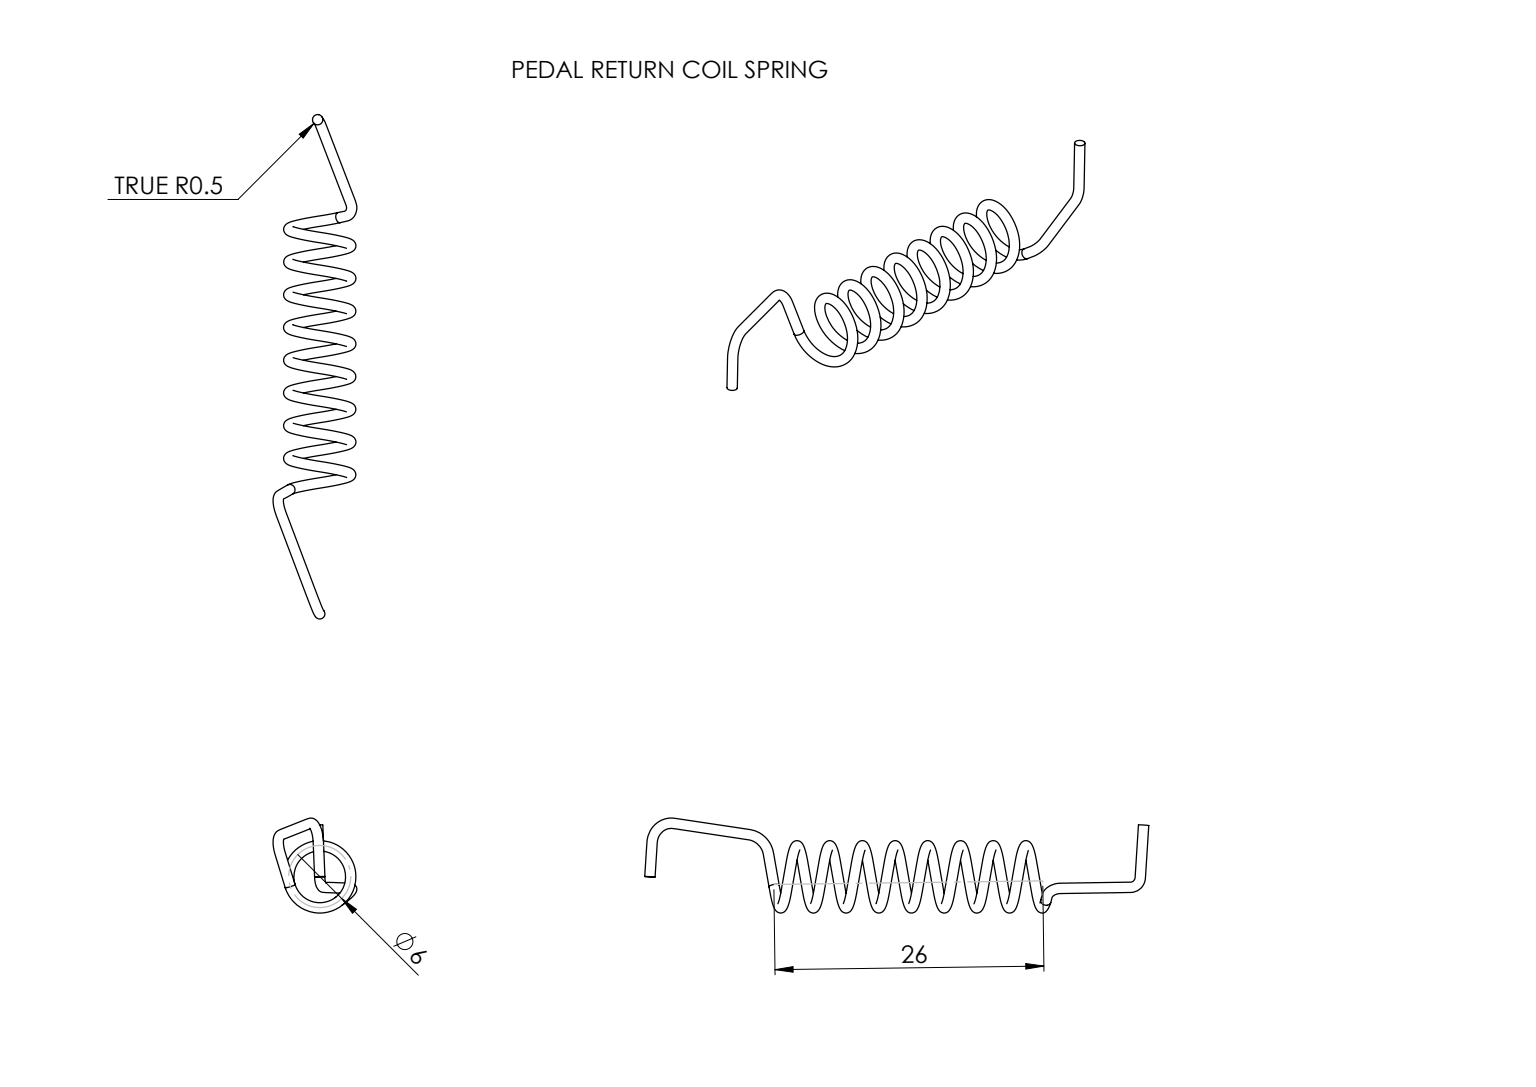
ISO-10303-21;
HEADER;
FILE_DESCRIPTION (('STEP AP214'),
    '1' );
FILE_NAME ('Pedal Return Coil Spring.step',
    '2026-09-30T16:28:02',
    ( '' ),
    ( '' ),
    'SwSTEP 2.0',
    'SolidWorks 2026',
    '' );
FILE_SCHEMA (( 'AUTOMOTIVE_DESIGN' ));
ENDSEC;

DATA;
#3=CARTESIAN_POINT ( 'NONE',  ( 10.46436961932593945, 16.48727764291732711, -17.33901581970886241 ) ) ;
#5=CARTESIAN_POINT ( 'NONE',  ( 33.35202879388211983, -12.33251541790028760, -19.68467382345759376 ) ) ;
#7=CARTESIAN_POINT ( 'NONE',  ( 11.86544027865023843, 7.919735734555668039, -16.84125344233394372 ) ) ;
#10=CARTESIAN_POINT ( 'NONE',  ( 20.51249478307574847, 1.942573248051725709, -13.31196225760961838 ) ) ;
#11=CARTESIAN_POINT ( 'NONE',  ( 11.27738072919014911, 16.67146171448561276, -16.78403338633166442 ) ) ;
#12=CARTESIAN_POINT ( 'NONE',  ( 35.03938282813840743, -19.89690018161999419, -20.20402626681843117 ) ) ;
#15=CARTESIAN_POINT ( 'NONE',  ( 9.776119957569173735, 17.05082265352876547, -16.72288386497739765 ) ) ;
#18=CARTESIAN_POINT ( 'NONE',  ( 9.641351338355821810, 17.66888872024471624, -17.91303689663363130 ) ) ;
#25=CARTESIAN_POINT ( 'NONE',  ( 10.43477690885096720, 16.62299358534909288, -17.37687480348504820 ) ) ;
#28=CARTESIAN_POINT ( 'NONE',  ( 36.54859390953724585, -22.18451583373416014, -17.64281456791166036 ) ) ;
#29=CARTESIAN_POINT ( 'NONE',  ( 24.62590367393082502, -9.567571807129121808, -15.85044010117769098 ) ) ;
#37=CARTESIAN_POINT ( 'NONE',  ( 19.85258860919307367, 6.732389232436280402, -16.96582824858274208 ) ) ;
#39=CARTESIAN_POINT ( 'NONE',  ( 29.40876261992080032, -8.787110225502646088, -16.42709622331022956 ) ) ;
#44=CARTESIAN_POINT ( 'NONE',  ( 10.00000000000007816, 17.32050807568872486, -23.00000000000000711 ) ) ;
#48=CARTESIAN_POINT ( 'NONE',  ( 10.33812866905494587, 18.38613571942487113, -17.90056368370468931 ) ) ;
#54=CARTESIAN_POINT ( 'NONE',  ( 9.917712295358372288, 16.40146214360271770, -16.50402730409559027 ) ) ;
#56=CARTESIAN_POINT ( 'NONE',  ( 28.55476651072185845, -11.97999099613336504, -13.94805024529803994 ) ) ;
#58=CARTESIAN_POINT ( 'NONE',  ( 25.71553203045151292, -8.406338935355361031, -18.42709291467145150 ) ) ;
#61=CARTESIAN_POINT ( 'NONE',  ( 11.05541548581436118, 17.68942261459453036, -17.91440211708152574 ) ) ;
#63=CARTESIAN_POINT ( 'NONE',  ( 32.97927115036063839, -11.75136040154610662, -17.31233706439427067 ) ) ;
#64=CARTESIAN_POINT ( 'NONE',  ( 14.34656430690936624, 9.113120221615268690, -15.03016663717492563 ) ) ;
#68=CARTESIAN_POINT ( 'NONE',  ( 23.37849240255853189, -5.075553540114302820, -18.86401745356084447 ) ) ;
#73=CARTESIAN_POINT ( 'NONE',  ( 16.00562779705659011, 2.776126820729137190, -17.20623408552720690 ) ) ;
#74=CARTESIAN_POINT ( 'NONE',  ( 16.42253358145367415, 4.166353156564198024, -16.06924993952044289 ) ) ;
#83=CARTESIAN_POINT ( 'NONE',  ( 9.641350810849047548, 17.66889113945805789, -17.91928203681695564 ) ) ;
#84=CARTESIAN_POINT ( 'NONE',  ( 20.82548126942529976, -5.669333895406754031, -14.77195412306030420 ) ) ;
#85=CARTESIAN_POINT ( 'NONE',  ( 23.74924978780510898, -3.048960050427876656, -13.27477993493952191 ) ) ;
#87=CARTESIAN_POINT ( 'NONE',  ( 36.54859390953724585, -23.18451583373416014, -18.06010107863414405 ) ) ;
#95=CARTESIAN_POINT ( 'NONE',  ( 10.33811987107833552, 18.38617606806709048, -17.90816805339326834 ) ) ;
#100=CARTESIAN_POINT ( 'NONE',  ( 14.18486973814142793, 6.324582201221724098, -17.68508340245422872 ) ) ;
#104=CARTESIAN_POINT ( 'NONE',  ( 25.08912532741139501, -12.86307741315042108, -14.91192194027685147 ) ) ;
#107=CARTESIAN_POINT ( 'NONE',  ( 34.90271572771163733, -20.28292729397994876, -21.20502438346732887 ) ) ;
#108=CARTESIAN_POINT ( 'NONE',  ( 24.18628427323349328, -0.8779346998738073449, -17.06787597161793357 ) ) ;
#109=CARTESIAN_POINT ( 'NONE',  ( 18.93384218461971358, 6.651393094135895190, -15.21227712214292538 ) ) ;
#111=CARTESIAN_POINT ( 'NONE',  ( 28.58746438791548528, -7.443717211345676432, -18.79719194573140584 ) ) ;
#120=CARTESIAN_POINT ( 'NONE',  ( 33.16581763841239194, -10.35476010881584052, -17.60936685258081624 ) ) ;
#121=CARTESIAN_POINT ( 'NONE',  ( 9.641890818133653340, 17.66641459721583374, -17.82828029666912073 ) ) ;
#126=CARTESIAN_POINT ( 'NONE',  ( 10.46960557229346733, 16.46326489517938541, -17.33590790293451178 ) ) ;
#139=CARTESIAN_POINT ( 'NONE',  ( 11.09431937732777129, 9.685491096586417825, -17.29518830297554643 ) ) ;
#140=CARTESIAN_POINT ( 'NONE',  ( 25.86320101420157158, -8.291784280105535032, -12.84902276017926859 ) ) ;
#141=CARTESIAN_POINT ( 'NONE',  ( 19.89307947303188229, -2.966738011908462092, -16.73278295482091949 ) ) ;
#143=CARTESIAN_POINT ( 'NONE',  ( 18.39996379557756256, 0.6904185378075045065, -15.43317298867526866 ) ) ;
#147=CARTESIAN_POINT ( 'NONE',  ( 27.44219139316946965, -6.774709612358828181, -18.29578255718776703 ) ) ;
#156=CARTESIAN_POINT ( 'NONE',  ( 10.35864918915110877, 16.97212501191939538, -17.92279151347709032 ) ) ;
#157=CARTESIAN_POINT ( 'NONE',  ( 35.24964364652129234, -20.84149066036063047, -20.16262864730545346 ) ) ;
#158=CARTESIAN_POINT ( 'NONE',  ( 31.39893620166130717, -10.86152586746012183, -14.84747879817187943 ) ) ;
#160=CARTESIAN_POINT ( 'NONE',  ( 8.944584812045984989, 16.95159217075808655, -17.91472939532503261 ) ) ;
#163=CARTESIAN_POINT ( 'NONE',  ( 19.38992137333195842, 2.881095379261479739, -20.30776781288435373 ) ) ;
#164=CARTESIAN_POINT ( 'NONE',  ( 11.27814055543051630, 16.66797705449195988, -16.78371917145281955 ) ) ;
#169=CARTESIAN_POINT ( 'NONE',  ( 9.916551108984865692, 16.40678749232849398, -16.50450761325770443 ) ) ;
#171=CARTESIAN_POINT ( 'NONE',  ( 9.843778300897430000, 16.74053286659246709, -16.57516421589427225 ) ) ;
#179=CARTESIAN_POINT ( 'NONE',  ( 10.35887147716723611, 16.97110557074245563, -17.87975733919941845 ) ) ;
#181=CARTESIAN_POINT ( 'NONE',  ( 36.04209255463945993, -19.90907354740926394, -20.43687144983462289 ) ) ;
#182=CARTESIAN_POINT ( 'NONE',  ( 21.18945582756405344, -5.194394521544061227, -16.21196392551894405 ) ) ;
#183=CARTESIAN_POINT ( 'NONE',  ( 27.21278356834291756, -7.014839303453253905, -18.45691071023835761 ) ) ;
#186=CIRCLE ( 'NONE', #15750, 0.4999999999999998335 ) ;
#189=CARTESIAN_POINT ( 'NONE',  ( 19.09420370221858931, 5.586061004495046056, -18.95245686415860220 ) ) ;
#190=CARTESIAN_POINT ( 'NONE',  ( 26.02011856185544048, -9.832954462109395166, -14.66174570188732140 ) ) ;
#200=CARTESIAN_POINT ( 'NONE',  ( 10.73095126193553028, 16.58460123524055874, -15.94999808000346242 ) ) ;
#204=CARTESIAN_POINT ( 'NONE',  ( 9.916551108984865692, 16.40678749232849398, -16.50450761325770443 ) ) ;
#206=CARTESIAN_POINT ( 'NONE',  ( 18.72855672543857608, 2.184447897796080174, -13.82944682127929426 ) ) ;
#210=CARTESIAN_POINT ( 'NONE',  ( 25.79824969357368047, -12.24460132778619226, -15.92960863319586906 ) ) ;
#213=CARTESIAN_POINT ( 'NONE',  ( 11.05541700792677062, 17.68941563399299710, -17.91138715956864047 ) ) ;
#215=CARTESIAN_POINT ( 'NONE',  ( 33.76744293605320024, -13.18274801178271005, -18.77722780292321758 ) ) ;
#219=CARTESIAN_POINT ( 'NONE',  ( 23.38597214775318278, -9.778565425610747042, -17.35394146810280347 ) ) ;
#223=CARTESIAN_POINT ( 'NONE',  ( 21.13650371987585075, 4.769999862021419901, -15.38713752973847448 ) ) ;
#224=CARTESIAN_POINT ( 'NONE',  ( 17.80416238081608071, 8.561068417093343541, -18.87148919878627140 ) ) ;
#238=CARTESIAN_POINT ( 'NONE',  ( 9.921764701973689426, 16.38287729030320250, -16.50235149140834778 ) ) ;
#239=CARTESIAN_POINT ( 'NONE',  ( 23.58034929565730309, -2.629172400889816075, -20.70693660786654888 ) ) ;
#240=CARTESIAN_POINT ( 'NONE',  ( 19.50876870223950377, -1.661710298099399630, -15.95382585723518432 ) ) ;
#241=CARTESIAN_POINT ( 'NONE',  ( 32.24963562184495203, -10.43994945000269148, -19.19593526939238970 ) ) ;
#242=ORIENTED_EDGE ( 'NONE', *, *, #15818, .F. ) ;
#248=CARTESIAN_POINT ( 'NONE',  ( 14.39533340154967433, 6.572929804808670617, -18.54476805420031837 ) ) ;
#251=CARTESIAN_POINT ( 'NONE',  ( 10.68867725192709273, 16.77847523382220984, -15.97313786900300059 ) ) ;
#255=CARTESIAN_POINT ( 'NONE',  ( 19.20291185354690811, 8.143073066566493878, -16.32372945079811188 ) ) ;
#256=CARTESIAN_POINT ( 'NONE',  ( 16.48605814428184857, 11.34583003460130435, -14.75612992736757256 ) ) ;
#258=CARTESIAN_POINT ( 'NONE',  ( 35.54859390953724585, -23.18451583373416014, -16.11276402859391510 ) ) ;
#259=CARTESIAN_POINT ( 'NONE',  ( 20.30498772102510685, -2.023023832184298154, -16.94527736422809028 ) ) ;
#260=CARTESIAN_POINT ( 'NONE',  ( 18.10666546173949953, 1.615696121519054618, -15.79491705146812563 ) ) ;
#262=CARTESIAN_POINT ( 'NONE',  ( 25.27233071153842303, -10.58027458246514207, -17.53878701932553952 ) ) ;
#272=CARTESIAN_POINT ( 'NONE',  ( 36.32827445255054499, -20.19473721995742821, -19.46526261299151983 ) ) ;
#273=CARTESIAN_POINT ( 'NONE',  ( 15.87304960759194650, 9.003283391651189405, -12.44179493704351280 ) ) ;
#277=CARTESIAN_POINT ( 'NONE',  ( 10.55304143273637330, 16.08061740358965253, -17.30129946959702281 ) ) ;
#289=CARTESIAN_POINT ( 'NONE',  ( 9.667856465286563505, 16.22743184293591057, -17.88508098240584587 ) ) ;
#290=CARTESIAN_POINT ( 'NONE',  ( 26.82298874931487020, -4.830090842487210878, -14.67398021261910301 ) ) ;
#291=CARTESIAN_POINT ( 'NONE',  ( 23.41849298471255381, -3.203224238779429633, -13.27670244232306018 ) ) ;
#296=CARTESIAN_POINT ( 'NONE',  ( 25.26806593431409453, -8.821542497490490575, -18.05414547114721557 ) ) ;
#309=CARTESIAN_POINT ( 'NONE',  ( 10.47103768343372288, 16.45669705093847313, -17.33522727542475295 ) ) ;
#313=CARTESIAN_POINT ( 'NONE',  ( 13.40647825129878612, 7.637826363492710158, -15.68645975549014082 ) ) ;
#316=CARTESIAN_POINT ( 'NONE',  ( 23.66272512268759343, 2.894330346666426745, -16.12005855839824520 ) ) ;
#317=CARTESIAN_POINT ( 'NONE',  ( 11.27662090294977837, 16.67494637447927275, -16.78434760121053060 ) ) ;
#321=CARTESIAN_POINT ( 'NONE',  ( 9.641350835837977584, 17.66889102485563612, -17.91507476468484938 ) ) ;
#324=CARTESIAN_POINT ( 'NONE',  ( 9.916953853453376766, 16.40494045485788632, -16.50434094533541085 ) ) ;
#330=CARTESIAN_POINT ( 'NONE',  ( 10.47325967749744180, 16.44650670292386607, -17.33429203187744250 ) ) ;
#333=CARTESIAN_POINT ( 'NONE',  ( 32.72409873491027099, -9.637868425582460929, -18.36260606011342844 ) ) ;
#334=CARTESIAN_POINT ( 'NONE',  ( 29.22485947447185595, -8.910266539455653501, -18.36689805200119707 ) ) ;
#335=CARTESIAN_POINT ( 'NONE',  ( 25.23810427664335165, -6.496417100615061280, -13.69959235629456629 ) ) ;
#338=CARTESIAN_POINT ( 'NONE',  ( 34.33515578781254618, -12.24072284059296933, -19.92088757525016973 ) ) ;
#340=CARTESIAN_POINT ( 'NONE',  ( 15.71409287621466788, 5.292507472020409942, -15.15310296786427635 ) ) ;
#341=CARTESIAN_POINT ( 'NONE',  ( 26.65048721414892086, -11.67344998524500355, -15.88597958324129777 ) ) ;
#353=CARTESIAN_POINT ( 'NONE',  ( 10.71275814632708823, 16.66803718250374899, -15.95787532639072914 ) ) ;
#358=CARTESIAN_POINT ( 'NONE',  ( 9.914377700407460026, 16.41675502110963336, -16.50544604630902867 ) ) ;
#359=CARTESIAN_POINT ( 'NONE',  ( 9.667469407758799704, 16.22920693809672343, -17.88529630510330293 ) ) ;
#360=CARTESIAN_POINT ( 'NONE',  ( 17.70496941102466693, 2.403166580496164606, -19.15355645582771871 ) ) ;
#363=CARTESIAN_POINT ( 'NONE',  ( 29.90031526554274777, -7.862644070287768905, -16.42500436498598049 ) ) ;
#365=CARTESIAN_POINT ( 'NONE',  ( 11.27712745377669101, 16.67262326781682802, -16.78413812462462573 ) ) ;
#367=CARTESIAN_POINT ( 'NONE',  ( 35.54859390953724585, -21.18451583373416014, -16.94733705004010105 ) ) ;
#370=CARTESIAN_POINT ( 'NONE',  ( 9.112490548836888138, 16.18155505883174783, -17.05474119751274031 ) ) ;
#371=CARTESIAN_POINT ( 'NONE',  ( 28.50845745928996067, -4.315366227951761502, -16.60164569054668604 ) ) ;
#375=CARTESIAN_POINT ( 'NONE',  ( 18.32179412900206827, 3.681508181950223335, -14.15692665485406643 ) ) ;
#377=CARTESIAN_POINT ( 'NONE',  ( 16.45434084995319424, 8.990804261541395448, -14.78801614696073408 ) ) ;
#387=CARTESIAN_POINT ( 'NONE',  ( 9.926830210242822972, 16.35964622367879784, -16.50025672554925293 ) ) ;
#388=CARTESIAN_POINT ( 'NONE',  ( 29.32553208039167458, -8.962988822949116141, -16.84503999589972523 ) ) ;
#389=CARTESIAN_POINT ( 'NONE',  ( 19.55718041265476970, -1.390565517676688900, -17.79492730709450754 ) ) ;
#390=CARTESIAN_POINT ( 'NONE',  ( 36.54859390953724585, -23.18451583373416014, -16.94733705004010105 ) ) ;
#396=CARTESIAN_POINT ( 'NONE',  ( 14.03850921439652311, 8.975161913830900673, -15.18271992443145635 ) ) ;
#399=CARTESIAN_POINT ( 'NONE',  ( 10.35722669462089840, 18.29854973974792998, -17.31575102165233915 ) ) ;
#403=CARTESIAN_POINT ( 'NONE',  ( 15.14574614762244487, 6.587483969391940697, -15.14885142785537830 ) ) ;
#405=CARTESIAN_POINT ( 'NONE',  ( 12.96291568738609890, 5.695260009123724210, -16.43886026595064109 ) ) ;
#407=CARTESIAN_POINT ( 'NONE',  ( 32.30218501430429967, -10.99871056796995816, -17.40035725849610060 ) ) ;
#410=CARTESIAN_POINT ( 'NONE',  ( 23.12480016457037379, 1.528454477237789488, -15.53356264363713102 ) ) ;
#412=CARTESIAN_POINT ( 'NONE',  ( 19.55510877418759819, -0.09764134006120470111, -19.21341144728512518 ) ) ;
#414=CARTESIAN_POINT ( 'NONE',  ( 27.32534031592636836, -8.675155620653059785, -19.25315075663615971 ) ) ;
#422=CARTESIAN_POINT ( 'NONE',  ( 35.57309713841538468, -16.80212557611773505, -19.25277297559858525 ) ) ;
#423=CARTESIAN_POINT ( 'NONE',  ( 9.641566850259106758, 17.66790035518494051, -17.86107206016944460 ) ) ;
#427=CARTESIAN_POINT ( 'NONE',  ( 12.02823749386838514, 9.315180647891255106, -16.69125397286443047 ) ) ;
#437=CARTESIAN_POINT ( 'NONE',  ( 9.667845848563926481, 16.22748053257927126, -17.88508528815513543 ) ) ;
#441=CARTESIAN_POINT ( 'NONE',  ( 25.04433344647707571, -4.420048373160954114, -18.22226412361657921 ) ) ;
#443=CARTESIAN_POINT ( 'NONE',  ( 21.55249387529322647, -4.041031698679099726, -14.19001464829599435 ) ) ;
#447=DIRECTION ( 'NONE',  ( -0.7172983783020613346, 0.6967661275386690667, -3.330669073875468142E-16 ) ) ;
#448=CARTESIAN_POINT ( 'NONE',  ( 26.72181814967143509, -3.137724904577397389, -15.69709663067708050 ) ) ;
#456=CARTESIAN_POINT ( 'NONE',  ( 12.02305193244137449, 9.338961869187645704, -16.69339841729684437 ) ) ;
#458=CARTESIAN_POINT ( 'NONE',  ( 34.96805304670973413, -19.57645325810014114, -20.18246498508359466 ) ) ;
#460=CARTESIAN_POINT ( 'NONE',  ( 13.81482270056995532, 7.818281081198240834, -15.36100202165747675 ) ) ;
#463=CARTESIAN_POINT ( 'NONE',  ( 21.66440995182641416, 5.535554982823286174, -17.57621636221614025 ) ) ;
#464=CARTESIAN_POINT ( 'NONE',  ( 12.84801357566967717, 9.517348710814296453, -16.13078356789775469 ) ) ;
#469=CARTESIAN_POINT ( 'NONE',  ( 11.40798482813988635, 9.566882342703072695, -15.88774718835883348 ) ) ;
#471=CARTESIAN_POINT ( 'NONE',  ( 10.24089172292967298, 14.91932009296530559, -16.37038124228770997 ) ) ;
#476=CARTESIAN_POINT ( 'NONE',  ( 10.40163623209820365, 16.77498095339038287, -17.46874319472340176 ) ) ;
#479=CARTESIAN_POINT ( 'NONE',  ( 32.45862320860160821, -9.597537451891041016, -17.61229109800368064 ) ) ;
#480=CARTESIAN_POINT ( 'NONE',  ( 29.62588713853392264, -10.65184931322849060, -12.76488833982454629 ) ) ;
#481=CARTESIAN_POINT ( 'NONE',  ( 29.46565128511723586, -7.689737916804423534, -14.82739468409561567 ) ) ;
#492=CARTESIAN_POINT ( 'NONE',  ( 28.92040988821396752, -12.03996551347764132, -12.87516188627701474 ) ) ;
#493=CARTESIAN_POINT ( 'NONE',  ( 26.45169718342334164, -9.008644514675534509, -18.11399877363951205 ) ) ;
#503=CARTESIAN_POINT ( 'NONE',  ( 10.33813570737955700, 18.38610344077106973, -17.89676158639688452 ) ) ;
#507=CARTESIAN_POINT ( 'NONE',  ( 9.917965570771830386, 16.40030059027150600, -16.50392256580263606 ) ) ;
#508=CARTESIAN_POINT ( 'NONE',  ( 20.43163981785493988, 0.2187255735321424754, -20.49791845872360341 ) ) ;
#514=CARTESIAN_POINT ( 'NONE',  ( 11.27864710625743427, 16.66565394782951515, -16.78350969486689692 ) ) ;
#516=EDGE_LOOP ( 'NONE', ( #242, #27504, #8040, #18443, #3018 ) ) ;
#517=CARTESIAN_POINT ( 'NONE',  ( 35.24753590068310416, -19.83202167481471889, -19.22462439892593977 ) ) ;
#519=CARTESIAN_POINT ( 'NONE',  ( 17.72480397827495224, 1.356124466512965476, -19.40231245121514903 ) ) ;
#522=CARTESIAN_POINT ( 'NONE',  ( 9.112135424753279977, 16.18318370314694832, -17.05489040841110437 ) ) ;
#523=CARTESIAN_POINT ( 'NONE',  ( 24.27832910178602788, -5.559203070376852018, -13.12236226054620047 ) ) ;
#530=CARTESIAN_POINT ( 'NONE',  ( 21.58357356133149807, 4.347441036859617469, -17.91576365920758107 ) ) ;
#531=CARTESIAN_POINT ( 'NONE',  ( 18.42634509371275797, 7.189141296957872740, -15.94500943014882210 ) ) ;
#545=CARTESIAN_POINT ( 'NONE',  ( 9.916411867603999397, 16.40742607105030260, -16.50456570466356965 ) ) ;
#546=CARTESIAN_POINT ( 'NONE',  ( 28.54819463643023880, -8.737303380947411213, -14.37855314081258307 ) ) ;
#547=CARTESIAN_POINT ( 'NONE',  ( 20.97044927184332508, -4.289323992320570156, -15.06659861376252429 ) ) ;
#549=CARTESIAN_POINT ( 'NONE',  ( 32.45272648307624053, -11.02157468472264412, -17.82583700188536824 ) ) ;
#555=CARTESIAN_POINT ( 'NONE',  ( 16.09764958744793262, 8.143416238145906760, -19.84970969296679044 ) ) ;
#558=CARTESIAN_POINT ( 'NONE',  ( 10.33819201225523621, 18.38584521943398187, -17.87775236254758227 ) ) ;
#561=CARTESIAN_POINT ( 'NONE',  ( 17.32695330507268494, 5.471673316493076200, -20.08600194542987794 ) ) ;
#562=CARTESIAN_POINT ( 'NONE',  ( 16.38450301900381945, 9.168174629645104545, -21.04437084800770918 ) ) ;
#564=CARTESIAN_POINT ( 'NONE',  ( 32.45272648307624053, -11.02157468472264412, -17.82583700188536824 ) ) ;
#566=CARTESIAN_POINT ( 'NONE',  ( 23.60892706051935619, -2.861763136178346212, -14.25286661070829908 ) ) ;
#568=CARTESIAN_POINT ( 'NONE',  ( 22.48601049859325585, 2.925819830077934558, -17.76611561182923893 ) ) ;
#569=CARTESIAN_POINT ( 'NONE',  ( 28.63790973356518776, -5.888324979419876648, -13.82040474618100312 ) ) ;
#577=CARTESIAN_POINT ( 'NONE',  ( 32.71419323209526908, -10.28616775856061416, -16.33292762241428520 ) ) ;
#579=CARTESIAN_POINT ( 'NONE',  ( 9.641354186875979337, 17.66887565656821124, -17.90893343548146177 ) ) ;
#583=CARTESIAN_POINT ( 'NONE',  ( 13.10707286029108865, 8.563798077496334926, -15.92507172258792281 ) ) ;
#593=CARTESIAN_POINT ( 'NONE',  ( 11.22273001195053155, 9.096583557657577757, -17.24208598844832352 ) ) ;
#594=CARTESIAN_POINT ( 'NONE',  ( 27.63487812444411418, -5.020849242181972372, -17.14317672846274831 ) ) ;
#595=CARTESIAN_POINT ( 'NONE',  ( 26.02348467347448491, -3.622150272347476108, -19.21400332953221124 ) ) ;
#602=CARTESIAN_POINT ( 'NONE',  ( 35.54859390953723874, -22.18451583373416014, -15.00000000000000000 ) ) ;
#605=CARTESIAN_POINT ( 'NONE',  ( 12.02786405831828986, 9.316892843345049968, -16.69140843421181231 ) ) ;
#609=CARTESIAN_POINT ( 'NONE',  ( 32.54305136433941215, -11.03529315477374517, -18.08112484791816499 ) ) ;
#611=CARTESIAN_POINT ( 'NONE',  ( 8.944584663113916534, 16.95159285377954461, -17.91618150236991269 ) ) ;
#616=CARTESIAN_POINT ( 'NONE',  ( 23.86551563699305234, 2.542095107771292106, -17.79649620197707094 ) ) ;
#617=CARTESIAN_POINT ( 'NONE',  ( 12.83210864641033844, 9.541281304504437344, -16.14109870176968897 ) ) ;
#620=CARTESIAN_POINT ( 'NONE',  ( 11.47029057985033340, 9.281140223223081520, -15.86198156829250117 ) ) ;
#622=CARTESIAN_POINT ( 'NONE',  ( 9.745779815811758340, 17.18996641109745482, -16.82979807527155458 ) ) ;
#627=CARTESIAN_POINT ( 'NONE',  ( 12.00785540763395254, 9.408655069060824161, -16.69968271487400813 ) ) ;
#629=CARTESIAN_POINT ( 'NONE',  ( 36.54859390954303677, -22.18451583373416014, -15.55638201429745848 ) ) ;
#630=CARTESIAN_POINT ( 'NONE',  ( 30.24922550192677306, -10.40856591028444278, -13.02298783260255988 ) ) ;
#631=CARTESIAN_POINT ( 'NONE',  ( 27.11191462667604313, -11.78482644060662743, -13.28705938033944989 ) ) ;
#636=CARTESIAN_POINT ( 'NONE',  ( 17.00902653454025071, 3.367308883600929281, -16.20218648120260951 ) ) ;
#637=CARTESIAN_POINT ( 'NONE',  ( 26.84622329165386745, -11.42663724297536554, -16.80226328336580366 ) ) ;
#649=CARTESIAN_POINT ( 'NONE',  ( 12.26681336913932974, 9.540941834721429871, -15.31486507153535648 ) ) ;
#654=CARTESIAN_POINT ( 'NONE',  ( 12.23783994716398560, 8.515526397163364791, -15.33449341356891615 ) ) ;
#656=CARTESIAN_POINT ( 'NONE',  ( 17.93652952100233833, 4.843921488302829204, -14.86957952233187896 ) ) ;
#661=CARTESIAN_POINT ( 'NONE',  ( 12.83625023806442655, 9.529724225483313660, -16.13881881377442795 ) ) ;
#663=CARTESIAN_POINT ( 'NONE',  ( 33.57416420788476330, -12.34692739235205217, -18.69991813917680190 ) ) ;
#664=CARTESIAN_POINT ( 'NONE',  ( 14.33367420948735393, 6.252843122977492563, -16.41390433006782956 ) ) ;
#666=CARTESIAN_POINT ( 'NONE',  ( 22.02790516022008660, -6.446180030103099590, -16.19395709203531197 ) ) ;
#670=CARTESIAN_POINT ( 'NONE',  ( 21.81760893248375766, -3.923850722439390815, -13.93537712798182682 ) ) ;
#671=CARTESIAN_POINT ( 'NONE',  ( 15.53255613197921647, 5.987779765840379298, -16.04456276566740058 ) ) ;
#684=CARTESIAN_POINT ( 'NONE',  ( 11.47748818427356987, 9.248962635895034978, -15.85894168489154765 ) ) ;
#686=CARTESIAN_POINT ( 'NONE',  ( 29.25528888857379783, -9.059906918047152757, -17.02304095575280130 ) ) ;
#687=CARTESIAN_POINT ( 'NONE',  ( 21.37428249720081297, 2.009508332918806151, -14.44682725892062614 ) ) ;
#688=CARTESIAN_POINT ( 'NONE',  ( 35.54750751241274287, -23.17963522693337453, -18.53372063443203999 ) ) ;
#695=CARTESIAN_POINT ( 'NONE',  ( 20.52488529563827058, 3.974637744936419637, -19.97762432673833288 ) ) ;
#698=CARTESIAN_POINT ( 'NONE',  ( 10.72031594518761466, 16.63337615353409760, -15.95439753950889106 ) ) ;
#702=CARTESIAN_POINT ( 'NONE',  ( 22.29983652437130814, 0.6627547066652448304, -20.09853802436992964 ) ) ;
#704=CARTESIAN_POINT ( 'NONE',  ( 28.86700826148938859, -9.048814421258168039, -19.66053155205330683 ) ) ;
#706=CARTESIAN_POINT ( 'NONE',  ( 35.32886446602115171, -21.19738783794349857, -20.03221113960638178 ) ) ;
#707=CARTESIAN_POINT ( 'NONE',  ( 22.40033610297568956, 1.362009800809227178, -14.54093962742820700 ) ) ;
#708=CARTESIAN_POINT ( 'NONE',  ( 19.97593658988278165, 3.663230212540239616, -18.70116431613266883 ) ) ;
#715=CARTESIAN_POINT ( 'NONE',  ( 34.70514358766799745, -13.90287004036446739, -20.03273298744158737 ) ) ;
#716=CARTESIAN_POINT ( 'NONE',  ( 12.81042928357508970, 7.649856678006609734, -14.88275739421262855 ) ) ;
#719=CARTESIAN_POINT ( 'NONE',  ( 13.12048998592846871, 8.569482736746577345, -15.91439669260688561 ) ) ;
#728=CARTESIAN_POINT ( 'NONE',  ( 11.21893088074867073, 9.114006857625895464, -17.24365706284262600 ) ) ;
#729=CARTESIAN_POINT ( 'NONE',  ( 24.63339645208565543, -5.721020077635508905, -14.05062826560360278 ) ) ;
#730=CARTESIAN_POINT ( 'NONE',  ( 20.05514754915220266, -1.452567280579552866, -14.87399747198034738 ) ) ;
#743=CARTESIAN_POINT ( 'NONE',  ( 10.79618582965528439, 14.96552620561766567, -17.20075070836251996 ) ) ;
#745=CARTESIAN_POINT ( 'NONE',  ( 33.55945865873172096, -12.30028340163019607, -18.68418013052470883 ) ) ;
#747=CARTESIAN_POINT ( 'NONE',  ( 13.39286676965551059, 7.631811206235384226, -15.69730834661896424 ) ) ;
#750=CARTESIAN_POINT ( 'NONE',  ( 21.69765170278760280, -5.035756590920279940, -14.89200278627170881 ) ) ;
#751=CARTESIAN_POINT ( 'NONE',  ( 12.86751881037522871, 9.515731068868671372, -16.11601834121851340 ) ) ;
#757=CARTESIAN_POINT ( 'NONE',  ( 11.47155695691762212, 9.275332456566969697, -15.86145787682774078 ) ) ;
#759=CARTESIAN_POINT ( 'NONE',  ( 9.870716668364401869, 16.61699007954640805, -16.53972800451630931 ) ) ;
#765=CARTESIAN_POINT ( 'NONE',  ( 12.02932678857878734, 9.310239991255825132, -16.69079931733866218 ) ) ;
#768=CARTESIAN_POINT ( 'NONE',  ( 36.54859682288668665, -23.18452892187019643, -18.24988411864624993 ) ) ;
#769=CARTESIAN_POINT ( 'NONE',  ( 24.62590367393082502, -9.567571807129121808, -15.85044010117769098 ) ) ;
#770=CARTESIAN_POINT ( 'NONE',  ( 31.22280883588763700, -10.09333740185288875, -13.86128061636125786 ) ) ;
#773=CARTESIAN_POINT ( 'NONE',  ( 34.31936231504242585, -12.17391896401218609, -19.91370162440023250 ) ) ;
#777=CARTESIAN_POINT ( 'NONE',  ( 18.73405575602592776, 1.888441813480535414, -14.99786396448725156 ) ) ;
#780=CARTESIAN_POINT ( 'NONE',  ( 14.79111372287554715, 6.954724682967856175, -19.27298399620107361 ) ) ;
#792=CARTESIAN_POINT ( 'NONE',  ( 12.27691635572497830, 9.494607244959519576, -15.31068720787289728 ) ) ;
#798=CARTESIAN_POINT ( 'NONE',  ( 12.50226005284522657, 8.571700941790735939, -15.12837371066060221 ) ) ;
#801=CARTESIAN_POINT ( 'NONE',  ( 19.55603740332541918, 4.113176889600292263, -19.54140316641015573 ) ) ;
#807=CARTESIAN_POINT ( 'NONE',  ( 12.57288446902313872, 10.73011642529405307, -16.24829701787703939 ) ) ;
#809=CARTESIAN_POINT ( 'NONE',  ( 34.19542162461613799, -15.10542955289956346, -18.90659549333309286 ) ) ;
#810=CARTESIAN_POINT ( 'NONE',  ( 15.14574614762244487, 6.587483969391940697, -15.14885142785537830 ) ) ;
#812=CARTESIAN_POINT ( 'NONE',  ( 16.96387855261641775, 8.441957738943033362, -20.67322241009641814 ) ) ;
#816=CARTESIAN_POINT ( 'NONE',  ( 21.34960977245966873, -3.524359730468174412, -18.69795900347392248 ) ) ;
#818=CARTESIAN_POINT ( 'NONE',  ( 17.70496941102466693, 2.403166580496164606, -19.15355645582771871 ) ) ;
#828=DIRECTION ( 'NONE',  ( 1.665334536937734318E-16, -2.498001805406601723E-16, -1.000000000000000000 ) ) ;
#833=CARTESIAN_POINT ( 'NONE',  ( 11.55687758731922798, 9.016417257711555777, -15.81607864292198329 ) ) ;
#834=CARTESIAN_POINT ( 'NONE',  ( 26.64397501440380012, -9.555891369342745634, -14.23407566704858951 ) ) ;
#835=CARTESIAN_POINT ( 'NONE',  ( 24.30592326428028827, -5.273034306582022879, -19.67074064463221106 ) ) ;
#836=CARTESIAN_POINT ( 'NONE',  ( 33.41663030065195272, -12.60673267154789201, -19.71350710734569134 ) ) ;
#845=CARTESIAN_POINT ( 'NONE',  ( 18.21616227284554057, 4.699354889203569918, -13.86658597208997179 ) ) ;
#848=CARTESIAN_POINT ( 'NONE',  ( 12.27693042220145969, 9.494543488390625896, -15.31068133337694803 ) ) ;
#853=CARTESIAN_POINT ( 'NONE',  ( 18.34549112274340033, 0.9605221043122941227, -13.99314825615798341 ) ) ;
#854=CARTESIAN_POINT ( 'NONE',  ( 18.76228799092704236, 0.4007544294800896578, -19.29634928253052806 ) ) ;
#856=CARTESIAN_POINT ( 'NONE',  ( 33.54145741815126058, -13.16751478770765793, -19.75123935038191192 ) ) ;
#857=( NAMED_UNIT ( * ) PLANE_ANGLE_UNIT ( ) SI_UNIT ( $, .RADIAN. ) );
#858=CARTESIAN_POINT ( 'NONE',  ( 25.72734949418555317, -2.696321649843969936, -17.76569039084671786 ) ) ;
#859=CARTESIAN_POINT ( 'NONE',  ( 17.76107737582129431, 3.703408080355245158, -15.36634439411934316 ) ) ;
#874=CARTESIAN_POINT ( 'NONE',  ( 33.36027191889437660, -10.38700102556154903, -18.15738432823107473 ) ) ;
#875=CIRCLE ( 'NONE', #26731, 0.4999999999999998335 ) ;
#876=CARTESIAN_POINT ( 'NONE',  ( 9.905109554012803130, 16.45925992188944420, -16.51025697316969953 ) ) ;
#879=CARTESIAN_POINT ( 'NONE',  ( 12.02558468657594659, 9.327346335875439820, -16.69235103436730938 ) ) ;
#889=CARTESIAN_POINT ( 'NONE',  ( 13.34629304935920757, 7.611730149031187054, -15.73439023580873730 ) ) ;
#891=CARTESIAN_POINT ( 'NONE',  ( 14.42366234001531922, 7.375548675892134476, -20.85295579936483179 ) ) ;
#893=CARTESIAN_POINT ( 'NONE',  ( 19.95076809599375878, -1.008983920988137495, -18.52968236344498720 ) ) ;
#904=CARTESIAN_POINT ( 'NONE',  ( 11.70392491148546732, 10.80251906652491556, -16.82536866641744311 ) ) ;
#905=CARTESIAN_POINT ( 'NONE',  ( 35.32886446602115171, -21.19738783794349857, -20.03221113960638178 ) ) ;
#908=CARTESIAN_POINT ( 'NONE',  ( 9.274674406624409784, 15.43775921338471413, -16.98767239532306661 ) ) ;
#909=CARTESIAN_POINT ( 'NONE',  ( 21.18945582756405344, -5.194394521544061227, -16.21196392551894405 ) ) ;
#910=CARTESIAN_POINT ( 'NONE',  ( 12.86796368952119174, 9.515911916162036022, -16.11566496612908139 ) ) ;
#917=CARTESIAN_POINT ( 'NONE',  ( 11.45661370752365116, 9.343864103108954211, -15.86763743611193789 ) ) ;
#923=CARTESIAN_POINT ( 'NONE',  ( 12.67163634847678644, 8.538173360731750705, -16.25940050138558135 ) ) ;
#925=CARTESIAN_POINT ( 'NONE',  ( 36.54859390953723874, -23.18451583373416014, -14.99999999999999822 ) ) ;
#926=CARTESIAN_POINT ( 'NONE',  ( 22.35254782987788147, 5.884919045556002537, -15.62344653218675283 ) ) ;
#927=CARTESIAN_POINT ( 'NONE',  ( 13.40325769311605164, 6.909072298322937122, -18.40730773563142719 ) ) ;
#937=B_SPLINE_CURVE_WITH_KNOTS ( 'NONE', 3,
 ( #12217, #16653, #16799, #14042, #25971, #23835, #3091, #9467, #19090, #18790, #19231, #11762, #12361, #23371, #21080, #2781, #7645, #14198, #9921, #2488, #23526, #26128, #5207, #16949, #7203, #14498, #21672, #773, #338, #10070, #4901, #19384, #5052, #7051, #16340, #21223, #9623, #18944, #14342, #23677, #28297, #21832, #13117, #24429, #12817, #29046, #10826, #1235, #22130, #8082, #3826, #19679, #28904, #28749, #6107, #19534, #29196, #3524, #17392, #8232, #15096, #1095, #24735, #7936, #26736, #5809, #17250, #12967, #29361, #24582, #17544, #10524, #19992, #26578, #3231, #10681, #5662, #10373 ),
 .UNSPECIFIED., .F., .F.,
 ( 4, 2, 2, 2, 2, 2, 2, 2, 2, 2, 2, 2, 2, 2, 2, 2, 2, 2, 2, 2, 2, 2, 2, 2, 2, 2, 2, 2, 2, 2, 2, 2, 2, 2, 2, 2, 2, 2, 4 ),
 ( 0.04625696548573639266, 0.1003381136405422785, 0.1505071704608134109, 0.1755916988709489979, 0.1881339630760167636, 0.1944050951785506465, 0.2006762272810845293, 0.2086934065084689038, 0.2167105857358532783, 0.2327449441906219718, 0.2648136611001593588, 0.2968823780096967457, 0.3129167364644654947, 0.3209339156918498137, 0.3289510949192341327, 0.3346579968240730452, 0.3403648987289118466, 0.3517787025385894495, 0.3746063101579446553, 0.4202615253966550668, 0.5115719558740758899, 0.6028823863514967130, 0.6485376015902071245, 0.6713652092095623303, 0.6827790130192399332, 0.6941928168289175360, 0.7036545619149295883, 0.7131163070009416405, 0.7320397971729657449, 0.7698867775170139538, 0.8077337578610621627, 0.8266572480330862671, 0.8361189931190984304, 0.8455807382051104826, 0.8552319420672911399, 0.8648831459294716861, 0.8841855536538327787, 0.9227903691025551858, 1.000000000000000000 ),
 .UNSPECIFIED. ) ;
#938=CARTESIAN_POINT ( 'NONE',  ( 18.22321846687148650, 1.664438589611230812, -15.57940112478783945 ) ) ;
#940=CARTESIAN_POINT ( 'NONE',  ( 19.91209246711783010, 5.411768277715644615, -14.29674560697521457 ) ) ;
#948=CARTESIAN_POINT ( 'NONE',  ( 12.25159070717542065, 9.517778977577904698, -15.32825133053543887 ) ) ;
#956=CARTESIAN_POINT ( 'NONE',  ( 12.49977518293622758, 8.570603418560722275, -15.13035415120363325 ) ) ;
#959=CARTESIAN_POINT ( 'NONE',  ( 10.58765414998594245, 9.416266744339480965, -16.44470908465386572 ) ) ;
#967=CARTESIAN_POINT ( 'NONE',  ( 12.81602886594196988, 9.615025227323064527, -16.14774825664093783 ) ) ;
#969=CARTESIAN_POINT ( 'NONE',  ( 33.33106278064285277, -11.02967194543584029, -16.07471553095689742 ) ) ;
#970=CARTESIAN_POINT ( 'NONE',  ( 21.19279910686179846, 4.720633506281588510, -19.26595127233560234 ) ) ;
#973=CARTESIAN_POINT ( 'NONE',  ( 18.51594006248351931, 7.284897756227690202, -14.24483590514913089 ) ) ;
#978=CARTESIAN_POINT ( 'NONE',  ( 21.30888034401541731, -0.8953576338359930942, -14.03585182699830369 ) ) ;
#980=CARTESIAN_POINT ( 'NONE',  ( 23.16309603597909472, 3.730466837354933674, -16.34659541137592598 ) ) ;
#992=CARTESIAN_POINT ( 'NONE',  ( 11.47464782381437587, 9.261287281732329291, -15.86016978468419936 ) ) ;
#993=CARTESIAN_POINT ( 'NONE',  ( 27.10702390817755614, -8.414881854042032927, -18.30456363717458146 ) ) ;
#994=CARTESIAN_POINT ( 'NONE',  ( 27.50962693642323131, -9.092369620780022643, -12.61635453147917474 ) ) ;
#997=CARTESIAN_POINT ( 'NONE',  ( 32.00110207675911767, -10.95298233446834502, -16.54939777171900417 ) ) ;
#1008=CARTESIAN_POINT ( 'NONE',  ( 16.89369580670022941, 0.5033910033923695293, -17.32063897790030893 ) ) ;
#1011=CARTESIAN_POINT ( 'NONE',  ( 12.24452513275510235, 9.643158527868859409, -15.32408204131529317 ) ) ;
#1016=CARTESIAN_POINT ( 'NONE',  ( 19.61192361542596529, -2.405681417800469291, -14.70675912396028906 ) ) ;
#1018=CARTESIAN_POINT ( 'NONE',  ( 18.97422388862426601, -0.1098198481195374748, -14.77765307979439058 ) ) ;
#1020=CARTESIAN_POINT ( 'NONE',  ( 35.49237112349044310, -21.93193663806729887, -19.32748734164077931 ) ) ;
#1022=CARTESIAN_POINT ( 'NONE',  ( 30.37590262355644910, -7.260401249342992358, -13.74898149931492775 ) ) ;
#1023=CARTESIAN_POINT ( 'NONE',  ( 24.20684193479931068, 1.026663266619176840, -14.52337054612115708 ) ) ;
#1025=CARTESIAN_POINT ( 'NONE',  ( 28.47856004806874353, -11.16640101040803401, -12.66155532224275149 ) ) ;
#1033=CARTESIAN_POINT ( 'NONE',  ( 34.06228043176686526, -11.34293828116054037, -19.64761387034043949 ) ) ;
#1034=CARTESIAN_POINT ( 'NONE',  ( 11.21346931060482000, 10.45895530107994098, -15.96818619734747458 ) ) ;
#1040=CARTESIAN_POINT ( 'NONE',  ( 11.98759337455738816, 9.501579335558542283, -16.70806177831036976 ) ) ;
#1052=CARTESIAN_POINT ( 'NONE',  ( 13.10901043280714084, 7.538357286119017786, -15.92110722978107873 ) ) ;
#1055=CARTESIAN_POINT ( 'NONE',  ( 15.78898853071975061, 11.08777142890889245, -14.37707943039971781 ) ) ;
#1056=CARTESIAN_POINT ( 'NONE',  ( 26.53548354394225228, -12.81408696708834860, -17.07385457597708367 ) ) ;
#1069=CARTESIAN_POINT ( 'NONE',  ( 12.67163634847678644, 8.538173360731750705, -16.25940050138558135 ) ) ;
#1071=CARTESIAN_POINT ( 'NONE',  ( 33.63121621376239290, -12.57075016180469262, -18.73605167971255980 ) ) ;
#1073=CARTESIAN_POINT ( 'NONE',  ( 9.106918858820071350, 16.20710753947419747, -17.05743340929950946 ) ) ;
#1076=CARTESIAN_POINT ( 'NONE',  ( 26.72358035960067824, -3.685970424986596772, -17.59444040205794835 ) ) ;
#1078=CARTESIAN_POINT ( 'NONE',  ( 12.83223741744420288, 9.540690758033102625, -16.14104544935691976 ) ) ;
#1084=CARTESIAN_POINT ( 'NONE',  ( 12.48484057295006977, 8.564241722236854315, -15.14223913367768759 ) ) ;
#1089=CARTESIAN_POINT ( 'NONE',  ( 12.02685106364323531, 9.321538569219327997, -16.69182734290254899 ) ) ;
#1091=CARTESIAN_POINT ( 'NONE',  ( 13.93547621865856634, 6.828337171336619882, -15.16703734247451507 ) ) ;
#1092=CARTESIAN_POINT ( 'NONE',  ( 26.48263329513011755, -12.06126822337667903, -13.95730679897583038 ) ) ;
#1095=CARTESIAN_POINT ( 'NONE',  ( 36.52322468491136220, -22.07054534594105988, -19.04503427665075321 ) ) ;
#1098=CARTESIAN_POINT ( 'NONE',  ( 19.48014203372339992, 3.175912578606837844, -18.88683143354647243 ) ) ;
#1099=CARTESIAN_POINT ( 'NONE',  ( 20.23291344124205793, 5.521974472852556381, -14.51730806008046137 ) ) ;
#1108=CARTESIAN_POINT ( 'NONE',  ( 12.27009251048667160, 9.509012028593735621, -15.31479730457434307 ) ) ;
#1113=CARTESIAN_POINT ( 'NONE',  ( 12.49860086554322436, 8.570087612320898884, -15.13128986298120537 ) ) ;
#1116=CARTESIAN_POINT ( 'NONE',  ( 10.90022735844294388, 8.411956631741958290, -16.28271526948893921 ) ) ;
#1123=CARTESIAN_POINT ( 'NONE',  ( 11.60030688134799171, 15.19048121717941768, -16.65049206281727479 ) ) ;
#1124=CARTESIAN_POINT ( 'NONE',  ( 33.69236230569678980, -11.08454582564024449, -17.09586691508924972 ) ) ;
#1125=CARTESIAN_POINT ( 'NONE',  ( 19.23836061553175369, 5.151828676608854352, -13.99136221198299168 ) ) ;
#1128=CARTESIAN_POINT ( 'NONE',  ( 16.36264732604271899, 7.873549196589271659, -20.78255227469630739 ) ) ;
#1131=CARTESIAN_POINT ( 'NONE',  ( 26.39122182234759961, -2.132411660323914049, -15.07701415690354274 ) ) ;
#1132=CARTESIAN_POINT ( 'NONE',  ( 20.97462796522363959, -1.010871063906457534, -12.65628865346789134 ) ) ;
#1142=CARTESIAN_POINT ( 'NONE',  ( 11.47257016429183452, 9.270685755423764718, -15.86103888016343255 ) ) ;
#1143=CARTESIAN_POINT ( 'NONE',  ( 16.53304876882650731, 8.555045913257369961, -19.77053526944897754 ) ) ;
#1144=CARTESIAN_POINT ( 'NONE',  ( 22.75855789899217640, -7.280205122891536540, -14.30210469086359915 ) ) ;
#1152=CARTESIAN_POINT ( 'NONE',  ( 20.99533150354982070, 4.487273811465053441, -19.54336078777620500 ) ) ;
#1156=CARTESIAN_POINT ( 'NONE',  ( 12.27630411038995106, 9.497004473356668086, -15.31097170929839812 ) ) ;
#1157=CARTESIAN_POINT ( 'NONE',  ( 32.57315965809380742, -11.03986597812349935, -18.16622079659612510 ) ) ;
#1159=CARTESIAN_POINT ( 'NONE',  ( 17.72480397827495224, 1.356124466512965476, -19.40231245121514903 ) ) ;
#1161=CARTESIAN_POINT ( 'NONE',  ( 20.68391251823057075, 0.6588762160484964436, -13.99488169736409304 ) ) ;
#1164=CARTESIAN_POINT ( 'NONE',  ( 30.91631662189391250, -8.208988707411489116, -18.28093047724294351 ) ) ;
#1165=CARTESIAN_POINT ( 'NONE',  ( 22.59259966355045890, -3.831908474886262184, -12.47183693924707804 ) ) ;
#1169=EDGE_CURVE ( 'NONE', #8937, #4557, #27768, .T. ) ;
#1180=CARTESIAN_POINT ( 'NONE',  ( 34.36632712588347260, -12.38074715364594347, -19.93031689919964222 ) ) ;
#1181=CARTESIAN_POINT ( 'NONE',  ( 9.916411867603999397, 16.40742607105030260, -16.50456570466356965 ) ) ;
#1185=CARTESIAN_POINT ( 'NONE',  ( 9.661883061612440926, 16.25482663361732705, -17.91796598306941135 ) ) ;
#1196=CARTESIAN_POINT ( 'NONE',  ( 8.944584663113916534, 16.95159285377954461, -17.91618150236991269 ) ) ;
#1198=CARTESIAN_POINT ( 'NONE',  ( 15.41439956623108642, 10.93483300904300215, -14.25553973300288568 ) ) ;
#1199=CARTESIAN_POINT ( 'NONE',  ( 27.03959252790357581, -7.665547941290169476, -19.57376043866218041 ) ) ;
#1212=CARTESIAN_POINT ( 'NONE',  ( 12.02859841272590735, 9.313533661810568631, -16.69110409223909741 ) ) ;
#1213=CARTESIAN_POINT ( 'NONE',  ( 33.51257387524950815, -12.16639167148776224, -18.62538556556795655 ) ) ;
#1215=CARTESIAN_POINT ( 'NONE',  ( 9.008298112641352162, 16.65939485267133335, -17.25320607661530303 ) ) ;
#1216=CARTESIAN_POINT ( 'NONE',  ( 23.21730923944814506, -4.364887171357101359, -13.63095412955673247 ) ) ;
#1217=CARTESIAN_POINT ( 'NONE',  ( 10.35865474790814211, 16.97209951875106526, -17.91014213605047445 ) ) ;
#1222=CARTESIAN_POINT ( 'NONE',  ( 11.47304865262203499, 9.268493388164605662, -15.86084085272616484 ) ) ;
#1228=CARTESIAN_POINT ( 'NONE',  ( 12.14965596459611774, 8.983642127099937369, -16.62385966901067391 ) ) ;
#1230=CARTESIAN_POINT ( 'NONE',  ( 20.25609397779747312, 2.611002146465201346, -20.92159891259701610 ) ) ;
#1231=CARTESIAN_POINT ( 'NONE',  ( 20.53425600248055005, 0.8933117467920750343, -13.02782074225586406 ) ) ;
#1235=CARTESIAN_POINT ( 'NONE',  ( 35.97124720801268438, -19.59080293283771823, -20.41544573823858144 ) ) ;
#1238=CARTESIAN_POINT ( 'NONE',  ( 17.88091890332929523, 4.544920326333207861, -13.91018511019278669 ) ) ;
#1246=CARTESIAN_POINT ( 'NONE',  ( 31.49119590023542870, -10.87553819600004701, -15.10823507476435523 ) ) ;
#1249=CARTESIAN_POINT ( 'NONE',  ( 11.05541531668977662, 17.68942339022145305, -17.92454625180715411 ) ) ;
#1255=CARTESIAN_POINT ( 'NONE',  ( 12.49957999542663600, 8.570517509188613658, -15.13050969259218981 ) ) ;
#1258=CARTESIAN_POINT ( 'NONE',  ( 10.67240773364005868, 9.027839897374207112, -16.40964036978800777 ) ) ;
#1265=CARTESIAN_POINT ( 'NONE',  ( 12.83192189813640738, 9.542137755788996145, -16.14117592875819440 ) ) ;
#1267=CARTESIAN_POINT ( 'NONE',  ( 34.59231264378541937, -12.39598037772099559, -18.95630535174095499 ) ) ;
#1268=CARTESIAN_POINT ( 'NONE',  ( 22.34083945069921739, -4.755659482961629436, -14.12236044035638116 ) ) ;
#1272=CARTESIAN_POINT ( 'NONE',  ( 18.47844294452917424, 10.16049799425131361, -18.92511192449534718 ) ) ;
#1275=CARTESIAN_POINT ( 'NONE',  ( 21.00058363250239069, -3.857595149258782996, -18.17417979037076847 ) ) ;
#1276=CARTESIAN_POINT ( 'NONE',  ( 18.66675855576620791, -1.414919486740021881, -19.12600662388792117 ) ) ;
#1290=CARTESIAN_POINT ( 'NONE',  ( 11.47250673971808688, 9.270976631574885829, -15.86106510822916249 ) ) ;
#1291=CARTESIAN_POINT ( 'NONE',  ( 26.84208138670940968, -2.489200896322508516, -17.35162900556907317 ) ) ;
#1299=CARTESIAN_POINT ( 'NONE',  ( 19.25770813156441008, -2.543370271471735222, -15.40753146551623587 ) ) ;
#1303=CARTESIAN_POINT ( 'NONE',  ( 12.25668235260104844, 9.587403967970216101, -15.31905460325341117 ) ) ;
#1306=CARTESIAN_POINT ( 'NONE',  ( 32.00110207675911767, -10.95298233446834502, -16.54939777171900417 ) ) ;
#1309=CARTESIAN_POINT ( 'NONE',  ( 19.50856600871340873, -1.908691058934758100, -18.90332006808282728 ) ) ;
#1311=CARTESIAN_POINT ( 'NONE',  ( 18.41232452102509143, -0.3525767977158695277, -15.58598945151665305 ) ) ;
#1314=CARTESIAN_POINT ( 'NONE',  ( 22.23398510282979146, -6.138177547518383292, -17.55864386164050472 ) ) ;
#1316=CARTESIAN_POINT ( 'NONE',  ( 22.08361411416106534, -2.618483922437499611, -20.46533185456077319 ) ) ;
#1327=CARTESIAN_POINT ( 'NONE',  ( 28.80153578082395427, -7.039779562103731791, -13.29052886957691371 ) ) ;
#1328=CARTESIAN_POINT ( 'NONE',  ( 13.15390973649967599, 8.859676595473322536, -14.60899741038990562 ) ) ;
#1329=CARTESIAN_POINT ( 'NONE',  ( 36.54779501103016770, -22.18092680593016652, -18.48200341583098449 ) ) ;
#1332=CARTESIAN_POINT ( 'NONE',  ( 9.917332382238186028, 16.40320447359955125, -16.50418441153501448 ) ) ;
#1336=CARTESIAN_POINT ( 'NONE',  ( 9.661883061612440926, 16.25482663361732705, -17.91928203681695564 ) ) ;
#1340=CARTESIAN_POINT ( 'NONE',  ( 9.924804006935172396, 16.36893865032855899, -16.50109463189289016 ) ) ;
#1349=CARTESIAN_POINT ( 'NONE',  ( 8.944584683310379702, 16.95159276115599667, -23.00000000000000711 ) ) ;
#1351=CARTESIAN_POINT ( 'NONE',  ( 27.68941694697105760, -11.75984073208553582, -11.85267853464266352 ) ) ;
#1352=CARTESIAN_POINT ( 'NONE',  ( 25.66600519952783799, -8.909200411882650883, -19.30012332941604924 ) ) ;
#1364=CARTESIAN_POINT ( 'NONE',  ( 13.11043623405165448, 8.565188957795726310, -15.92239833454181230 ) ) ;
#1365=CARTESIAN_POINT ( 'NONE',  ( 32.61797162530606187, -11.69648652134232414, -16.29118568026193614 ) ) ;
#1367=CARTESIAN_POINT ( 'NONE',  ( 9.112490548836888138, 16.18155505883174783, -17.05474119751274031 ) ) ;
#1370=CARTESIAN_POINT ( 'NONE',  ( 21.43917814492346707, -4.799604530101110988, -17.97822123721208243 ) ) ;
#1371=CARTESIAN_POINT ( 'NONE',  ( 13.00452062571394229, 9.576253617860157163, -16.00682707811506233 ) ) ;
#1377=CARTESIAN_POINT ( 'NONE',  ( 11.47276097331165623, 9.269810413962238371, -15.86095999428340697 ) ) ;
#1384=CARTESIAN_POINT ( 'NONE',  ( 9.661883061612440926, 16.25482663361732705, -17.98596209335946128 ) ) ;
#1386=CARTESIAN_POINT ( 'NONE',  ( 22.56675539556120924, 5.189497681140571750, -18.50903523470404011 ) ) ;
#1387=CARTESIAN_POINT ( 'NONE',  ( 19.63206833423595299, 9.033623817254925470, -16.13982763006638166 ) ) ;
#1392=CARTESIAN_POINT ( 'NONE',  ( 16.53304876882650731, 8.555045913257369961, -19.77053526944897754 ) ) ;
#1400=CARTESIAN_POINT ( 'NONE',  ( 33.57712230886461668, -13.32773824946660923, -19.76201999124979736 ) ) ;
#1405=CARTESIAN_POINT ( 'NONE',  ( 12.35402573141577598, 9.564223303342972216, -15.24651908135525957 ) ) ;
#1408=CARTESIAN_POINT ( 'NONE',  ( 13.04501788334644630, 8.811555337407297017, -14.69578613943112799 ) ) ;
#1411=CARTESIAN_POINT ( 'NONE',  ( 10.66667607898454939, 9.053862104998891880, -16.41203073725236905 ) ) ;
#1414=EDGE_CURVE ( 'NONE', #4557, #23709, #24844, .T. ) ;
#1416=CARTESIAN_POINT ( 'NONE',  ( 13.77718166750865869, 8.859676595473324312, -15.39100258941132182 ) ) ;
#1419=CARTESIAN_POINT ( 'NONE',  ( 12.86818510107347890, 9.516005823298000266, -16.11548879760486130 ) ) ;
#1421=CARTESIAN_POINT ( 'NONE',  ( 36.25073006198487491, -19.84637134955221072, -19.45760515208133512 ) ) ;
#1422=CARTESIAN_POINT ( 'NONE',  ( 23.66601916330066402, 2.199037240492611733, -18.57254039386976885 ) ) ;
#1429=CARTESIAN_POINT ( 'NONE',  ( 26.64416741123070054, -12.70369174447049332, -17.39020166599120643 ) ) ;
#1430=CARTESIAN_POINT ( 'NONE',  ( 18.16797961131436523, 4.950584380424773556, -14.83967967756414730 ) ) ;
#1440=CARTESIAN_POINT ( 'NONE',  ( 11.19157713609530269, 9.239454617397717229, -17.25496879848155629 ) ) ;
#1441=CARTESIAN_POINT ( 'NONE',  ( 12.48484057295006977, 8.564241722236854315, -15.14223913367768759 ) ) ;
#1443=CARTESIAN_POINT ( 'NONE',  ( 23.54468722040186890, -6.934586491718037315, -13.40271233150634878 ) ) ;
#1455=CARTESIAN_POINT ( 'NONE',  ( 26.84970692451943819, -5.812874930055231815, -14.04107299160273037 ) ) ;
#1459=CARTESIAN_POINT ( 'NONE',  ( 10.78565875124225393, 16.33370571569710705, -15.92737460872590738 ) ) ;
#1460=FACE_OUTER_BOUND ( 'NONE', #27089, .T. ) ;
#1462=CARTESIAN_POINT ( 'NONE',  ( 22.09544204423535874, -4.864148257255451746, -14.35781331922719772 ) ) ;
#1464=CARTESIAN_POINT ( 'NONE',  ( 20.51677437365689372, 7.544110930723523012, -19.48516728630390915 ) ) ;
#1468=CARTESIAN_POINT ( 'NONE',  ( 25.64694198568010819, -13.68525919019184300, -15.02544717525507778 ) ) ;
#1469=CARTESIAN_POINT ( 'NONE',  ( 27.64540148246904749, -2.072091111371471506, -15.50399641584551702 ) ) ;
#1473=CARTESIAN_POINT ( 'NONE',  ( 27.20760296572909809, -8.488227175050779394, -13.35743234967312354 ) ) ;
#1479=MANIFOLD_SOLID_BREP ( 'Sweep3', #18491 ) ;
#1484=CARTESIAN_POINT ( 'NONE',  ( 23.44948677240984480, -6.246615351793893822, -14.99377964970044808 ) ) ;
#1486=CARTESIAN_POINT ( 'NONE',  ( 32.94969931363368687, -9.746457777152386370, -18.95700739231402920 ) ) ;
#1489=CARTESIAN_POINT ( 'NONE',  ( 9.916824447075894611, 16.40553392900050156, -16.50439446175997205 ) ) ;
#1493=CARTESIAN_POINT ( 'NONE',  ( 9.661884236495001943, 16.25482124545614937, -17.91517755594902894 ) ) ;
#1496=CARTESIAN_POINT ( 'NONE',  ( 11.49350937636955372, 9.187954247928445284, -15.85136552863131421 ) ) ;
#1500=CARTESIAN_POINT ( 'NONE',  ( 17.32873655921053313, 10.26331207550778579, -16.20725374984683143 ) ) ;
#1503=CARTESIAN_POINT ( 'NONE',  ( 8.944589832665828411, 16.95156914555548866, -17.90909639166975609 ) ) ;
#1504=CARTESIAN_POINT ( 'NONE',  ( 31.74553205326546390, -10.26435202779689604, -17.82876124730869805 ) ) ;
#1506=CARTESIAN_POINT ( 'NONE',  ( 13.62270618888621776, 10.12723052195839024, -14.35540206260209573 ) ) ;
#1508=CARTESIAN_POINT ( 'NONE',  ( 26.83671086236671144, -5.482767762337403816, -13.01846673106422436 ) ) ;
#1516=( NAMED_UNIT ( * ) SI_UNIT ( $, .STERADIAN. ) SOLID_ANGLE_UNIT ( ) );
#1522=CARTESIAN_POINT ( 'NONE',  ( 13.19188795686497429, 8.601024833420110483, -15.85749200792911573 ) ) ;
#1523=CARTESIAN_POINT ( 'NONE',  ( 33.45149595566165601, -11.04796323883829423, -16.41509932566969354 ) ) ;
#1526=CARTESIAN_POINT ( 'NONE',  ( 9.112705230111354027, 16.18057050314154210, -17.05465234812585607 ) ) ;
#1529=CARTESIAN_POINT ( 'NONE',  ( 10.35864918915110877, 16.97212501191939538, -17.92981046679734547 ) ) ;
#1534=CARTESIAN_POINT ( 'NONE',  ( 11.47652547240386944, 9.253065934422213701, -15.85936358228339316 ) ) ;
#1538=CARTESIAN_POINT ( 'NONE',  ( 9.661883061612440926, 16.25482663361732705, -17.92981046679734547 ) ) ;
#1539=CARTESIAN_POINT ( 'NONE',  ( 13.26656245924271005, 6.725567473591735457, -17.69027979179009691 ) ) ;
#1540=CARTESIAN_POINT ( 'NONE',  ( 14.64418905516944314, 2.941711854493593403, -16.63492386420942282 ) ) ;
#1547=CARTESIAN_POINT ( 'NONE',  ( 22.89472691350227507, 1.279074496056108901, -19.72372301458170796 ) ) ;
#1556=CARTESIAN_POINT ( 'NONE',  ( 32.45272648307624053, -11.02157468472264412, -17.82583700188536824 ) ) ;
#1561=CARTESIAN_POINT ( 'NONE',  ( 11.05541531668977662, 17.68942339022145305, -17.92981046679734547 ) ) ;
#1562=CARTESIAN_POINT ( 'NONE',  ( 35.54859661768235668, -23.18452799999607805, -18.25366188177437365 ) ) ;
#1564=CARTESIAN_POINT ( 'NONE',  ( 9.641350810849047548, 17.66889113945805789, -23.00000000000000711 ) ) ;
#1565=CARTESIAN_POINT ( 'NONE',  ( 10.66059746906157635, 9.081739384948186000, -16.41454445628326297 ) ) ;
#1571=CARTESIAN_POINT ( 'NONE',  ( 10.35864918915110877, 16.97212501191939538, -17.92454625180715766 ) ) ;
#1572=CARTESIAN_POINT ( 'NONE',  ( 33.42826320546385688, -10.41623213582910523, -18.33855703361424361 ) ) ;
#1573=CARTESIAN_POINT ( 'NONE',  ( 24.79644250101478065, -1.608028467720058918, -19.02763285027648976 ) ) ;
#1582=CARTESIAN_POINT ( 'NONE',  ( 29.00434111665888182, -5.389956126880047549, -17.18324766788818181 ) ) ;
#1583=CARTESIAN_POINT ( 'NONE',  ( 26.07721637849146390, 0.4197350235787081774, -17.11807909718082144 ) ) ;
#1597=CARTESIAN_POINT ( 'NONE',  ( 12.60230244812736800, 7.534144488243946114, -16.30820540178382316 ) ) ;
#1598=CARTESIAN_POINT ( 'NONE',  ( 12.50906579366657390, 8.574708520419219937, -15.12294941509656354 ) ) ;
#1599=CARTESIAN_POINT ( 'NONE',  ( 30.50415327504139285, -11.36213899161910135, -13.19862950667920565 ) ) ;
#1604=CARTESIAN_POINT ( 'NONE',  ( 9.641350810849047548, 17.66889113945805789, -23.00000000000000711 ) ) ;
#1609=CARTESIAN_POINT ( 'NONE',  ( 25.04068920418659161, -5.475481712173364990, -18.92835678451453774 ) ) ;
#1612=CARTESIAN_POINT ( 'NONE',  ( 12.24516467974477152, 9.516115653471018732, -15.33328326133307762 ) ) ;
#1613=CARTESIAN_POINT ( 'NONE',  ( 32.74314609665832165, -11.10724048739539782, -18.62249297335446840 ) ) ;
#1615=CARTESIAN_POINT ( 'NONE',  ( 27.31974442496251143, -5.660127319198639206, -14.41990313654811651 ) ) ;
#1617=CARTESIAN_POINT ( 'NONE',  ( 22.60936069168443652, -2.585520780102871896, -18.46111163327002913 ) ) ;
#1620=CARTESIAN_POINT ( 'NONE',  ( 13.93479307118181509, 9.207276677253689812, -14.11477394318545286 ) ) ;
#1622=CARTESIAN_POINT ( 'NONE',  ( 26.83635784119175938, -3.902057423304301942, -19.75319010936098962 ) ) ;
#1625=CARTESIAN_POINT ( 'NONE',  ( 26.87449084144840938, -11.88902188497427481, -13.49525739704605343 ) ) ;
#1635=CARTESIAN_POINT ( 'NONE',  ( 25.76376746566330311, -3.589579415956118069, -17.31313795625071350 ) ) ;
#1636=CARTESIAN_POINT ( 'NONE',  ( 15.33641899704135980, 5.898237403637139664, -14.35162154369138676 ) ) ;
#1637=CARTESIAN_POINT ( 'NONE',  ( 32.63927297112797277, -9.624974391992262568, -18.12286679007055312 ) ) ;
#1639=CARTESIAN_POINT ( 'NONE',  ( 11.48043977940431226, 9.236673419044803879, -15.85762597608872326 ) ) ;
#1642=CARTESIAN_POINT ( 'NONE',  ( 9.661883061612440926, 16.25482663361732705, -23.00000000000000711 ) ) ;
#1646=CARTESIAN_POINT ( 'NONE',  ( 12.50268541164654756, 8.571888915454989544, -15.12803469218787811 ) ) ;
#1654=CARTESIAN_POINT ( 'NONE',  ( 8.945901566930443138, 16.94555336501101550, -17.80918358208353069 ) ) ;
#1655=CARTESIAN_POINT ( 'NONE',  ( 32.24963562184495203, -10.43994945000269148, -19.19593526939238970 ) ) ;
#1657=CARTESIAN_POINT ( 'NONE',  ( 17.78670086218314239, 4.747145650100266678, -21.23922340053293212 ) ) ;
#1658=CARTESIAN_POINT ( 'NONE',  ( 30.68845550234816244, -8.154108532121835395, -15.50657635367809917 ) ) ;
#1663=CARTESIAN_POINT ( 'NONE',  ( 19.79992434292498515, 0.1278105412470878222, -19.37491769885296122 ) ) ;
#1671=CARTESIAN_POINT ( 'NONE',  ( 13.12341270237516078, 8.570764515250925086, -15.91206798513452192 ) ) ;
#1672=CARTESIAN_POINT ( 'NONE',  ( 33.91010249890941708, -13.82364185882242147, -18.82035036639317482 ) ) ;
#1674=CARTESIAN_POINT ( 'NONE',  ( 12.74961974476379289, 7.623002797808662301, -14.93122222525392928 ) ) ;
#1676=CARTESIAN_POINT ( 'NONE',  ( 28.06689949639850212, -8.111051215268487269, -13.49421662364394514 ) ) ;
#1677=CARTESIAN_POINT ( 'NONE',  ( 10.35864918915110877, 16.97212501191939538, -17.91796598306941135 ) ) ;
#1686=CARTESIAN_POINT ( 'NONE',  ( 9.661883061612440926, 16.25482663361732705, -17.94384837343789130 ) ) ;
#1688=CARTESIAN_POINT ( 'NONE',  ( 24.81022290780906658, -1.767900772465358372, -17.79475844156381470 ) ) ;
#1689=CARTESIAN_POINT ( 'NONE',  ( 14.98730560944732559, 2.974898859484017333, -15.20016081292634169 ) ) ;
#1693=CARTESIAN_POINT ( 'NONE',  ( 17.55424633453837302, 0.6138019359854992585, -14.89346452969079060 ) ) ;
#1699=CARTESIAN_POINT ( 'NONE',  ( 32.57315965809380742, -11.03986597812349935, -18.16622079659612510 ) ) ;
#1705=CARTESIAN_POINT ( 'NONE',  ( 16.75072914628186282, 8.771658487634226731, -19.67538163746542779 ) ) ;
#1706=CARTESIAN_POINT ( 'NONE',  ( 12.24670349824113380, 9.516721811805902931, -15.33206243003379754 ) ) ;
#1707=CARTESIAN_POINT ( 'NONE',  ( 35.16668739017224965, -20.46881214373840763, -20.22602438870426766 ) ) ;
#1710=CARTESIAN_POINT ( 'NONE',  ( 9.641359250860388030, 17.66885243249017634, -17.90483003768722625 ) ) ;
#1717=CARTESIAN_POINT ( 'NONE',  ( 10.35864919943752405, 16.97212496474457311, -17.91550491156534974 ) ) ;
#1720=CARTESIAN_POINT ( 'NONE',  ( 36.54859390953724585, -21.18451583373416014, -16.94733705004010105 ) ) ;
#1721=CARTESIAN_POINT ( 'NONE',  ( 25.31619048431776875, -0.2099727537683927225, -15.56338435260822628 ) ) ;
#1730=CARTESIAN_POINT ( 'NONE',  ( 25.71810023473615203, -5.953606672203104466, -12.71518937071605038 ) ) ;
#1731=CARTESIAN_POINT ( 'NONE',  ( 26.19520757255249066, -7.109971961106261951, -13.37903969216112898 ) ) ;
#1740=CARTESIAN_POINT ( 'NONE',  ( 13.24589568141979612, 7.574869496316740225, -15.81383618087551746 ) ) ;
#1741=CARTESIAN_POINT ( 'NONE',  ( 12.50076791318051761, 8.571041463825640250, -15.12956297801270900 ) ) ;
#1742=CARTESIAN_POINT ( 'NONE',  ( 26.46413748225140594, -13.10274310649288942, -15.24000415025259692 ) ) ;
#1747=CARTESIAN_POINT ( 'NONE',  ( 9.675370519060759733, 17.51287242109451014, -17.23928541814325399 ) ) ;
#1752=CARTESIAN_POINT ( 'NONE',  ( 21.42923412144385509, -1.598955984811285536, -13.33006947543598741 ) ) ;
#1756=CARTESIAN_POINT ( 'NONE',  ( 11.05541531668977662, 17.68942339022145305, -17.92279151347708677 ) ) ;
#1758=CARTESIAN_POINT ( 'NONE',  ( 33.38708106686501509, -12.47399286361455850, -19.70456970583452616 ) ) ;
#1763=CARTESIAN_POINT ( 'NONE',  ( 25.67262840375075328, -3.322766148301121714, -14.04542551033457798 ) ) ;
#1766=CARTESIAN_POINT ( 'NONE',  ( 24.12901349891383163, -0.6887463444711696692, -16.28517635256633156 ) ) ;
#1770=CARTESIAN_POINT ( 'NONE',  ( 26.55441479597953247, -12.51626325376082249, -18.99724541349076645 ) ) ;
#1771=CARTESIAN_POINT ( 'NONE',  ( 29.20193236150002392, -6.731655735042891386, -17.98962132073140552 ) ) ;
#1782=CARTESIAN_POINT ( 'NONE',  ( 9.641350810849047548, 17.66889113945805789, -19.66666666666842644 ) ) ;
#1783=CARTESIAN_POINT ( 'NONE',  ( 23.18962843369624949, -6.128656054388458507, -17.19981796389819095 ) ) ;
#1784=CARTESIAN_POINT ( 'NONE',  ( 18.54205238286641588, 5.219565156008159512, -20.23764637224795848 ) ) ;
#1785=CARTESIAN_POINT ( 'NONE',  ( 35.88008189734257769, -20.18124548360443882, -21.42481968387543390 ) ) ;
#1787=CARTESIAN_POINT ( 'NONE',  ( 11.46471852075427478, 9.306694396509932687, -15.86428581073749378 ) ) ;
#1790=CARTESIAN_POINT ( 'NONE',  ( 9.667746079407143256, 16.22793808664985704, -17.88513208046981617 ) ) ;
#1794=CARTESIAN_POINT ( 'NONE',  ( 12.50162201464318557, 8.571418981294288031, -15.12888223836978341 ) ) ;
#1807=CARTESIAN_POINT ( 'NONE',  ( 13.38138208201938895, 7.626735917299793499, -15.70646184538344770 ) ) ;
#1808=CARTESIAN_POINT ( 'NONE',  ( 35.47777500975636400, -18.37389374556380517, -21.30860247919107664 ) ) ;
#1810=CARTESIAN_POINT ( 'NONE',  ( 22.56790106455553868, 4.272635385308135803, -18.10442882813315535 ) ) ;
#1811=CARTESIAN_POINT ( 'NONE',  ( 17.46640274557904959, 4.060524459741898795, -18.82505950134852313 ) ) ;
#1814=CARTESIAN_POINT ( 'NONE',  ( 27.77130384954419995, -2.130748013457071099, -15.99611347415175366 ) ) ;
#1825=CARTESIAN_POINT ( 'NONE',  ( 33.92041909680281719, -11.11917911243856238, -17.74043268107170235 ) ) ;
#1828=CARTESIAN_POINT ( 'NONE',  ( 10.67240773364005868, 9.027839897374207112, -16.40964036978800777 ) ) ;
#1830=CARTESIAN_POINT ( 'NONE',  ( 31.59793210864275537, -10.01186915388335485, -14.42687813506083039 ) ) ;
#1832=CARTESIAN_POINT ( 'NONE',  ( 10.35864940629342890, 16.97212401607702148, -17.91464645457531191 ) ) ;
#1848=CARTESIAN_POINT ( 'NONE',  ( 13.12048998592846871, 8.569482736746577345, -15.91439669260688561 ) ) ;
#1851=CARTESIAN_POINT ( 'NONE',  ( 24.88259999727891625, -1.109419405293186944, -15.69091174474707451 ) ) ;
#1852=CARTESIAN_POINT ( 'NONE',  ( 16.98604603105943767, -0.4850832133139416080, -17.48051239862526884 ) ) ;
#1853=CARTESIAN_POINT ( 'NONE',  ( 13.86827785273622737, 5.312354197023893221, -16.63408457058017120 ) ) ;
#1857=CARTESIAN_POINT ( 'NONE',  ( 21.10023079691774228, -0.4353598523292347422, -20.14113737667230097 ) ) ;
#1863=CARTESIAN_POINT ( 'NONE',  ( 10.35864918915111055, 16.97212501191939182, -23.00000000000000711 ) ) ;
#1864=CARTESIAN_POINT ( 'NONE',  ( 32.30218501430429967, -10.99871056796995816, -17.40035725849610060 ) ) ;
#1869=CARTESIAN_POINT ( 'NONE',  ( 14.57776618122778700, 6.338444840345393239, -15.85465340776532095 ) ) ;
#1870=CARTESIAN_POINT ( 'NONE',  ( 12.25874535991881764, 9.522117202545773651, -15.32245921924925902 ) ) ;
#1871=CARTESIAN_POINT ( 'NONE',  ( 35.12509383387676820, -20.28195432802065312, -20.22992657050740917 ) ) ;
#1874=CARTESIAN_POINT ( 'NONE',  ( 12.75639466810640776, 7.625977817552541005, -14.92582393630036108 ) ) ;
#1879=CARTESIAN_POINT ( 'NONE',  ( 12.86836073382838563, 9.516082146233362238, -16.11534891376273748 ) ) ;
#1880=CARTESIAN_POINT ( 'NONE',  ( 36.54859390953724585, -21.18451583373416014, -18.19919658220850422 ) ) ;
#1881=CARTESIAN_POINT ( 'NONE',  ( 24.52797215547132836, -1.897736678990579184, -19.26084780660264073 ) ) ;
#1887=CARTESIAN_POINT ( 'NONE',  ( 23.43951749033787735, -6.062008688038916127, -19.28752554440484701 ) ) ;
#1889=CARTESIAN_POINT ( 'NONE',  ( 21.35588827150667512, -4.635113535248831518, -19.58358080364444476 ) ) ;
#1898=CARTESIAN_POINT ( 'NONE',  ( 12.44984726620633353, 8.550925603015029353, -15.16996558791898231 ) ) ;
#1904=CARTESIAN_POINT ( 'NONE',  ( 9.641350810849047548, 17.66889113945805789, -17.94384837343789485 ) ) ;
#1905=CARTESIAN_POINT ( 'NONE',  ( 29.62334656761623819, -11.49549692320935890, -13.92735753183835712 ) ) ;
#1909=CARTESIAN_POINT ( 'NONE',  ( 22.86252235622482587, -0.9498377794471745128, -13.29674124224850118 ) ) ;
#1914=CARTESIAN_POINT ( 'NONE',  ( 11.05541531668977662, 17.68942339022145305, -17.91796598306941135 ) ) ;
#1915=CARTESIAN_POINT ( 'NONE',  ( 35.54859390953724585, -22.18451583373416014, -17.78191007148576475 ) ) ;
#1917=CARTESIAN_POINT ( 'NONE',  ( 21.54098841764929873, -5.100688324319140321, -15.19385678519978633 ) ) ;
#1919=CARTESIAN_POINT ( 'NONE',  ( 20.43449928165676965, -1.849542096390112356, -17.64764676960594869 ) ) ;
#1922=PRESENTATION_STYLE_ASSIGNMENT (( #22522 ) ) ;
#1923=CARTESIAN_POINT ( 'NONE',  ( 16.22940209442605308, 10.22534693890197133, -14.12725775589269084 ) ) ;
#1924=CARTESIAN_POINT ( 'NONE',  ( 28.05683000375443825, -12.20169833507544865, -14.26034257730772126 ) ) ;
#1938=CARTESIAN_POINT ( 'NONE',  ( 24.36960067559809318, -5.041758482997499513, -18.26785210147486538 ) ) ;
#1939=CARTESIAN_POINT ( 'NONE',  ( 18.51594006248351931, 7.284897756227690202, -14.24483590514913089 ) ) ;
#1940=CARTESIAN_POINT ( 'NONE',  ( 32.09732368354767118, -9.542663571685382706, -16.59113971387166941 ) ) ;
#1942=CARTESIAN_POINT ( 'NONE',  ( 12.13006862794127017, 8.527244997094612700, -15.41586291625151972 ) ) ;
#1945=CARTESIAN_POINT ( 'NONE',  ( 9.667069921042207525, 16.23103903510144619, -17.88562738470040969 ) ) ;
#1949=CARTESIAN_POINT ( 'NONE',  ( 12.44984726620633353, 8.550925603015029353, -15.16996558791898231 ) ) ;
#1956=CARTESIAN_POINT ( 'NONE',  ( 9.112356771736518368, 16.18216857766665484, -17.05479705382001399 ) ) ;
#1957=CARTESIAN_POINT ( 'NONE',  ( 34.79556486487921774, -19.80155522666461465, -21.17264749384332134 ) ) ;
#1959=CARTESIAN_POINT ( 'NONE',  ( 17.27385296224481337, 7.553222137591894203, -13.16260341916398069 ) ) ;
#1960=CARTESIAN_POINT ( 'NONE',  ( 27.03191753302054323, -12.88672130028117735, -14.08881772908025454 ) ) ;
#1962=CARTESIAN_POINT ( 'NONE',  ( 23.51547714073238282, 0.8170344765809651744, -13.87895193235286051 ) ) ;
#1977=CARTESIAN_POINT ( 'NONE',  ( 34.22536682013040377, -11.37642754387024979, -18.47965768629886085 ) ) ;
#1979=CARTESIAN_POINT ( 'NONE',  ( 12.33231149932895221, 7.515762311178675326, -15.25793818847554562 ) ) ;
#1981=CARTESIAN_POINT ( 'NONE',  ( 24.60501232743784783, -9.531698448777172317, -16.22453333552994792 ) ) ;
#1983=CARTESIAN_POINT ( 'NONE',  ( 10.46247360472336041, 16.49597300757040230, -17.34042816522791952 ) ) ;
#1989=CARTESIAN_POINT ( 'NONE',  ( 12.50098444160134470, 8.571137227758441668, -15.12939039523150520 ) ) ;
#1994=CARTESIAN_POINT ( 'NONE',  ( 9.661883061612440926, 16.25482663361732705, -17.93331994345748726 ) ) ;
#1996=CARTESIAN_POINT ( 'NONE',  ( 20.60316120045176902, -2.756227665500133206, -14.85995437523845553 ) ) ;
#1997=CARTESIAN_POINT ( 'NONE',  ( 24.59799960276797393, -1.134526835705675918, -15.12159415400816975 ) ) ;
#1998=CARTESIAN_POINT ( 'NONE',  ( 21.58357356133149807, 4.347441036859617469, -17.91576365920758107 ) ) ;
#2001=CARTESIAN_POINT ( 'NONE',  ( 19.02541433733466647, 1.263421280649871248, -13.57496312174407826 ) ) ;
#2010=CARTESIAN_POINT ( 'NONE',  ( 10.35864953657871190, 16.97212341857210660, -17.91436492910080247 ) ) ;
#2016=CARTESIAN_POINT ( 'NONE',  ( 14.29829396236512729, 6.476847147513518088, -18.28004444394726491 ) ) ;
#2017=CARTESIAN_POINT ( 'NONE',  ( 11.05610776857519184, 17.68624771760786274, -17.82814161748832760 ) ) ;
#2018=CARTESIAN_POINT ( 'NONE',  ( 35.22227017426903473, -20.71851614966110233, -20.19360243392694088 ) ) ;
#2021=CARTESIAN_POINT ( 'NONE',  ( 12.75768479220908169, 7.626547943635540783, -14.92479568483475028 ) ) ;
#2028=CARTESIAN_POINT ( 'NONE',  ( 15.98547205987755149, 10.89358938796158149, -13.63095616771664709 ) ) ;
#2030=CARTESIAN_POINT ( 'NONE',  ( 32.83462640711407232, -10.30445905196369516, -16.67331141712644538 ) ) ;
#2032=CARTESIAN_POINT ( 'NONE',  ( 24.68825858685077179, -9.385095155728059524, -16.92495907518576104 ) ) ;
#2038=CARTESIAN_POINT ( 'NONE',  ( 27.15223745481332784, -12.21752729395051063, -18.24437427626675046 ) ) ;
#2039=CARTESIAN_POINT ( 'NONE',  ( 24.41106252871404436, -7.915231898853421377, -13.94454578273958667 ) ) ;
#2047=CARTESIAN_POINT ( 'NONE',  ( 12.48799528366842360, 8.565546312597838607, -15.13973160209665991 ) ) ;
#2048=CARTESIAN_POINT ( 'NONE',  ( 27.61484239614359737, -11.78684095324212855, -18.66559939683001446 ) ) ;
#2052=CARTESIAN_POINT ( 'NONE',  ( 9.641350810849047548, 17.66889113945805789, -17.93331994345748370 ) ) ;
#2053=CARTESIAN_POINT ( 'NONE',  ( 27.56197131007709444, -12.41890123633259435, -14.84244373703855935 ) ) ;
#2057=CARTESIAN_POINT ( 'NONE',  ( 23.56138260001205964, -6.829566487537672259, -18.05074380722902916 ) ) ;
#2061=CARTESIAN_POINT ( 'NONE',  ( 11.05541531668977662, 17.68942339022145305, -17.92981046679734547 ) ) ;
#2062=CARTESIAN_POINT ( 'NONE',  ( 35.54859215833182873, -22.18450796649496226, -18.40462262104107083 ) ) ;
#2065=CARTESIAN_POINT ( 'NONE',  ( 24.14158683625483803, -3.940216521628096658, -13.50644477367014673 ) ) ;
#2068=CARTESIAN_POINT ( 'NONE',  ( 21.79248024726475563, -3.676524810334697246, -15.28166220873658077 ) ) ;
#2073=CARTESIAN_POINT ( 'NONE',  ( 16.38240814442996651, 6.370603895193741373, -13.89573738210111919 ) ) ;
#2075=CARTESIAN_POINT ( 'NONE',  ( 30.15014520769674533, -9.019674524353797906, -15.19912247041013842 ) ) ;
#2086=CARTESIAN_POINT ( 'NONE',  ( 23.39714218815755231, -8.028440028060597200, -17.83143846932372512 ) ) ;
#2087=CARTESIAN_POINT ( 'NONE',  ( 21.65198393244800812, 4.573788442230395823, -17.29480057625502454 ) ) ;
#2088=CARTESIAN_POINT ( 'NONE',  ( 33.72790161547175103, -10.96501189107364738, -20.51660325596433765 ) ) ;
#2091=CARTESIAN_POINT ( 'NONE',  ( 12.44984726620633353, 8.550925603015029353, -15.16996558791898231 ) ) ;
#2094=CARTESIAN_POINT ( 'NONE',  ( 9.667840685194843076, 16.22750421244806063, -17.88508776754438401 ) ) ;
#2098=CARTESIAN_POINT ( 'NONE',  ( 12.23783994716398560, 8.515526397163364791, -15.33449341356891615 ) ) ;
#2106=CARTESIAN_POINT ( 'NONE',  ( 10.34450975306715570, 10.53135794231081057, -16.54525784588868120 ) ) ;
#2107=CARTESIAN_POINT ( 'NONE',  ( 31.15806985163746390, -10.82494328065958911, -14.16671120874331358 ) ) ;
#2110=CARTESIAN_POINT ( 'NONE',  ( 18.14419664895403272, 7.915595134365798202, -13.41836860846829538 ) ) ;
#2112=CARTESIAN_POINT ( 'NONE',  ( 14.70507544977879100, 5.024503852999842479, -17.88552553980999704 ) ) ;
#2116=CARTESIAN_POINT ( 'NONE',  ( 22.15378238435969394, -4.028439702987021143, -12.64872919198682943 ) ) ;
#2124=CARTESIAN_POINT ( 'NONE',  ( 13.66828981435543788, 8.811555337407297017, -15.47779131845254952 ) ) ;
#2125=CARTESIAN_POINT ( 'NONE',  ( 35.05137900175546406, -18.95079263513605028, -19.16533087415493952 ) ) ;
#2126=CARTESIAN_POINT ( 'NONE',  ( 10.70135522441200671, 8.911701773272509897, -16.39640207298747754 ) ) ;
#2129=CARTESIAN_POINT ( 'NONE',  ( 28.15048769591263067, -5.842385520647848551, -16.89978903947823241 ) ) ;
#2131=CARTESIAN_POINT ( 'NONE',  ( 10.47300640208398370, 16.44766825625507778, -17.33439677017039671 ) ) ;
#2136=CARTESIAN_POINT ( 'NONE',  ( 12.55500454421123457, 8.595009676161804890, -15.08633542003848049 ) ) ;
#2140=CARTESIAN_POINT ( 'NONE',  ( 9.667821753224751902, 16.22759103687616999, -17.88509611560606061 ) ) ;
#2142=CARTESIAN_POINT ( 'NONE',  ( 24.26229878782818261, 2.002655289519151172, -16.31248287692968546 ) ) ;
#2143=CARTESIAN_POINT ( 'NONE',  ( 23.66883837772530441, 2.046813550970532969, -14.77838854720118000 ) ) ;
#2146=CARTESIAN_POINT ( 'NONE',  ( 17.20140313730510684, 4.016069822000726042, -19.84498366692964666 ) ) ;
#2150=CARTESIAN_POINT ( 'NONE',  ( 17.72480397827495224, 1.356124466512965476, -19.40231245121514903 ) ) ;
#2154=CARTESIAN_POINT ( 'NONE',  ( 10.35865005771744762, 16.97212102856341787, -17.91352035578586310 ) ) ;
#2160=CARTESIAN_POINT ( 'NONE',  ( 17.29421355564066332, 9.360779442694735053, -19.18964209290773937 ) ) ;
#2161=CARTESIAN_POINT ( 'NONE',  ( 11.25757798850943381, 16.76227960750979307, -16.79548539596511247 ) ) ;
#2165=CARTESIAN_POINT ( 'NONE',  ( 9.893572868141015775, 16.51216863388285461, -16.51808063826580408 ) ) ;
#2167=CARTESIAN_POINT ( 'NONE',  ( 9.641350810849047548, 17.66889113945805789, -21.33333333332589277 ) ) ;
#2173=CARTESIAN_POINT ( 'NONE',  ( 10.46817501828509123, 16.46982559821503145, -17.33665662920367723 ) ) ;
#2174=CARTESIAN_POINT ( 'NONE',  ( 33.97319001242765779, -11.13623552147873141, -19.50814438409551954 ) ) ;
#2175=CARTESIAN_POINT ( 'NONE',  ( 27.31974442496251143, -5.660127319198639206, -14.41990313654811651 ) ) ;
#2186=CARTESIAN_POINT ( 'NONE',  ( 15.30293317557315902, 5.113330479851449617, -15.60941525921096051 ) ) ;
#2187=CARTESIAN_POINT ( 'NONE',  ( 25.07632161252335123, -1.101686516974712315, -19.85338880782979132 ) ) ;
#2195=CARTESIAN_POINT ( 'NONE',  ( 10.72335299953182286, 16.61944783517715862, -15.95314022879208693 ) ) ;
#2200=CARTESIAN_POINT ( 'NONE',  ( 9.919231947839115549, 16.39449282361540483, -16.50339887433786501 ) ) ;
#2201=CARTESIAN_POINT ( 'NONE',  ( 17.86202776125589153, 5.750484210099715554, -19.07881598002096268 ) ) ;
#2204=CARTESIAN_POINT ( 'NONE',  ( 25.07290406138036687, -9.006318079059196791, -17.79994936451110732 ) ) ;
#2208=CARTESIAN_POINT ( 'NONE',  ( 12.38124869470495781, 9.576253617860157163, -15.22482189909362660 ) ) ;
#2210=CARTESIAN_POINT ( 'NONE',  ( 32.25667210025905263, -11.64161264113965011, -15.27003429613047025 ) ) ;
#2216=CARTESIAN_POINT ( 'NONE',  ( 24.19805618307960060, -0.7920880973371497991, -16.79971198345035432 ) ) ;
#2222=CARTESIAN_POINT ( 'NONE',  ( 20.55949567978923298, 1.660703385868308235, -14.27713627412184039 ) ) ;
#2223=CARTESIAN_POINT ( 'NONE',  ( 27.32970014129078962, -12.32490512882196754, -16.69500413328365696 ) ) ;
#2231=CARTESIAN_POINT ( 'NONE',  ( 9.917205744531459644, 16.40378525026516243, -16.50423678068149869 ) ) ;
#2232=CARTESIAN_POINT ( 'NONE',  ( 20.87485249991972580, -5.094386175754089585, -18.86169636093909219 ) ) ;
#2233=CARTESIAN_POINT ( 'NONE',  ( 18.32179412900206827, 3.681508181950223335, -14.15692665485406643 ) ) ;
#2236=CARTESIAN_POINT ( 'NONE',  ( 33.45813146310553066, -13.79317541067231723, -20.76837346131055639 ) ) ;
#2238=CARTESIAN_POINT ( 'NONE',  ( 12.39803340617553928, 8.535179507765855433, -15.21071672276548625 ) ) ;
#2241=CARTESIAN_POINT ( 'NONE',  ( 14.34656430690936624, 9.113120221615268690, -15.03016663717492563 ) ) ;
#2244=CARTESIAN_POINT ( 'NONE',  ( 14.38576730248667701, 9.404056492746565965, -13.62718518646353161 ) ) ;
#2250=CARTESIAN_POINT ( 'NONE',  ( 16.75072914628186282, 8.771658487634226731, -19.67538163746542779 ) ) ;
#2253=CARTESIAN_POINT ( 'NONE',  ( 9.109746387114286748, 16.19414013429083710, -17.05597298747021640 ) ) ;
#2254=CARTESIAN_POINT ( 'NONE',  ( 33.35113679096266992, -13.31250502539155534, -20.73603153870848104 ) ) ;
#2255=CARTESIAN_POINT ( 'NONE',  ( 16.82931527361030533, 7.354042003703605168, -13.11858969620360504 ) ) ;
#2257=CARTESIAN_POINT ( 'NONE',  ( 27.62103240953636174, -12.62788667074165794, -13.46147607715242245 ) ) ;
#2260=CARTESIAN_POINT ( 'NONE',  ( 20.29686952095399377, -4.285349973794369660, -18.75376381207850329 ) ) ;
#2271=CARTESIAN_POINT ( 'NONE',  ( 36.44623027834506956, -20.72465026231317253, -19.27049969669971929 ) ) ;
#2273=CARTESIAN_POINT ( 'NONE',  ( 10.63628302936969483, 9.193248504745362482, -16.42459933240677827 ) ) ;
#2279=CARTESIAN_POINT ( 'NONE',  ( 10.63408956504272140, 15.70892033759881734, -17.26778321585235787 ) ) ;
#2287=CARTESIAN_POINT ( 'NONE',  ( 9.732710754582456048, 15.93000180522596665, -17.85826136589200175 ) ) ;
#2288=CARTESIAN_POINT ( 'NONE',  ( 22.68697051328012293, -3.855329871767240402, -18.23939831819710733 ) ) ;
#2289=CARTESIAN_POINT ( 'NONE',  ( 23.24226111988221888, -3.343277867803439829, -18.62279721135557509 ) ) ;
#2290=CARTESIAN_POINT ( 'NONE',  ( 21.63689124574611711, 4.661388338709377521, -16.95871344450652174 ) ) ;
#2296=CARTESIAN_POINT ( 'NONE',  ( 27.78884322698630882, -6.380937659459246625, -17.89340433249687834 ) ) ;
#2304=CARTESIAN_POINT ( 'NONE',  ( 10.46247360472336041, 16.49597300757040230, -17.34042816522791952 ) ) ;
#2309=CARTESIAN_POINT ( 'NONE',  ( 10.96464236563772943, 10.28020640217055259, -17.34881430896752619 ) ) ;
#2315=CARTESIAN_POINT ( 'NONE',  ( 20.39549844898813191, -2.061726703908969505, -13.85117726305786512 ) ) ;
#2316=CARTESIAN_POINT ( 'NONE',  ( 11.08268301555968094, 17.56437024738003316, -17.37355016474266733 ) ) ;
#2317=CARTESIAN_POINT ( 'NONE',  ( 33.47012763672258728, -12.84706786418751534, -19.72967806864707541 ) ) ;
#2321=CARTESIAN_POINT ( 'NONE',  ( 9.641350810849047548, 17.66889113945805789, -17.92015940598198753 ) ) ;
#2323=CARTESIAN_POINT ( 'NONE',  ( 9.641350810849047548, 17.66889113945805789, -17.92454625180715766 ) ) ;
#2330=CARTESIAN_POINT ( 'NONE',  ( 10.47204342302745417, 16.45208460095963687, -17.33479495221483901 ) ) ;
#2331=CARTESIAN_POINT ( 'NONE',  ( 34.15817405333866219, -12.44562566045073204, -20.90971876709214783 ) ) ;
#2332=CARTESIAN_POINT ( 'NONE',  ( 25.24878800877705487, -9.370948223588685622, -14.18615728435988288 ) ) ;
#2337=CARTESIAN_POINT ( 'NONE',  ( 19.14730738223925854, 6.711798791111892371, -15.43835307388804701 ) ) ;
#2338=CARTESIAN_POINT ( 'NONE',  ( 26.67280208910032258, -8.806626608708889137, -18.22016464309510653 ) ) ;
#2350=CARTESIAN_POINT ( 'NONE',  ( 10.72031594518761466, 16.63337615353409760, -15.95439753950889106 ) ) ;
#2356=CARTESIAN_POINT ( 'NONE',  ( 10.43540724046455992, 14.02724713458965233, -16.28994223329847202 ) ) ;
#2358=CARTESIAN_POINT ( 'NONE',  ( 16.45434084995319424, 8.990804261541395448, -14.78801614696073408 ) ) ;
#2361=CARTESIAN_POINT ( 'NONE',  ( 25.97256211245905533, -8.171536508395311316, -18.54953510021574559 ) ) ;
#2365=CARTESIAN_POINT ( 'NONE',  ( 11.40579136381300174, 16.08255417555669453, -16.73093107180499928 ) ) ;
#2368=CARTESIAN_POINT ( 'NONE',  ( 32.61797162530606187, -11.69648652134232414, -16.29118568026193614 ) ) ;
#2370=CARTESIAN_POINT ( 'NONE',  ( 28.52362724998032917, -7.841767518281756111, -12.14325827080317666 ) ) ;
#2373=CARTESIAN_POINT ( 'NONE',  ( 18.54205238286641588, 5.219565156008159512, -20.23764637224795848 ) ) ;
#2374=CARTESIAN_POINT ( 'NONE',  ( 29.75294099516071711, -10.02427176990993196, -17.65830536592410738 ) ) ;
#2385=CARTESIAN_POINT ( 'NONE',  ( 9.916824447075894611, 16.40553392900050156, -16.50439446175997205 ) ) ;
#2388=CARTESIAN_POINT ( 'NONE',  ( 27.54556670433429488, -3.970347839692917713, -18.20727554117155123 ) ) ;
#2389=CARTESIAN_POINT ( 'NONE',  ( 22.34648740292275093, -2.602002351270185532, -19.46322174391540116 ) ) ;
#2390=CARTESIAN_POINT ( 'NONE',  ( 32.03687507811291368, -10.31171301082699543, -18.65038288416666390 ) ) ;
#2395=CARTESIAN_POINT ( 'NONE',  ( 14.33367420948735393, 6.252843122977492563, -16.41390433006782956 ) ) ;
#2398=CARTESIAN_POINT ( 'NONE',  ( 10.73095126193553028, 16.58460123524055874, -15.94999808000346242 ) ) ;
#2402=CARTESIAN_POINT ( 'NONE',  ( 18.88762249820254624, 5.002188274287570735, -13.90571046850145542 ) ) ;
#2404=CARTESIAN_POINT ( 'NONE',  ( 13.70585326225313771, 5.953887885347688425, -14.73188983601744617 ) ) ;
#2406=CARTESIAN_POINT ( 'NONE',  ( 32.74140904187309786, -11.17293925747269867, -20.20304766317806866 ) ) ;
#2408=CARTESIAN_POINT ( 'NONE',  ( 23.40821609032294859, 1.473297984346819245, -16.37969033120859308 ) ) ;
#2410=CARTESIAN_POINT ( 'NONE',  ( 15.92010713857317938, 6.231155140105813395, -20.15531274222559333 ) ) ;
#2412=CARTESIAN_POINT ( 'NONE',  ( 29.77493782482978091, -9.049732786019394126, -14.43420072379011643 ) ) ;
#2422=CARTESIAN_POINT ( 'NONE',  ( 36.54645402898028550, -21.17490248391822050, -18.49223762587710951 ) ) ;
#2424=CARTESIAN_POINT ( 'NONE',  ( 12.75441094417786658, 7.625102360211175601, -14.92740490885063309 ) ) ;
#2427=CARTESIAN_POINT ( 'NONE',  ( 10.35887147716723611, 16.97110557074245563, -17.87975733919941845 ) ) ;
#2433=VERTEX_POINT ( 'NONE', #6457 ) ;
#2438=CARTESIAN_POINT ( 'NONE',  ( 10.31625730718771017, 13.25378293009361563, -17.61694433892753153 ) ) ;
#2439=CARTESIAN_POINT ( 'NONE',  ( 24.47745745569867637, -8.908941985067972524, -13.71056886683244258 ) ) ;
#2440=CARTESIAN_POINT ( 'NONE',  ( 25.07020310977553024, -1.264175079641418398, -16.65545549153034699 ) ) ;
#2442=CARTESIAN_POINT ( 'NONE',  ( 19.82332968365342296, 2.432204761014481242, -19.52120720162773537 ) ) ;
#2450=CARTESIAN_POINT ( 'NONE',  ( 23.11440248821028831, -7.346120041196752659, -16.32852059634029018 ) ) ;
#2458=CARTESIAN_POINT ( 'NONE',  ( 10.35900481074863322, 16.97049408594186914, -17.87076805301065363 ) ) ;
#2460=CARTESIAN_POINT ( 'NONE',  ( 32.67186286342521839, -11.06527230177895227, -18.43913201350460440 ) ) ;
#2462=CARTESIAN_POINT ( 'NONE',  ( 13.32639783386816212, 7.603689066773378968, -15.75018979827038912 ) ) ;
#2465=CARTESIAN_POINT ( 'NONE',  ( 17.55424633453837302, 0.6138019359854992585, -14.89346452969079060 ) ) ;
#2466=CARTESIAN_POINT ( 'NONE',  ( 11.27518382607279968, 16.68153699222178687, -16.78494985227356295 ) ) ;
#2472=CARTESIAN_POINT ( 'NONE',  ( 9.916953853453376766, 16.40494045485788632, -16.50434094533541085 ) ) ;
#2475=CARTESIAN_POINT ( 'NONE',  ( 9.915973561396301150, 16.40943619918981256, -16.50475030878699556 ) ) ;
#2481=CARTESIAN_POINT ( 'NONE',  ( 10.51251736658329961, 16.26646593658467310, -17.31805759646961462 ) ) ;
#2483=CARTESIAN_POINT ( 'NONE',  ( 32.62421882425100961, -9.622687980317111922, -18.08031881573170097 ) ) ;
#2484=CARTESIAN_POINT ( 'NONE',  ( 28.67486520862709654, -7.888541471525570614, -13.83454100519475105 ) ) ;
#2488=CARTESIAN_POINT ( 'NONE',  ( 33.68917633736438688, -10.64779379647620949, -18.96437360758372748 ) ) ;
#2493=CARTESIAN_POINT ( 'NONE',  ( 17.64917075666736679, 6.165203978315560995, -14.56523922633501655 ) ) ;
#2494=AXIS2_PLACEMENT_3D ( 'NONE', #19113, #21556, #22010 ) ;
#2496=CARTESIAN_POINT ( 'NONE',  ( 28.11208967899271371, -8.897075463600188527, -14.13618326516971990 ) ) ;
#2505=CARTESIAN_POINT ( 'NONE',  ( 10.33841720888800531, 18.38481243897025053, -17.83974501271621449 ) ) ;
#2511=CARTESIAN_POINT ( 'NONE',  ( 9.917015787971365626, 16.40465641526357743, -16.50431533440121257 ) ) ;
#2513=CARTESIAN_POINT ( 'NONE',  ( 15.27107031639597423, 6.121678041989828678, -18.36639460046777828 ) ) ;
#2516=CARTESIAN_POINT ( 'NONE',  ( 27.83100014064079275, -5.545984359997562230, -15.13782040115233052 ) ) ;
#2519=CARTESIAN_POINT ( 'NONE',  ( 11.27518382607279968, 16.68153699222178687, -16.78494985227356295 ) ) ;
#2521=CARTESIAN_POINT ( 'NONE',  ( 33.66044826391103584, -12.70207762650279015, -18.74488588032081893 ) ) ;
#2522=CARTESIAN_POINT ( 'NONE',  ( 17.12833724908345800, 9.171387755021909172, -19.38714867094073213 ) ) ;
#2525=CARTESIAN_POINT ( 'NONE',  ( 25.29949251596307036, -5.094144391296384633, -13.01082609127739076 ) ) ;
#2528=CARTESIAN_POINT ( 'NONE',  ( 20.41927524488895429, 4.553956414902842198, -14.69105443414393264 ) ) ;
#2529=CARTESIAN_POINT ( 'NONE',  ( 18.11961939296043056, 8.971021047410516758, -18.23824686698257125 ) ) ;
#2541=CARTESIAN_POINT ( 'NONE',  ( 9.917332382238186028, 16.40320447359955125, -16.50418441153501448 ) ) ;
#2542=CARTESIAN_POINT ( 'NONE',  ( 20.32939975687981615, -5.674178230592766603, -17.16996371750385109 ) ) ;
#2543=CARTESIAN_POINT ( 'NONE',  ( 21.84445237452005628, 0.7298858868756038509, -19.18266460542251295 ) ) ;
#2544=CARTESIAN_POINT ( 'NONE',  ( 30.54120030308987666, -10.08143909378498293, -14.42492330020037272 ) ) ;
#2547=CARTESIAN_POINT ( 'NONE',  ( 13.04501788334644630, 8.811555337407297017, -14.69578613943112799 ) ) ;
#2550=CARTESIAN_POINT ( 'NONE',  ( 17.08157517049449581, 7.460725202527481947, -14.57009041681831896 ) ) ;
#2553=CARTESIAN_POINT ( 'NONE',  ( 10.33811693838771717, 18.38618951776012267, -17.91752729848688830 ) ) ;
#2558=CARTESIAN_POINT ( 'NONE',  ( 14.17177033308128031, 6.273687421093853800, -17.36430109743762173 ) ) ;
#2559=CARTESIAN_POINT ( 'NONE',  ( 25.32913879335529472, -12.33208189297920221, -17.76794973357399243 ) ) ;
#2561=CARTESIAN_POINT ( 'NONE',  ( 35.46335518829674527, -22.80158341140986167, -19.83799967047498924 ) ) ;
#2562=CARTESIAN_POINT ( 'NONE',  ( 21.26848706961299129, -1.060808783303755387, -18.71231287479539063 ) ) ;
#2563=CARTESIAN_POINT ( 'NONE',  ( 19.79992434292498515, 0.1278105412470878222, -19.37491769885296122 ) ) ;
#2567=CARTESIAN_POINT ( 'NONE',  ( 29.18140637672732396, -9.206484972055292815, -13.74645275385354815 ) ) ;
#2574=CARTESIAN_POINT ( 'NONE',  ( 36.54859390953724585, -21.18451583373416014, -17.99055332684694974 ) ) ;
#2575=CARTESIAN_POINT ( 'NONE',  ( 13.02821298986966703, 7.746099194123166498, -14.70917993614958519 ) ) ;
#2580=CARTESIAN_POINT ( 'NONE',  ( 10.47705880869930084, 16.42908340295556258, -17.33272095748315422 ) ) ;
#2589=CARTESIAN_POINT ( 'NONE',  ( 11.06190012440529102, 9.834169922982590961, -17.30859480447365328 ) ) ;
#2590=CARTESIAN_POINT ( 'NONE',  ( 23.04322939705109974, -6.346999004730295546, -16.23111451206203881 ) ) ;
#2591=CARTESIAN_POINT ( 'NONE',  ( 19.92565466131104301, 6.686648131885553958, -19.16379146452587179 ) ) ;
#2597=CARTESIAN_POINT ( 'NONE',  ( 25.71553203045151292, -8.406338935355361031, -18.42709291467145150 ) ) ;
#2604=CARTESIAN_POINT ( 'NONE',  ( 10.50441255335269020, 16.30363564318377811, -17.32140922184415288 ) ) ;
#2606=CARTESIAN_POINT ( 'NONE',  ( 33.17819505895439391, -11.78846528140086924, -19.49437495119144259 ) ) ;
#2608=CARTESIAN_POINT ( 'NONE',  ( 8.944584683310379702, 16.95159276115599667, -17.92981046679734547 ) ) ;
#2611=CARTESIAN_POINT ( 'NONE',  ( 21.41025690189560748, 5.821651141963339882, -16.00656683556521998 ) ) ;
#2612=CARTESIAN_POINT ( 'NONE',  ( 11.26682494837019277, 16.71987187087499294, -16.78921452078379062 ) ) ;
#2617=CARTESIAN_POINT ( 'NONE',  ( 9.745779815811758340, 17.18996641109745482, -16.82979807527155458 ) ) ;
#2619=CARTESIAN_POINT ( 'NONE',  ( 9.916336358462064737, 16.40777236560037622, -16.50459729666445696 ) ) ;
#2625=CARTESIAN_POINT ( 'NONE',  ( 10.35867142355733783, 16.97202304209818990, -17.90451223021000260 ) ) ;
#2627=CARTESIAN_POINT ( 'NONE',  ( 36.30362226317071617, -21.08398799169651738, -20.22680612736627026 ) ) ;
#2628=CARTESIAN_POINT ( 'NONE',  ( 15.57351372253994271, 10.71565324155555388, -15.28765949597478624 ) ) ;
#2629=CARTESIAN_POINT ( 'NONE',  ( 26.58455406938135468, -5.910422570377376950, -13.89432871846328688 ) ) ;
#2633=CARTESIAN_POINT ( 'NONE',  ( 30.50415327504139285, -11.36213899161910135, -13.19862950667920565 ) ) ;
#2634=CARTESIAN_POINT ( 'NONE',  ( 16.01392728624657025, 9.853228751548474662, -15.03783782146776105 ) ) ;
#2642=CARTESIAN_POINT ( 'NONE',  ( 10.33816386007038268, 18.38597432894226458, -17.88535571907410571 ) ) ;
#2648=CARTESIAN_POINT ( 'NONE',  ( 11.47269659055779378, 9.270105954394804115, -15.86098659800193644 ) ) ;
#2650=CARTESIAN_POINT ( 'NONE',  ( 9.668885350391278166, 16.22271324469333109, -17.88465541571617834 ) ) ;
#2651=CARTESIAN_POINT ( 'NONE',  ( 18.87764716858279002, 3.471780965079254599, -19.68009874701989048 ) ) ;
#2654=CARTESIAN_POINT ( 'NONE',  ( 25.24878800877705487, -9.370948223588685622, -14.18615728435988288 ) ) ;
#2656=CARTESIAN_POINT ( 'NONE',  ( 11.05818223728759264, 17.67673393965927175, -17.74095938596937572 ) ) ;
#2658=CARTESIAN_POINT ( 'NONE',  ( 35.54859390953724585, -21.18451583373416014, -18.06010107863414405 ) ) ;
#2661=CARTESIAN_POINT ( 'NONE',  ( 22.52525573827019301, -5.869110285238294367, -18.12586539066504798 ) ) ;
#2664=CARTESIAN_POINT ( 'NONE',  ( 21.50147616854745891, 4.214167280306792662, -18.19698480873994839 ) ) ;
#2665=CARTESIAN_POINT ( 'NONE',  ( 17.93652952100233833, 4.843921488302829204, -14.86957952233187896 ) ) ;
#2673=CARTESIAN_POINT ( 'NONE',  ( 9.641351021852148762, 17.66889017177091503, -17.91406276888456617 ) ) ;
#2674=CARTESIAN_POINT ( 'NONE',  ( 21.89112544314524200, -5.209854132323804343, -13.34451667507982364 ) ) ;
#2675=CARTESIAN_POINT ( 'NONE',  ( 19.87821071931953298, -1.530402839103173651, -15.12151443550766494 ) ) ;
#2677=CARTESIAN_POINT ( 'NONE',  ( 31.74553205326546390, -10.26435202779689604, -17.82876124730869805 ) ) ;
#2680=CARTESIAN_POINT ( 'NONE',  ( 12.63667343406881294, 8.631100619704961119, -15.02124387326777111 ) ) ;
#2685=EDGE_CURVE ( 'NONE', #2433, #14962, #875, .T. ) ;
#2689=CARTESIAN_POINT ( 'NONE',  ( 10.33811693838771717, 18.38618951776012267, -17.91664992932185996 ) ) ;
#2693=CARTESIAN_POINT ( 'NONE',  ( 21.04385110482095200, 5.766204710259658306, -15.30406332615466347 ) ) ;
#2695=CARTESIAN_POINT ( 'NONE',  ( 25.72097854023329688, -11.95459465090917917, -18.51508836554082293 ) ) ;
#2697=CARTESIAN_POINT ( 'NONE',  ( 35.54859215833182873, -22.18450796649496226, -18.40462262104107083 ) ) ;
#2698=CARTESIAN_POINT ( 'NONE',  ( 23.33644427035094537, 1.513498076802863190, -16.07814869553001103 ) ) ;
#2699=CARTESIAN_POINT ( 'NONE',  ( 19.19659130220728116, 4.347481709847851761, -15.16398724834160916 ) ) ;
#2701=CARTESIAN_POINT ( 'NONE',  ( 28.07139740185986199, -11.61962552671339388, -17.78409693965565452 ) ) ;
#2710=CARTESIAN_POINT ( 'NONE',  ( 36.54859286093297754, -21.18451112290966165, -18.39168789611893118 ) ) ;
#2711=CARTESIAN_POINT ( 'NONE',  ( 12.76449053303042902, 7.629555522264023892, -14.91937138927071160 ) ) ;
#2718=CARTESIAN_POINT ( 'NONE',  ( 11.96327893486549776, 9.613088455355432771, -16.71811665443363992 ) ) ;
#2731=CARTESIAN_POINT ( 'NONE',  ( 9.671924655352764688, 16.20877460471870535, -17.88339855620073848 ) ) ;
#2733=CARTESIAN_POINT ( 'NONE',  ( 27.30941123812745275, -4.721684434479056947, -15.35818731037458029 ) ) ;
#2734=CARTESIAN_POINT ( 'NONE',  ( 23.93603600111211804, 0.1510904554606163908, -14.93755387302875448 ) ) ;
#2738=CARTESIAN_POINT ( 'NONE',  ( 25.04992766293576878, -3.547109489677171101, -13.67097983722207033 ) ) ;
#2749=CARTESIAN_POINT ( 'NONE',  ( 12.01190781424926435, 9.390070215761314287, -16.69800690218674788 ) ) ;
#2751=CARTESIAN_POINT ( 'NONE',  ( 32.48283477683061449, -11.02614750807341260, -17.91093295056291979 ) ) ;
#2753=CARTESIAN_POINT ( 'NONE',  ( 8.944584683310379702, 16.95159276115599667, -17.98596209335946128 ) ) ;
#2757=CARTESIAN_POINT ( 'NONE',  ( 18.88762249820254624, 5.002188274287570735, -13.90571046850145542 ) ) ;
#2759=CARTESIAN_POINT ( 'NONE',  ( 12.84002880955021197, 9.524163120117652426, -16.13635871874149430 ) ) ;
#2765=CARTESIAN_POINT ( 'NONE',  ( 9.912057827679275235, 16.42739425315605928, -16.50652470164456531 ) ) ;
#2768=CARTESIAN_POINT ( 'NONE',  ( 9.921764701973689426, 16.38287729030320250, -16.50235149140834778 ) ) ;
#2773=CARTESIAN_POINT ( 'NONE',  ( 10.35865057885519214, 16.97211863855931924, -17.91295731025335414 ) ) ;
#2776=CARTESIAN_POINT ( 'NONE',  ( 36.54859390953724585, -22.18451583373416014, -16.94733705004010460 ) ) ;
#2777=CARTESIAN_POINT ( 'NONE',  ( 26.32595758385100382, -12.12905223104374386, -14.21117607008287642 ) ) ;
#2778=CARTESIAN_POINT ( 'NONE',  ( 14.76280285026742867, 7.190900411307756812, -14.35234371774122408 ) ) ;
#2781=CARTESIAN_POINT ( 'NONE',  ( 33.40535544545146251, -10.40465400369240356, -18.27852168438239389 ) ) ;
#2783=CARTESIAN_POINT ( 'NONE',  ( 15.50826552155665183, 8.864470348925614474, -13.64319937614855149 ) ) ;
#2784=CARTESIAN_POINT ( 'NONE',  ( 25.57659404178318141, -9.842204813007603192, -16.83936284125123706 ) ) ;
#2797=CARTESIAN_POINT ( 'NONE',  ( 10.72094366404044408, 16.63049735485946101, -15.95413657539408980 ) ) ;
#2802=CARTESIAN_POINT ( 'NONE',  ( 9.915248083523094280, 16.41276333319327918, -16.50506225043874409 ) ) ;
#2804=CARTESIAN_POINT ( 'NONE',  ( 9.666286124033039329, 16.23463362809610899, -17.88661257689534878 ) ) ;
#2805=CARTESIAN_POINT ( 'NONE',  ( 18.15277384750198308, 2.816914934748806054, -19.48283598520044180 ) ) ;
#2807=CARTESIAN_POINT ( 'NONE',  ( 29.62588713853392264, -10.65184931322849060, -12.76488833982454629 ) ) ;
#2810=CARTESIAN_POINT ( 'NONE',  ( 11.27425361364269563, 16.68580306500076915, -16.78535843524344173 ) ) ;
#2812=CARTESIAN_POINT ( 'NONE',  ( 33.71394559998177698, -12.94241281914233355, -18.76105684162217457 ) ) ;
#2813=CARTESIAN_POINT ( 'NONE',  ( 20.24985932600369409, 3.694099309552050237, -20.13309853732883781 ) ) ;
#2816=CARTESIAN_POINT ( 'NONE',  ( 8.952973202525470242, 16.91312194274802749, -17.65238394630757313 ) ) ;
#2817=CARTESIAN_POINT ( 'NONE',  ( 30.91631662189391250, -8.208988707411489116, -18.28093047724294351 ) ) ;
#2820=CARTESIAN_POINT ( 'NONE',  ( 18.63710449947919301, 3.826706299981984305, -14.11708861520305192 ) ) ;
#2822=CARTESIAN_POINT ( 'NONE',  ( 15.60359850163179551, 6.442352727238609411, -18.97839103356167101 ) ) ;
#2833=CARTESIAN_POINT ( 'NONE',  ( 9.641350810849047548, 17.66889113945805789, -17.91664992932186351 ) ) ;
#2834=CARTESIAN_POINT ( 'NONE',  ( 25.27624414898354388, -7.528478751523516088, -13.47981680254768655 ) ) ;
#2835=CARTESIAN_POINT ( 'NONE',  ( 24.59961324288297391, 0.2024632608770970121, -16.27125138369466484 ) ) ;
#2836=CARTESIAN_POINT ( 'NONE',  ( 31.02293300316137348, -10.15460426738793664, -15.78645847904462052 ) ) ;
#2843=CARTESIAN_POINT ( 'NONE',  ( 14.18486973814142793, 6.324582201221724098, -17.68508340245422872 ) ) ;
#2846=CARTESIAN_POINT ( 'NONE',  ( 10.72061166913284325, 16.63201992582523658, -15.95427402900266856 ) ) ;
#2850=CARTESIAN_POINT ( 'NONE',  ( 15.22033579473957410, 7.355362781181614018, -19.64495939069069763 ) ) ;
#2851=CARTESIAN_POINT ( 'NONE',  ( 26.55477173981947914, -11.17418396328012342, -19.38009549175560053 ) ) ;
#2853=CARTESIAN_POINT ( 'NONE',  ( 32.54305136433941215, -11.03529315477374517, -18.08112484791816499 ) ) ;
#2854=CARTESIAN_POINT ( 'NONE',  ( 23.72730982194951466, -1.509008702439352589, -18.09242500859757996 ) ) ;
#2855=CARTESIAN_POINT ( 'NONE',  ( 18.47998620531167902, -1.197692507188573785, -16.87724725366775402 ) ) ;
#2857=CARTESIAN_POINT ( 'NONE',  ( 29.53935142057454755, -5.962610374456907003, -16.12847026952743690 ) ) ;
#2870=CARTESIAN_POINT ( 'NONE',  ( 36.54859390954302967, -21.18451583373416014, -15.55638201429745848 ) ) ;
#2871=CARTESIAN_POINT ( 'NONE',  ( 9.649959050778257108, 17.62941265384766254, -17.56860460898032628 ) ) ;
#2874=CARTESIAN_POINT ( 'NONE',  ( 12.03006260835556951, 9.306948544855226046, -16.69048869075990638 ) ) ;
#2886=CARTESIAN_POINT ( 'NONE',  ( 13.37720302390605553, 7.624891072754538257, -15.70979247928349132 ) ) ;
#2889=CARTESIAN_POINT ( 'NONE',  ( 25.37470919123784086, -4.075530507763302168, -17.99687124876041011 ) ) ;
#2891=CARTESIAN_POINT ( 'NONE',  ( 21.59786356094703308, -0.7637721020719707710, -13.97513905925265298 ) ) ;
#2895=EDGE_CURVE ( 'NONE', #8851, #3493, #22818, .T. ) ;
#2907=CARTESIAN_POINT ( 'NONE',  ( 12.00785540763395254, 9.408655069060824161, -16.69968271487400813 ) ) ;
#2909=CARTESIAN_POINT ( 'NONE',  ( 32.12153525177792091, -10.97127362787143312, -16.88978156643115724 ) ) ;
#2911=CARTESIAN_POINT ( 'NONE',  ( 8.944667066222118379, 16.95121494262130213, -17.88907156968992496 ) ) ;
#2913=CARTESIAN_POINT ( 'NONE',  ( 19.40121574091639189, 1.432572567346982240, -13.43353846741550406 ) ) ;
#2914=CARTESIAN_POINT ( 'NONE',  ( 12.86106464449595777, 9.514195438118767001, -16.12106201145810047 ) ) ;
#2917=CARTESIAN_POINT ( 'NONE',  ( 10.43540724046455992, 14.02724713458965233, -16.28994223329847202 ) ) ;
#2919=CARTESIAN_POINT ( 'NONE',  ( 9.916637298967875935, 16.40639221407973380, -16.50447193873893781 ) ) ;
#2924=CARTESIAN_POINT ( 'NONE',  ( 12.02609123740286101, 9.325023229212996867, -16.69214155778140096 ) ) ;
#2928=CARTESIAN_POINT ( 'NONE',  ( 32.54894808986480115, -9.611255921941241454, -17.86757894403779900 ) ) ;
#2929=CARTESIAN_POINT ( 'NONE',  ( 31.22280883588763700, -10.09333740185288875, -13.86128061636125786 ) ) ;
#2930=CARTESIAN_POINT ( 'NONE',  ( 29.90031526554274777, -7.862644070287768905, -16.42500436498598049 ) ) ;
#2934=PRODUCT_CONTEXT ( 'NONE', #26477, 'mechanical' ) ;
#2935=CARTESIAN_POINT ( 'NONE',  ( 18.57704598647189798, -1.039939211366111005, -17.60664924018008293 ) ) ;
#2936=CARTESIAN_POINT ( 'NONE',  ( 27.10702390817755614, -8.414881854042032927, -18.30456363717458146 ) ) ;
#2953=CARTESIAN_POINT ( 'NONE',  ( 12.24830724310059082, 9.517209185634078139, -15.33080109912759070 ) ) ;
#2957=CARTESIAN_POINT ( 'NONE',  ( 11.48043977940431226, 9.236673419044803879, -15.85762597608872326 ) ) ;
#2959=CARTESIAN_POINT ( 'NONE',  ( 23.26502027940742678, 3.673231887600847845, -16.77589761210995789 ) ) ;
#2966=CARTESIAN_POINT ( 'NONE',  ( 11.05552354607739929, 17.68892703645376585, -17.88069451076903249 ) ) ;
#2969=CARTESIAN_POINT ( 'NONE',  ( 35.54859390953724585, -21.18451583373416014, -17.64281456791166391 ) ) ;
#2971=CARTESIAN_POINT ( 'NONE',  ( 15.54217852991911997, 3.796156774867226247, -18.16774540469225485 ) ) ;
#2973=CARTESIAN_POINT ( 'NONE',  ( 9.057417708256320310, 16.43412612588882027, -17.11704294810955318 ) ) ;
#2974=CARTESIAN_POINT ( 'NONE',  ( 28.55206495951409096, -10.69471729813234795, -19.99811924356017911 ) ) ;
#2979=CARTESIAN_POINT ( 'NONE',  ( 23.41849298471255381, -3.203224238779429633, -13.27670244232306018 ) ) ;
#2980=CARTESIAN_POINT ( 'NONE',  ( 16.99436549934495133, 9.190724047982882894, -15.08166918603070528 ) ) ;
#2983=EDGE_CURVE ( 'NONE', #23709, #8851, #22290, .T. ) ;
#2992=CARTESIAN_POINT ( 'NONE',  ( 11.47652547240386944, 9.253065934422213701, -15.85936358228339316 ) ) ;
#2993=CARTESIAN_POINT ( 'NONE',  ( 26.84622329165386745, -11.42663724297536554, -16.80226328336580366 ) ) ;
#2994=CARTESIAN_POINT ( 'NONE',  ( 21.12965431673027794, -4.223434333162931154, -14.75790768142083031 ) ) ;
#2995=CARTESIAN_POINT ( 'NONE',  ( 32.62126879184269512, -11.04717877266006987, -18.30218954475424908 ) ) ;
#2999=CARTESIAN_POINT ( 'NONE',  ( 12.50736435846123484, 8.573956625762026107, -15.12430548898761806 ) ) ;
#3002=CARTESIAN_POINT ( 'NONE',  ( 21.04385110482095200, 5.766204710259658306, -15.30406332615466347 ) ) ;
#3004=CARTESIAN_POINT ( 'NONE',  ( 10.69507909363156628, 16.74911557172037391, -15.96836912279556309 ) ) ;
#3008=CARTESIAN_POINT ( 'NONE',  ( 17.96884874826282186, 1.586046385177752871, -19.67104016136476119 ) ) ;
#3009=CARTESIAN_POINT ( 'NONE',  ( 17.34455430865552472, 11.59597468841007384, -15.61519298676701695 ) ) ;
#3011=CARTESIAN_POINT ( 'NONE',  ( 34.93238815599637803, -19.41622979634004764, -20.17168434421570922 ) ) ;
#3013=CARTESIAN_POINT ( 'NONE',  ( 21.98307778806466928, -1.383504679822651795, -14.66368364926259460 ) ) ;
#3015=CARTESIAN_POINT ( 'NONE',  ( 18.61935276534875783, -1.259532457306228315, -15.72749031817820331 ) ) ;
#3016=CARTESIAN_POINT ( 'NONE',  ( 27.79808892257030806, -9.771933472778439267, -13.29678235002263165 ) ) ;
#3018=ORIENTED_EDGE ( 'NONE', *, *, #2895, .T. ) ;
#3025=CARTESIAN_POINT ( 'NONE',  ( 36.12281451779777797, -20.27171456826661355, -20.44288436412734100 ) ) ;
#3026=CARTESIAN_POINT ( 'NONE',  ( 9.641350810849047548, 17.66889113945805789, -17.95086732675817132 ) ) ;
#3029=CARTESIAN_POINT ( 'NONE',  ( 12.90142504057275197, 8.513187104919181181, -16.08590544042818493 ) ) ;
#3043=CARTESIAN_POINT ( 'NONE',  ( 11.23377902493292879, 9.047655202846097922, -17.23738383348171865 ) ) ;
#3044=CARTESIAN_POINT ( 'NONE',  ( 24.46642504186807088, -8.279991823955473507, -18.31266784446766493 ) ) ;
#3045=CARTESIAN_POINT ( 'NONE',  ( 20.86695504291294156, -3.984745147917406971, -17.88565525751875995 ) ) ;
#3056=CARTESIAN_POINT ( 'NONE',  ( 10.51251736658329961, 16.26646593658467310, -17.31805759646961462 ) ) ;
#3058=CARTESIAN_POINT ( 'NONE',  ( 33.66044826391103584, -12.70207762650279015, -18.74488588032081893 ) ) ;
#3060=CARTESIAN_POINT ( 'NONE',  ( 13.39626964006587428, 7.633314995549595139, -15.69459619883729928 ) ) ;
#3063=CARTESIAN_POINT ( 'NONE',  ( 24.52797215547132836, -1.897736678990579184, -19.26084780660264073 ) ) ;
#3064=CARTESIAN_POINT ( 'NONE',  ( 12.83519646890166577, 9.531778640408997916, -16.13946648208032641 ) ) ;
#3070=CARTESIAN_POINT ( 'NONE',  ( 11.47748818427356987, 9.248962635895034978, -15.85894168489154765 ) ) ;
#3075=CARTESIAN_POINT ( 'NONE',  ( 9.655099948573186097, 17.60583584124798051, -17.48406748397995614 ) ) ;
#3082=CARTESIAN_POINT ( 'NONE',  ( 11.50940939395034768, 11.69459202490242689, -16.90580767540677343 ) ) ;
#3084=CARTESIAN_POINT ( 'NONE',  ( 36.51148101492068321, -23.01778725746827803, -19.37219236604238759 ) ) ;
#3085=CARTESIAN_POINT ( 'NONE',  ( 27.20760296572909809, -8.488227175050779394, -13.35743234967312354 ) ) ;
#3086=CARTESIAN_POINT ( 'NONE',  ( 16.19004574127830054, 9.516462436566445859, -20.03842800660303070 ) ) ;
#3091=CARTESIAN_POINT ( 'NONE',  ( 33.07549275714919901, -10.34104163876563831, -17.35407900654646340 ) ) ;
#3093=CARTESIAN_POINT ( 'NONE',  ( 16.81761937449845234, 3.371063479271922514, -17.17107737352595720 ) ) ;
#3094=CARTESIAN_POINT ( 'NONE',  ( 19.23836061553175369, 5.151828676608854352, -13.99136221198299168 ) ) ;
#3102=CARTESIAN_POINT ( 'NONE',  ( 12.27682979692750997, 9.494989133591600350, -15.31072415319233215 ) ) ;
#3106=CARTESIAN_POINT ( 'NONE',  ( 12.44984726620633353, 8.550925603015029353, -15.16996558791898231 ) ) ;
#3110=CARTESIAN_POINT ( 'NONE',  ( 16.85369750842388825, 4.841181898090542113, -18.70119709635011418 ) ) ;
#3118=CARTESIAN_POINT ( 'NONE',  ( 12.83225144795546235, 9.540626470039393681, -16.14103964284477399 ) ) ;
#3120=CARTESIAN_POINT ( 'NONE',  ( 33.61336211056222112, -12.49217533051321993, -18.72970452740151970 ) ) ;
#3121=CARTESIAN_POINT ( 'NONE',  ( 17.88091890332929523, 4.544920326333207861, -13.91018511019278669 ) ) ;
#3123=CARTESIAN_POINT ( 'NONE',  ( 16.22940209442605308, 10.22534693890197133, -14.12725775589269084 ) ) ;
#3126=CARTESIAN_POINT ( 'NONE',  ( 21.59786356094703308, -0.7637721020719707710, -13.97513905925265298 ) ) ;
#3127=CARTESIAN_POINT ( 'NONE',  ( 16.47391574482200483, 4.481796633190492152, -18.19319569287263150 ) ) ;
#3139=CARTESIAN_POINT ( 'NONE',  ( 10.43540724046455992, 14.02724713458965233, -16.28994223329847202 ) ) ;
#3140=CARTESIAN_POINT ( 'NONE',  ( 29.29807706749550889, -8.594015191909356588, -15.50881839395299444 ) ) ;
#3141=CARTESIAN_POINT ( 'NONE',  ( 30.68845550234816244, -8.154108532121835395, -15.50657635367809917 ) ) ;
#3142=CARTESIAN_POINT ( 'NONE',  ( 33.37634376253905089, -12.42895282922877342, -19.69946502924221932 ) ) ;
#3152=CARTESIAN_POINT ( 'NONE',  ( 22.39939798857497877, 2.694615832958070722, -14.02792042734668065 ) ) ;
#3155=CARTESIAN_POINT ( 'NONE',  ( 12.26306961015461461, 9.515005556349402482, -15.31970085818224980 ) ) ;
#3158=CARTESIAN_POINT ( 'NONE',  ( 21.63873165585565417, 2.424707942738766331, -13.54651715722292060 ) ) ;
#3160=CARTESIAN_POINT ( 'NONE',  ( 21.48460829514769799, 2.948577479130256584, -19.81588663513211657 ) ) ;
#3162=CARTESIAN_POINT ( 'NONE',  ( 33.40713826534622655, -12.56408340279653757, -19.71064172033093698 ) ) ;
#3164=CARTESIAN_POINT ( 'NONE',  ( 25.66261690555348807, -4.931278859741150100, -13.05994810794548933 ) ) ;
#3165=CARTESIAN_POINT ( 'NONE',  ( 16.89975486243277913, 3.514059009776604015, -17.86885937027150817 ) ) ;
#3176=CARTESIAN_POINT ( 'NONE',  ( 18.00441060066494003, 9.543425513107552050, -19.87907960298149490 ) ) ;
#3177=CARTESIAN_POINT ( 'NONE',  ( 35.48977118337261771, -17.42778619908077076, -20.26990708652652629 ) ) ;
#3178=CARTESIAN_POINT ( 'NONE',  ( 10.82443827553465177, 12.24310121783546634, -16.12906421532448675 ) ) ;
#3181=CARTESIAN_POINT ( 'NONE',  ( 12.03842576178837298, 9.272001309349649389, -16.68677036593512497 ) ) ;
#3190=CARTESIAN_POINT ( 'NONE',  ( 11.22446318822032296, 9.088639264749929225, -17.24136893309019669 ) ) ;
#3192=CARTESIAN_POINT ( 'NONE',  ( 24.94601217299843654, -12.81575267032737742, -15.97323768315044035 ) ) ;
#3193=CARTESIAN_POINT ( 'NONE',  ( 26.55721583451634160, -2.971036115494387175, -18.36415422809029607 ) ) ;
#3205=CARTESIAN_POINT ( 'NONE',  ( 11.96327893486549776, 9.613088455355432771, -16.71811665443363992 ) ) ;
#3206=CARTESIAN_POINT ( 'NONE',  ( 35.54859390953724585, -22.18451583373416014, -17.22552805718784441 ) ) ;
#3208=CARTESIAN_POINT ( 'NONE',  ( 9.436770671236972774, 14.69436508140356246, -16.92063988783295159 ) ) ;
#3210=CARTESIAN_POINT ( 'NONE',  ( 23.77086030874127687, -7.150112426529108944, -14.59934731766091431 ) ) ;
#3211=CARTESIAN_POINT ( 'NONE',  ( 12.83227036137552446, 9.540540802112166929, -16.14103173976383587 ) ) ;
#3214=CARTESIAN_POINT ( 'NONE',  ( 11.51951884677450266, 9.108496074915260365, -15.83757232928968683 ) ) ;
#3216=CARTESIAN_POINT ( 'NONE',  ( 11.47269659055779378, 9.270105954394804115, -15.86098659800193644 ) ) ;
#3221=CARTESIAN_POINT ( 'NONE',  ( 11.70392491148546732, 10.80251906652491556, -16.82536866641744311 ) ) ;
#3224=CARTESIAN_POINT ( 'NONE',  ( 36.54859390953724585, -23.18451583373416014, -16.94733705004010105 ) ) ;
#3225=CARTESIAN_POINT ( 'NONE',  ( 25.90632082398269276, -12.28056132945115841, -15.12647891527467969 ) ) ;
#3226=CARTESIAN_POINT ( 'NONE',  ( 14.03447742461322534, 10.03307406631979326, -15.27079475659193086 ) ) ;
#3231=CARTESIAN_POINT ( 'NONE',  ( 36.54859390953724585, -22.18451583373416014, -16.94733705004010460 ) ) ;
#3233=CARTESIAN_POINT ( 'NONE',  ( 17.18133768520950255, 3.791981501156216350, -18.48732239789962506 ) ) ;
#3235=CARTESIAN_POINT ( 'NONE',  ( 19.20291185354690811, 8.143073066566493878, -16.32372945079811188 ) ) ;
#3249=CARTESIAN_POINT ( 'NONE',  ( 12.27129069473257239, 9.507470051170034964, -15.31400031939534045 ) ) ;
#3255=CARTESIAN_POINT ( 'NONE',  ( 11.69419402147360110, 8.800013620902292999, -15.72776802682527730 ) ) ;
#3257=CARTESIAN_POINT ( 'NONE',  ( 19.77054944300549622, 4.331964111641410042, -19.42026316723860901 ) ) ;
#3263=CARTESIAN_POINT ( 'NONE',  ( 12.85347977544317111, 9.515020184875311315, -16.12678873937763413 ) ) ;
#3265=CARTESIAN_POINT ( 'NONE',  ( 36.36958547251401797, -20.38032574959806098, -19.43068663056894252 ) ) ;
#3266=CARTESIAN_POINT ( 'NONE',  ( 14.57776618122778700, 6.338444840345393239, -15.85465340776532095 ) ) ;
#3269=CARTESIAN_POINT ( 'NONE',  ( 15.02162844583664736, 5.759011576665847620, -14.59661587647459591 ) ) ;
#3272=CARTESIAN_POINT ( 'NONE',  ( 26.55721583451634160, -2.971036115494387175, -18.36415422809029607 ) ) ;
#3273=CARTESIAN_POINT ( 'NONE',  ( 20.29966856415212817, 4.923229158599749411, -18.85509502865480869 ) ) ;
#3287=CARTESIAN_POINT ( 'NONE',  ( 11.82447321682112751, 8.672047275158794477, -15.63808403058127006 ) ) ;
#3288=CARTESIAN_POINT ( 'NONE',  ( 25.57659404178318141, -9.842204813007603192, -16.83936284125123706 ) ) ;
#3289=CARTESIAN_POINT ( 'NONE',  ( 24.97892660363778106, -6.291154998746494087, -12.74939059104742256 ) ) ;
#3290=CARTESIAN_POINT ( 'NONE',  ( 32.89062095351589932, -11.25267498498577723, -18.96775996542842435 ) ) ;
#3299=CARTESIAN_POINT ( 'NONE',  ( 19.50856600871340873, -1.908691058934758100, -18.90332006808282728 ) ) ;
#3302=CARTESIAN_POINT ( 'NONE',  ( 11.62855932722735908, 12.46805622939721836, -15.57880556977976916 ) ) ;
#3304=CARTESIAN_POINT ( 'NONE',  ( 33.10952763335142635, -11.62914684427059697, -19.38687730282833499 ) ) ;
#3307=CARTESIAN_POINT ( 'NONE',  ( 25.21413058671614849, -1.115224416820481457, -18.44856734933592080 ) ) ;
#3308=CARTESIAN_POINT ( 'NONE',  ( 17.05458169553830317, 2.837819561348359887, -13.69156784695313611 ) ) ;
#3310=CARTESIAN_POINT ( 'NONE',  ( 32.77977724007769211, -11.13765286058784554, -18.71157503069099448 ) ) ;
#3311=CARTESIAN_POINT ( 'NONE',  ( 25.92665957894408280, -9.004797978260709712, -12.14503282074142909 ) ) ;
#3312=CARTESIAN_POINT ( 'NONE',  ( 24.07185007603571592, -6.521566527568181115, -20.06683206624251525 ) ) ;
#3313=CARTESIAN_POINT ( 'NONE',  ( 25.23810427664335165, -6.496417100615061280, -13.69959235629456629 ) ) ;
#3324=CARTESIAN_POINT ( 'NONE',  ( 16.36264732604271899, 7.873549196589271659, -20.78255227469630739 ) ) ;
#3325=CARTESIAN_POINT ( 'NONE',  ( 36.18478257229246964, -20.55010421171508028, -20.40673782175607442 ) ) ;
#3326=CARTESIAN_POINT ( 'NONE',  ( 9.957223259857686415, 16.22025982393231303, -16.48768813039480818 ) ) ;
#3329=CARTESIAN_POINT ( 'NONE',  ( 12.02805304935487563, 9.316025821727821565, -16.69133030147860453 ) ) ;
#3339=CARTESIAN_POINT ( 'NONE',  ( 11.22879857168519813, 9.069188343361037852, -17.23954317433854300 ) ) ;
#3341=CARTESIAN_POINT ( 'NONE',  ( 27.55585723563325473, -10.26521964199731407, -19.78748283923107820 ) ) ;
#3342=CARTESIAN_POINT ( 'NONE',  ( 22.09907825138052218, -7.445301066569870230, -16.29136317631293807 ) ) ;
#3353=CARTESIAN_POINT ( 'NONE',  ( 12.02932678857878734, 9.310239991255825132, -16.69079931733866218 ) ) ;
#3354=CARTESIAN_POINT ( 'NONE',  ( 31.77493940018505114, -11.56844746753418640, -13.90849911728625266 ) ) ;
#3357=CARTESIAN_POINT ( 'NONE',  ( 9.110807846758516959, 16.18927214505777812, -17.05547580459120383 ) ) ;
#3358=CARTESIAN_POINT ( 'NONE',  ( 21.54098841764929873, -5.100688324319140321, -15.19385678519978633 ) ) ;
#3359=CARTESIAN_POINT ( 'NONE',  ( 12.82210747586494293, 9.587147947373788170, -16.14523453761016825 ) ) ;
#3365=CARTESIAN_POINT ( 'NONE',  ( 11.47338783222600789, 9.266948822715743717, -15.86069975447064806 ) ) ;
#3370=CARTESIAN_POINT ( 'NONE',  ( 12.02871927673971619, 9.312984558958580905, -16.69105371450780595 ) ) ;
#3373=CARTESIAN_POINT ( 'NONE',  ( 20.04052888069229610, 8.940267654624740601, -17.40200224619232117 ) ) ;
#3374=CARTESIAN_POINT ( 'NONE',  ( 16.83828815103352028, 11.11029360287396983, -16.41243972054167344 ) ) ;
#3378=CARTESIAN_POINT ( 'NONE',  ( 17.06466135374324011, 3.680263393506696179, -18.28590298471088005 ) ) ;
#3380=CARTESIAN_POINT ( 'NONE',  ( 15.14574614762244487, 6.587483969391940697, -15.14885142785537830 ) ) ;
#3385=CARTESIAN_POINT ( 'NONE',  ( 12.89848499353137434, 9.804829592035655850, -14.81257543908856000 ) ) ;
#3387=CARTESIAN_POINT ( 'NONE',  ( 12.27681432698556918, 9.495076167121005994, -15.31072932366845407 ) ) ;
#3392=CARTESIAN_POINT ( 'NONE',  ( 12.53458732174692258, 8.585986940276173485, -15.10260830673100330 ) ) ;
#3394=CARTESIAN_POINT ( 'NONE',  ( 10.50660601767968139, 9.787963810330234438, -16.47822533839871539 ) ) ;
#3401=CARTESIAN_POINT ( 'NONE',  ( 12.84461350077944886, 9.519659821018855439, -16.13320262440205966 ) ) ;
#3404=CARTESIAN_POINT ( 'NONE',  ( 34.39665924806198660, -11.72086467124742981, -18.77862448471655199 ) ) ;
#3405=CARTESIAN_POINT ( 'NONE',  ( 16.06572049258021195, 3.735912457719189117, -15.00855390560170477 ) ) ;
#3409=CARTESIAN_POINT ( 'NONE',  ( 25.50411877999659893, -13.63830170496968996, -16.08255890605547123 ) ) ;
#3413=CARTESIAN_POINT ( 'NONE',  ( 24.52508672555368463, -0.3756359333432500169, -18.08805785897195051 ) ) ;
#3414=CARTESIAN_POINT ( 'NONE',  ( 19.73758642798775753, -1.564653675968832314, -13.27997001701493041 ) ) ;
#3425=CARTESIAN_POINT ( 'NONE',  ( 9.949118446627077006, 16.25742953053141804, -16.49103975576934644 ) ) ;
#3426=CARTESIAN_POINT ( 'NONE',  ( 29.41685937463160272, -8.713933360145817986, -16.19581194183416883 ) ) ;
#3427=CARTESIAN_POINT ( 'NONE',  ( 23.43951749033787735, -6.062008688038916127, -19.28752554440484701 ) ) ;
#3432=CIRCLE ( 'NONE', #2494, 0.4999999999999986677 ) ;
#3436=CARTESIAN_POINT ( 'NONE',  ( 19.40121574091639189, 1.432572567346982240, -13.43353846741550406 ) ) ;
#3439=CARTESIAN_POINT ( 'NONE',  ( 12.27691635572497830, 9.494607244959519576, -15.31068720787289728 ) ) ;
#3442=CARTESIAN_POINT ( 'NONE',  ( 32.30218501430429967, -10.99871056796995816, -17.40035725849610060 ) ) ;
#3446=CARTESIAN_POINT ( 'NONE',  ( 16.94076125623460527, 0.4124075662712927692, -16.40086227390004936 ) ) ;
#3448=ADVANCED_FACE ( 'NONE', ( #27137 ), #5061, .F. ) ;
#3449=CARTESIAN_POINT ( 'NONE',  ( 19.77430725462212635, 0.2453161447429414443, -14.21425550582737074 ) ) ;
#3452=CARTESIAN_POINT ( 'NONE',  ( 22.52525573827019301, -5.869110285238294367, -18.12586539066504798 ) ) ;
#3453=CARTESIAN_POINT ( 'NONE',  ( 19.78633661418711043, -4.982883274218824710, -16.00186916550291727 ) ) ;
#3456=CARTESIAN_POINT ( 'NONE',  ( 26.08768104250457753, -11.87935956797728210, -17.28510650846989805 ) ) ;
#3464=CARTESIAN_POINT ( 'NONE',  ( 34.41982446195410716, -12.62108234628556680, -19.94648786050102274 ) ) ;
#3465=CARTESIAN_POINT ( 'NONE',  ( 9.997747326010761881, 16.03441129093729245, -16.47093000352221637 ) ) ;
#3468=CARTESIAN_POINT ( 'NONE',  ( 13.55939796120610019, 8.763434079353435990, -15.56458004748339619 ) ) ;
#3484=CARTESIAN_POINT ( 'NONE',  ( 11.22423757029256741, 9.089670537749404033, -17.24146249637195183 ) ) ;
#3488=CARTESIAN_POINT ( 'NONE',  ( 26.88742137321887427, -10.86886578961255978, -19.57440296808016100 ) ) ;
#3489=CARTESIAN_POINT ( 'NONE',  ( 22.33774198005919587, -7.088069534354142220, -17.87445411435389886 ) ) ;
#3493=VERTEX_POINT ( 'NONE', #4807 ) ;
#3502=CARTESIAN_POINT ( 'NONE',  ( 13.12216094266758581, 8.570213704404382682, -15.91306547940487448 ) ) ;
#3503=CARTESIAN_POINT ( 'NONE',  ( 35.13870703111577143, -20.34311121210408757, -20.23074448643712486 ) ) ;
#3505=CARTESIAN_POINT ( 'NONE',  ( 9.112223960064733674, 16.18277766892301983, -17.05485288603163951 ) ) ;
#3506=CARTESIAN_POINT ( 'NONE',  ( 26.04489551603160180, -6.130266781319400948, -13.71289979607875154 ) ) ;
#3507=CARTESIAN_POINT ( 'NONE',  ( 10.35865005771744762, 16.97212102856341787, -17.91352035578586310 ) ) ;
#3512=CARTESIAN_POINT ( 'NONE',  ( 12.50016782010997751, 8.570776461014483871, -15.13004124836345632 ) ) ;
#3518=CARTESIAN_POINT ( 'NONE',  ( 13.05603179413191839, 8.545058472539723837, -15.96546128479914373 ) ) ;
#3520=CARTESIAN_POINT ( 'NONE',  ( 21.27922114827105204, 3.617311378231426566, -20.53498548623805675 ) ) ;
#3521=CARTESIAN_POINT ( 'NONE',  ( 19.69280650922798515, 8.111729275751024204, -19.45082099569356160 ) ) ;
#3524=CARTESIAN_POINT ( 'NONE',  ( 36.30362226317071617, -21.08398799169651738, -20.22680612736627026 ) ) ;
#3526=CARTESIAN_POINT ( 'NONE',  ( 15.78240017141095741, 4.038647184180326200, -18.77507866864583619 ) ) ;
#3533=CARTESIAN_POINT ( 'NONE',  ( 35.13870703111577143, -20.34311121210408757, -20.23074448643712486 ) ) ;
#3537=CARTESIAN_POINT ( 'NONE',  ( 12.27692691330339514, 9.494559429826583852, -15.31068279593241144 ) ) ;
#3541=CARTESIAN_POINT ( 'NONE',  ( 12.49664108868010182, 8.569232744350554043, -15.13285098609708790 ) ) ;
#3544=CARTESIAN_POINT ( 'NONE',  ( 11.38288633050183307, 7.831121701799675705, -15.95859485361821939 ) ) ;
#3551=CARTESIAN_POINT ( 'NONE',  ( 12.81197645932666163, 9.633610080622574401, -16.14942406932820163 ) ) ;
#3553=CARTESIAN_POINT ( 'NONE',  ( 33.94960473074984009, -11.12362044852780407, -17.82291586202971700 ) ) ;
#3554=CARTESIAN_POINT ( 'NONE',  ( 23.66272512268759343, 2.894330346666426745, -16.12005855839824520 ) ) ;
#3558=CARTESIAN_POINT ( 'NONE',  ( 28.19717681610909210, -11.01075670644066662, -19.96981485020118541 ) ) ;
#3563=CARTESIAN_POINT ( 'NONE',  ( 20.53420570626898822, -0.4664991210283321310, -19.04361528682417415 ) ) ;
#3564=CARTESIAN_POINT ( 'NONE',  ( 19.61234978942155038, 5.539603999143367652, -15.30853080630118512 ) ) ;
#3577=CARTESIAN_POINT ( 'NONE',  ( 11.46269231744662420, 9.315986823159681407, -15.86512371708112212 ) ) ;
#3578=CARTESIAN_POINT ( 'NONE',  ( 17.17204249742301059, 10.23148044644768362, -15.96021614775051667 ) ) ;
#3579=CARTESIAN_POINT ( 'NONE',  ( 29.30807694892355286, -8.357723062633453992, -13.20244061823602522 ) ) ;
#3586=CARTESIAN_POINT ( 'NONE',  ( 21.40051611374530793, -0.1690565882708310874, -20.18282279970310000 ) ) ;
#3589=CARTESIAN_POINT ( 'NONE',  ( 12.27644674946102832, 9.496504630232381672, -15.31090095340427304 ) ) ;
#3591=CARTESIAN_POINT ( 'NONE',  ( 18.50902107916489570, 2.085137940960992697, -20.06823964296112450 ) ) ;
#3593=CARTESIAN_POINT ( 'NONE',  ( 20.23665759668125474, 8.554704514664523529, -15.35188933034790182 ) ) ;
#3596=CARTESIAN_POINT ( 'NONE',  ( 28.15806058933612022, -5.108324757233392077, -18.51472486207664758 ) ) ;
#3597=CARTESIAN_POINT ( 'NONE',  ( 22.44149885728860028, -8.037961521189897596, -18.19026436706728234 ) ) ;
#3612=CARTESIAN_POINT ( 'NONE',  ( 28.02170931380428698, -7.325026966936788675, -12.85224998211816860 ) ) ;
#3614=CARTESIAN_POINT ( 'NONE',  ( 33.97319001242765779, -11.13623552147873141, -19.50814438409551954 ) ) ;
#3616=CARTESIAN_POINT ( 'NONE',  ( 9.918725397012197575, 16.39681593027784956, -16.50360835092378409 ) ) ;
#3620=CARTESIAN_POINT ( 'NONE',  ( 13.12341270237516078, 8.570764515250925086, -15.91206798513452192 ) ) ;
#3629=CARTESIAN_POINT ( 'NONE',  ( 8.944584683310379702, 16.95159276115599667, -17.91796598306941135 ) ) ;
#3630=CARTESIAN_POINT ( 'NONE',  ( 16.69609108537820674, 9.478167028156011753, -20.90851310094495474 ) ) ;
#3631=CARTESIAN_POINT ( 'NONE',  ( 30.27313844582349489, -8.115497507854934511, -14.41531361995715876 ) ) ;
#3638=DIRECTION ( 'NONE',  ( -0.06678507476159963041, 0.9947851038922184141, -0.07708664516786083165 ) ) ;
#3647=CARTESIAN_POINT ( 'NONE',  ( 12.04525852301462585, 9.245982119944198274, -16.68353927915122981 ) ) ;
#3648=CARTESIAN_POINT ( 'NONE',  ( 32.25667210025905263, -11.64161264113965011, -15.27003429613047025 ) ) ;
#3650=CARTESIAN_POINT ( 'NONE',  ( 8.946690830082905777, 16.94193370358561879, -17.78270686867927708 ) ) ;
#3652=CARTESIAN_POINT ( 'NONE',  ( 25.31619048431776875, -0.2099727537683927225, -15.56338435260822628 ) ) ;
#3653=CARTESIAN_POINT ( 'NONE',  ( 12.86836073382838563, 9.516082146233362238, -16.11534891376273748 ) ) ;
#3659=CARTESIAN_POINT ( 'NONE',  ( 11.48249212886396897, 9.228508165798535501, -15.85668214399537845 ) ) ;
#3664=CARTESIAN_POINT ( 'NONE',  ( 9.661883079970770893, 16.25482654942367233, -17.91569817988508362 ) ) ;
#3666=CARTESIAN_POINT ( 'NONE',  ( 14.64418905516944314, 2.941711854493593403, -16.63492386420942282 ) ) ;
#3667=CARTESIAN_POINT ( 'NONE',  ( 20.94368124868196901, 3.275021729503806878, -20.72479390824751633 ) ) ;
#3672=CARTESIAN_POINT ( 'NONE',  ( 19.05868480923028940, 8.129737193291200370, -16.02886444249750042 ) ) ;
#3680=CARTESIAN_POINT ( 'NONE',  ( 32.77977724007769211, -11.13765286058784554, -18.71157503069099448 ) ) ;
#3684=CARTESIAN_POINT ( 'NONE',  ( 12.27235684156208961, 9.528132359803098694, -15.31161062812042317 ) ) ;
#3691=CARTESIAN_POINT ( 'NONE',  ( 10.67054149815029618, 9.036200773601834157, -16.41042721873081689 ) ) ;
#3697=CARTESIAN_POINT ( 'NONE',  ( 12.83226850357503501, 9.540548187773516986, -16.14103259455261608 ) ) ;
#3699=CARTESIAN_POINT ( 'NONE',  ( 34.22536682013040377, -11.37642754387024979, -18.47965768629886085 ) ) ;
#3700=CARTESIAN_POINT ( 'NONE',  ( 20.72626264887238534, -1.914771856900582714, -13.62749948506543518 ) ) ;
#3705=CARTESIAN_POINT ( 'NONE',  ( 26.19910047366428429, -13.48590472426672626, -13.82108881675422829 ) ) ;
#3710=CARTESIAN_POINT ( 'NONE',  ( 30.27313844582349489, -8.115497507854934511, -14.41531361995715876 ) ) ;
#3712=CARTESIAN_POINT ( 'NONE',  ( 20.76503381105741397, 0.5146303624313508518, -20.54264311693622602 ) ) ;
#3724=CARTESIAN_POINT ( 'NONE',  ( 13.35290877858212255, 7.614465999429414822, -15.72913170295453966 ) ) ;
#3726=CARTESIAN_POINT ( 'NONE',  ( 16.84948243412402036, 10.49281628697410262, -11.66356073909478575 ) ) ;
#3727=CARTESIAN_POINT ( 'NONE',  ( 24.40455984355908114, -10.10244183743681035, -17.68366952546245585 ) ) ;
#3732=CARTESIAN_POINT ( 'NONE',  ( 9.893572868141015775, 16.51216863388285461, -16.51808063826580408 ) ) ;
#3734=CARTESIAN_POINT ( 'NONE',  ( 25.57370974413349884, -0.4222200280313516685, -16.88676729435558599 ) ) ;
#3738=CARTESIAN_POINT ( 'NONE',  ( 11.04501277462238029, 15.14427510452705583, -15.82012259674246657 ) ) ;
#3739=CARTESIAN_POINT ( 'NONE',  ( 32.67186286342521839, -11.06527230177895227, -18.43913201350460440 ) ) ;
#3741=CARTESIAN_POINT ( 'NONE',  ( 25.07290406138036687, -9.006318079059196791, -17.79994936451110732 ) ) ;
#3743=CARTESIAN_POINT ( 'NONE',  ( 21.98221344960014889, 4.819993630401092410, -14.81438138791982162 ) ) ;
#3748=CARTESIAN_POINT ( 'NONE',  ( 23.96437976099892708, -9.208260125601851698, -18.67152130837153123 ) ) ;
#3750=CARTESIAN_POINT ( 'NONE',  ( 23.15972007162554291, -8.148303969466700991, -13.79129035937103431 ) ) ;
#3763=CARTESIAN_POINT ( 'NONE',  ( 26.82298874931487020, -4.830090842487210878, -14.67398021261910301 ) ) ;
#3765=CARTESIAN_POINT ( 'NONE',  ( 34.10649047503919462, -12.21345526111254287, -20.89408644300621987 ) ) ;
#3768=CARTESIAN_POINT ( 'NONE',  ( 9.916551108984865692, 16.40678749232849398, -16.50450761325770443 ) ) ;
#3771=CARTESIAN_POINT ( 'NONE',  ( 9.661883079970770893, 16.25482654942367233, -17.91569817988508362 ) ) ;
#3774=CARTESIAN_POINT ( 'NONE',  ( 9.926830210242822972, 16.35964622367879784, -16.50025672554925293 ) ) ;
#3780=CARTESIAN_POINT ( 'NONE',  ( 13.65148492087865151, 7.746099194123166498, -15.49118511517110619 ) ) ;
#3781=CARTESIAN_POINT ( 'NONE',  ( 36.54859390953724585, -23.18451583373416014, -17.78191007148576119 ) ) ;
#3784=CARTESIAN_POINT ( 'NONE',  ( 30.21326039400183561, -7.476461571224066738, -17.86537319528562051 ) ) ;
#3786=CARTESIAN_POINT ( 'NONE',  ( 22.98083118076628040, -7.181321033737746440, -13.97658420854277850 ) ) ;
#3796=PRESENTATION_STYLE_ASSIGNMENT (( #20554 ) ) ;
#3800=CARTESIAN_POINT ( 'NONE',  ( 12.05017172662707381, 9.228765020691243492, -16.68110209197688221 ) ) ;
#3801=CARTESIAN_POINT ( 'NONE',  ( 35.54582861202835886, -21.17209281684672817, -18.49356017204852520 ) ) ;
#3803=CARTESIAN_POINT ( 'NONE',  ( 9.113084692838755885, 16.17883023870341930, -17.05449542622726966 ) ) ;
#3805=CARTESIAN_POINT ( 'NONE',  ( 24.68825858685077179, -9.385095155728059524, -16.92495907518576104 ) ) ;
#3806=CARTESIAN_POINT ( 'NONE',  ( 10.35864918915110877, 16.97212501191939538, -17.92454625180715766 ) ) ;
#3812=CARTESIAN_POINT ( 'NONE',  ( 11.47288049726737214, 9.269262779257836371, -15.86091052746238184 ) ) ;
#3817=CARTESIAN_POINT ( 'NONE',  ( 13.12489394565217005, 8.571418981294288031, -15.91088741739120671 ) ) ;
#3819=CARTESIAN_POINT ( 'NONE',  ( 19.58395429099637752, 5.031901065175194532, -13.05446103591450147 ) ) ;
#3820=CARTESIAN_POINT ( 'NONE',  ( 21.27922114827105204, 3.617311378231426566, -20.53498548623805675 ) ) ;
#3821=EDGE_CURVE ( 'NONE', #2433, #29043, #12772, .T. ) ;
#3826=CARTESIAN_POINT ( 'NONE',  ( 36.04209255463945993, -19.90907354740926394, -20.43687144983462289 ) ) ;
#3827=CARTESIAN_POINT ( 'NONE',  ( 18.34549112274340033, 0.9605221043122941227, -13.99314825615798341 ) ) ;
#3839=CARTESIAN_POINT ( 'NONE',  ( 12.24523086077475220, 9.516144614896692389, -15.33323053563244898 ) ) ;
#3840=CARTESIAN_POINT ( 'NONE',  ( 32.57315965809380742, -11.03986597812349935, -18.16622079659612510 ) ) ;
#3845=CARTESIAN_POINT ( 'NONE',  ( 12.74005437760208181, 7.618877980503234504, -14.93883819022932080 ) ) ;
#3851=CARTESIAN_POINT ( 'NONE',  ( 10.35864918915110877, 16.97212501191939538, -17.92981046679734547 ) ) ;
#3853=CARTESIAN_POINT ( 'NONE',  ( 33.92041909680281719, -11.11917911243856238, -17.74043268107170235 ) ) ;
#3854=CARTESIAN_POINT ( 'NONE',  ( 22.29983652437130814, 0.6627547066652448304, -20.09853802436992964 ) ) ;
#3864=CARTESIAN_POINT ( 'NONE',  ( 24.27430760268559595, -10.23567508289028716, -17.26834523416827949 ) ) ;
#3865=CARTESIAN_POINT ( 'NONE',  ( 27.87740037347163735, -3.310382910926334521, -16.69022314910379734 ) ) ;
#3875=CARTESIAN_POINT ( 'NONE',  ( 11.46306169112780537, 8.437560028716553973, -17.10890052424691632 ) ) ;
#3876=CARTESIAN_POINT ( 'NONE',  ( 12.50162201464318557, 8.571418981294288031, -15.12888223836978341 ) ) ;
#3886=CARTESIAN_POINT ( 'NONE',  ( 25.04992766293576878, -3.547109489677171101, -13.67097983722207033 ) ) ;
#3890=CARTESIAN_POINT ( 'NONE',  ( 12.24710219714225268, 9.516853694884586545, -15.33174803936941366 ) ) ;
#3894=CARTESIAN_POINT ( 'NONE',  ( 25.04068920418659161, -5.475481712173364990, -18.92835678451453774 ) ) ;
#3896=CARTESIAN_POINT ( 'NONE',  ( 22.92155253933561809, -3.178009374129639131, -14.34666800710537693 ) ) ;
#3901=CARTESIAN_POINT ( 'NONE',  ( 16.06097560829885040, 7.604535090956617616, -20.76572858943923094 ) ) ;
#3902=CARTESIAN_POINT ( 'NONE',  ( 27.27607810006200140, -2.061267822988343656, -14.60586277656102006 ) ) ;
#3905=CARTESIAN_POINT ( 'NONE',  ( 29.88803641097454999, -7.968445601786871002, -16.75847372370488131 ) ) ;
#3913=CARTESIAN_POINT ( 'NONE',  ( 25.04433344647707571, -4.420048373160954114, -18.22226412361657921 ) ) ;
#3914=CARTESIAN_POINT ( 'NONE',  ( 19.30972751531945519, 5.994221256738944348, -19.84686166629000326 ) ) ;
#3916=CARTESIAN_POINT ( 'NONE',  ( 34.26516872548082659, -12.92629604573065549, -20.94206068969455004 ) ) ;
#3919=CARTESIAN_POINT ( 'NONE',  ( 11.47288049726737214, 9.269262779257836371, -15.86091052746238184 ) ) ;
#3923=CARTESIAN_POINT ( 'NONE',  ( 13.12278719711289732, 8.570488965836000617, -15.91256645732111430 ) ) ;
#3926=CARTESIAN_POINT ( 'NONE',  ( 11.47338783222600789, 9.266948822715743717, -15.86069975447064806 ) ) ;
#3932=CARTESIAN_POINT ( 'NONE',  ( 8.944914148442956403, 16.95008179206086396, -17.86239244656949765 ) ) ;
#3933=CARTESIAN_POINT ( 'NONE',  ( 31.96909791962396596, -10.29830001063286460, -18.46063605759182735 ) ) ;
#3935=CARTESIAN_POINT ( 'NONE',  ( 18.76228799092704236, 0.4007544294800896578, -19.29634928253052806 ) ) ;
#3937=CARTESIAN_POINT ( 'NONE',  ( 27.61484239614359737, -11.78684095324212855, -18.66559939683001446 ) ) ;
#3941=CARTESIAN_POINT ( 'NONE',  ( 18.31666763169264911, 2.112308299563359970, -18.35152529819803746 ) ) ;
#3950=CARTESIAN_POINT ( 'NONE',  ( 12.03842576178837298, 9.272001309349649389, -16.68677036593512497 ) ) ;
#3953=CARTESIAN_POINT ( 'NONE',  ( 35.54859390953723164, -21.18451583373416014, -14.99999999999999822 ) ) ;
#3956=CARTESIAN_POINT ( 'NONE',  ( 10.66984875114861886, 9.039338215604900029, -16.41071671300888823 ) ) ;
#3959=CARTESIAN_POINT ( 'NONE',  ( 27.20760296572909809, -8.488227175050779394, -13.35743234967312354 ) ) ;
#3960=CARTESIAN_POINT ( 'NONE',  ( 12.93646321750111916, 9.546177831575306527, -16.06107003375496944 ) ) ;
#3966=CARTESIAN_POINT ( 'NONE',  ( 12.50481220565295004, 8.572828783776230921, -15.12633959982445653 ) ) ;
#3970=CARTESIAN_POINT ( 'NONE',  ( 13.25994536507779742, 8.631100619704961119, -15.80324905228922994 ) ) ;
#3971=CARTESIAN_POINT ( 'NONE',  ( 20.85347709306256547, 5.504344946561741558, -13.72608531385973407 ) ) ;
#3972=CARTESIAN_POINT ( 'NONE',  ( 18.68383238644686273, 8.832144196210188980, -14.76942027321762119 ) ) ;
#3977=CARTESIAN_POINT ( 'NONE',  ( 18.80472905218952917, 2.352968372735388503, -20.19605574946481497 ) ) ;
#3983=CARTESIAN_POINT ( 'NONE',  ( 34.96805304670973413, -19.57645325810014114, -20.18246498508359466 ) ) ;
#3986=ADVANCED_FACE ( 'NONE', ( #22303 ), #15573, .F. ) ;
#3990=CARTESIAN_POINT ( 'NONE',  ( 11.05541531668977662, 17.68942339022145305, -17.91796598306941135 ) ) ;
#3994=CARTESIAN_POINT ( 'NONE',  ( 9.641351021852148762, 17.66889017177091503, -17.91406276888456617 ) ) ;
#4000=CARTESIAN_POINT ( 'NONE',  ( 10.35864918915110877, 16.97212501191939538, -17.91664992932186351 ) ) ;
#4001=CARTESIAN_POINT ( 'NONE',  ( 35.48977118337261771, -17.42778619908077076, -20.26990708652652629 ) ) ;
#4002=CARTESIAN_POINT ( 'NONE',  ( 21.42923412144385509, -1.598955984811285536, -13.33006947543598741 ) ) ;
#4008=CARTESIAN_POINT ( 'NONE',  ( 30.58006126958193249, -8.114715823802763239, -15.12008790671442426 ) ) ;
#4009=CARTESIAN_POINT ( 'NONE',  ( 27.81650010061016332, -6.490163795910067535, -14.16582606047713178 ) ) ;
#4020=CARTESIAN_POINT ( 'NONE',  ( 11.22637516657937162, 9.079975409179585455, -17.24057027585384105 ) ) ;
#4023=CARTESIAN_POINT ( 'NONE',  ( 12.71834232392635045, 8.667191563245470576, -14.95615232649864090 ) ) ;
#4025=CARTESIAN_POINT ( 'NONE',  ( 30.78125299044525320, -8.317598597646391312, -16.28273480984023891 ) ) ;
#4029=CARTESIAN_POINT ( 'NONE',  ( 9.641350810849047548, 17.66889113945805789, -21.33333333332589277 ) ) ;
#4034=CARTESIAN_POINT ( 'NONE',  ( 22.34083945069921739, -4.755659482961629436, -14.12236044035638116 ) ) ;
#4038=CARTESIAN_POINT ( 'NONE',  ( 12.68070129083326236, 9.708587077508630259, -14.98615289428795094 ) ) ;
#4039=CARTESIAN_POINT ( 'NONE',  ( 33.15992091288699584, -11.77879734164826786, -17.82291275646110407 ) ) ;
#4041=CARTESIAN_POINT ( 'NONE',  ( 26.47511176763426377, -7.718147522161595830, -18.64721581247919602 ) ) ;
#4043=CARTESIAN_POINT ( 'NONE',  ( 20.36893440901172170, -1.919154233093003814, -17.42624063329192552 ) ) ;
#4046=( NAMED_UNIT ( * ) SI_UNIT ( $, .STERADIAN. ) SOLID_ANGLE_UNIT ( ) );
#4047=CARTESIAN_POINT ( 'NONE',  ( 13.86827785273622737, 5.312354197023893221, -16.63408457058017120 ) ) ;
#4049=CARTESIAN_POINT ( 'NONE',  ( 29.48152472672500579, -5.877396966218813468, -15.70213184580788379 ) ) ;
#4053=CARTESIAN_POINT ( 'NONE',  ( 25.97851742199650005, -11.98992670343847244, -16.97112261376066655 ) ) ;
#4062=CARTESIAN_POINT ( 'NONE',  ( 9.641350810849047548, 17.66889113945805789, -17.97192418671891190 ) ) ;
#4064=CARTESIAN_POINT ( 'NONE',  ( 25.84319962709097140, -7.021413190281159622, -18.98986798778381058 ) ) ;
#4065=CARTESIAN_POINT ( 'NONE',  ( 18.12654306171327079, 0.8625984663607378922, -18.09208126113620452 ) ) ;
#4066=CARTESIAN_POINT ( 'NONE',  ( 35.12112610261377910, -16.77165912796762726, -21.20079607051596327 ) ) ;
#4068=CARTESIAN_POINT ( 'NONE',  ( 12.29195110325218288, 8.516770644378290456, -15.29309475950548958 ) ) ;
#4071=CARTESIAN_POINT ( 'NONE',  ( 13.13063628947021755, 8.573956625762026107, -15.90631066800904669 ) ) ;
#4075=CARTESIAN_POINT ( 'NONE',  ( 12.37169234869624646, 8.529253869913038244, -15.23127513898213081 ) ) ;
#4083=CARTESIAN_POINT ( 'NONE',  ( 13.37957753592864663, 7.625938299336016968, -15.70790011242621453 ) ) ;
#4084=CARTESIAN_POINT ( 'NONE',  ( 34.40782828833705054, -13.56718989277036691, -20.98518325316450372 ) ) ;
#4085=CARTESIAN_POINT ( 'NONE',  ( 20.33560388840259137, 1.841519175196629998, -20.14887626749220217 ) ) ;
#4086=CARTESIAN_POINT ( 'NONE',  ( 18.55323344277375242, 5.040171350539718098, -19.22783755317104237 ) ) ;
#4089=CARTESIAN_POINT ( 'NONE',  ( 22.85243615162648112, -7.655412890396200432, -19.01377894019457315 ) ) ;
#4101=CARTESIAN_POINT ( 'NONE',  ( 35.26536834604049631, -19.91213340569504808, -19.23001471935974038 ) ) ;
#4102=CARTESIAN_POINT ( 'NONE',  ( 10.66838568802538845, 9.046021620013140918, -16.41132375377494057 ) ) ;
#4104=CARTESIAN_POINT ( 'NONE',  ( 29.76939623719675510, -8.219725197086590995, -17.35520659559267287 ) ) ;
#4106=CARTESIAN_POINT ( 'NONE',  ( 10.35864927600819740, 16.97212461358170188, -17.91506874352199574 ) ) ;
#4116=CARTESIAN_POINT ( 'NONE',  ( 13.14084490070201738, 8.578467993704791184, -15.89817422466314945 ) ) ;
#4118=CARTESIAN_POINT ( 'NONE',  ( 22.03599841643320190, -0.8527435389730096960, -19.82300248246997398 ) ) ;
#4119=CARTESIAN_POINT ( 'NONE',  ( 17.94761415789183445, 0.5003475314714088684, -19.87472444338139965 ) ) ;
#4125=CARTESIAN_POINT ( 'NONE',  ( 21.40051611374530793, -0.1690565882708310874, -20.18282279970310000 ) ) ;
#4131=CARTESIAN_POINT ( 'NONE',  ( 10.47008273352651564, 16.46107657294071203, -17.33567129194344858 ) ) ;
#4132=CARTESIAN_POINT ( 'NONE',  ( 33.33926371295168423, -12.28475995124076903, -19.67523791759492013 ) ) ;
#4138=CARTESIAN_POINT ( 'NONE',  ( 14.34656430690936624, 9.113120221615268690, -15.03016663717492563 ) ) ;
#4139=CARTESIAN_POINT ( 'NONE',  ( 12.24596961785936777, 9.516471373605908113, -15.33264171117454744 ) ) ;
#4142=CARTESIAN_POINT ( 'NONE',  ( 9.641350810849047548, 17.66889113945805789, -17.95086732675817132 ) ) ;
#4143=CARTESIAN_POINT ( 'NONE',  ( 13.30044262271030142, 7.866402339252101861, -14.49220811360527605 ) ) ;
#4148=CARTESIAN_POINT ( 'NONE',  ( 10.35864953657871190, 16.97212341857210660, -17.91436492910080247 ) ) ;
#4149=CARTESIAN_POINT ( 'NONE',  ( 34.21937970685856101, -11.80343312934236089, -19.83772509046166732 ) ) ;
#4150=CARTESIAN_POINT ( 'NONE',  ( 25.57370974413349884, -0.4222200280313516685, -16.88676729435558599 ) ) ;
#4155=CARTESIAN_POINT ( 'NONE',  ( 28.40444427461093113, -11.06999723682266179, -18.98653349803348078 ) ) ;
#4157=CARTESIAN_POINT ( 'NONE',  ( 27.79171034377997884, -3.119812929724471662, -15.83729198868751276 ) ) ;
#4167=CARTESIAN_POINT ( 'NONE',  ( 12.50396148805030627, 8.572452836447732594, -15.12701763676990119 ) ) ;
#4173=CARTESIAN_POINT ( 'NONE',  ( 9.641350810849047548, 17.66889113945805789, -17.91664992932186351 ) ) ;
#4176=CARTESIAN_POINT ( 'NONE',  ( 17.68287507214707688, 6.939063861736925354, -15.39301800483504934 ) ) ;
#4179=CARTESIAN_POINT ( 'NONE',  ( 23.63863231746517712, -2.790269051896475450, -19.68844555248840678 ) ) ;
#4183=CARTESIAN_POINT ( 'NONE',  ( 12.24523086077475220, 9.516144614896692389, -15.33323053563244898 ) ) ;
#4185=CARTESIAN_POINT ( 'NONE',  ( 35.54859390953724585, -22.18451583373416014, -18.19919658220850778 ) ) ;
#4188=CARTESIAN_POINT ( 'NONE',  ( 25.26806593431409453, -8.821542497490490575, -18.05414547114721557 ) ) ;
#4190=CARTESIAN_POINT ( 'NONE',  ( 25.50636554463319072, -2.203555497659483553, -15.54816553724606187 ) ) ;
#4193=CARTESIAN_POINT ( 'NONE',  ( 18.04976943019953239, 10.79320383120880145, -15.74583687248850161 ) ) ;
#4194=CARTESIAN_POINT ( 'NONE',  ( 27.61097550864939265, -12.05054904645494673, -17.30446993171443637 ) ) ;
#4208=CARTESIAN_POINT ( 'NONE',  ( 9.641350810849047548, 17.66889113945805789, -17.92454625180715766 ) ) ;
#4209=CARTESIAN_POINT ( 'NONE',  ( 24.63339645208565543, -5.721020077635508905, -14.05062826560360278 ) ) ;
#4210=CARTESIAN_POINT ( 'NONE',  ( 18.16551323082808267, 7.152368624112494189, -14.07085781252208712 ) ) ;
#4211=CARTESIAN_POINT ( 'NONE',  ( 32.54894808986480115, -9.611255921941241454, -17.86757894403779900 ) ) ;
#4213=CARTESIAN_POINT ( 'NONE',  ( 11.48249212886396897, 9.228508165798535501, -15.85668214399537845 ) ) ;
#4217=CARTESIAN_POINT ( 'NONE',  ( 10.18658029549746935, 13.84849823568026217, -17.67057034492011525 ) ) ;
#4221=CARTESIAN_POINT ( 'NONE',  ( 12.63667343406881294, 8.631100619704961119, -15.02124387326777111 ) ) ;
#4224=PLANE ( 'NONE',  #18580 ) ;
#4226=CARTESIAN_POINT ( 'NONE',  ( 14.34656430690936624, 9.113120221615268690, -15.03016663717492563 ) ) ;
#4228=CARTESIAN_POINT ( 'NONE',  ( 8.944584683310379702, 16.95159276115599667, -17.93331994345748726 ) ) ;
#4229=CARTESIAN_POINT ( 'NONE',  ( 33.02439791605519304, -11.93986616049457261, -20.58189241239533374 ) ) ;
#4231=CARTESIAN_POINT ( 'NONE',  ( 18.97422388862426601, -0.1098198481195374748, -14.77765307979439058 ) ) ;
#4233=CARTESIAN_POINT ( 'NONE',  ( 16.27660620799252911, 9.202420196601492464, -13.74949690087879439 ) ) ;
#4237=CARTESIAN_POINT ( 'NONE',  ( 20.76230466941008146, -3.840972149463459218, -19.45223659164069474 ) ) ;
#4249=CARTESIAN_POINT ( 'NONE',  ( 34.07550722110926955, -11.19626532300822674, -18.14763417942564061 ) ) ;
#4250=CARTESIAN_POINT ( 'NONE',  ( 10.67622114788023246, 9.011142735252827052, -16.40800301137445416 ) ) ;
#4253=CARTESIAN_POINT ( 'NONE',  ( 26.07968421886551980, -9.001936657367064498, -13.61655714643126913 ) ) ;
#4255=CARTESIAN_POINT ( 'NONE',  ( 11.89844042902047505, 9.910446108148166289, -16.74492965742949835 ) ) ;
#4257=ORIENTED_EDGE ( 'NONE', *, *, #9754, .T. ) ;
#4260=CARTESIAN_POINT ( 'NONE',  ( 12.93612603019711571, 8.763434079353435990, -14.78257486846209545 ) ) ;
#4266=CARTESIAN_POINT ( 'NONE',  ( 13.66828981435543078, 8.811555337407297017, -15.47779131845255307 ) ) ;
#4268=CARTESIAN_POINT ( 'NONE',  ( 23.86816030614728135, 2.079196616232401595, -15.13732202275373062 ) ) ;
#4269=CARTESIAN_POINT ( 'NONE',  ( 22.03599841643320190, -0.8527435389730096960, -19.82300248246997398 ) ) ;
#4271=CARTESIAN_POINT ( 'NONE',  ( 18.54205238286641588, 5.219565156008159512, -20.23764637224795848 ) ) ;
#4275=CARTESIAN_POINT ( 'NONE',  ( 20.51249478307574847, 1.942573248051725709, -13.31196225760961838 ) ) ;
#4287=CARTESIAN_POINT ( 'NONE',  ( 30.87383483136289541, -10.13329766739009052, -15.36655316835725138 ) ) ;
#4288=CARTESIAN_POINT ( 'NONE',  ( 11.05541531668977662, 17.68942339022145305, -17.92279151347708677 ) ) ;
#4289=CARTESIAN_POINT ( 'NONE',  ( 33.57712230886461668, -13.32773824946660923, -19.76201999124979736 ) ) ;
#4295=CARTESIAN_POINT ( 'NONE',  ( 9.641352920869014298, 17.66888146263751125, -17.91030124961049097 ) ) ;
#4301=CARTESIAN_POINT ( 'NONE',  ( 12.86884521499632150, 9.516296226583106588, -16.11496277528728527 ) ) ;
#4302=CARTESIAN_POINT ( 'NONE',  ( 34.91913293194685508, -14.86421081092256280, -20.09741683264573808 ) ) ;
#4303=CARTESIAN_POINT ( 'NONE',  ( 28.09718568327657806, -5.958257988085632562, -17.17874431236187149 ) ) ;
#4307=CARTESIAN_POINT ( 'NONE',  ( 30.07542022419311678, -8.155067017681195907, -14.09159111155252120 ) ) ;
#4309=CARTESIAN_POINT ( 'NONE',  ( 22.63726333831294468, -4.877931240889711972, -12.86144741616201870 ) ) ;
#4315=CARTESIAN_POINT ( 'NONE',  ( 12.37169234869624646, 8.529253869913038244, -15.23127513898213081 ) ) ;
#4322=CARTESIAN_POINT ( 'NONE',  ( 9.641350810849047548, 17.66889113945805789, -17.92279151347709032 ) ) ;
#4324=CARTESIAN_POINT ( 'NONE',  ( 29.99716341122577745, -11.34936846952144585, -14.08097903537201212 ) ) ;
#4328=CARTESIAN_POINT ( 'NONE',  ( 26.85315702054868936, -3.432285194908070380, -17.01323758698984889 ) ) ;
#4333=CARTESIAN_POINT ( 'NONE',  ( 11.05541531668977662, 17.68942339022145305, -23.00000000000000711 ) ) ;
#4335=CARTESIAN_POINT ( 'NONE',  ( 35.16668739017224965, -20.46881214373840763, -20.22602438870426766 ) ) ;
#4337=CARTESIAN_POINT ( 'NONE',  ( 27.44219139316946965, -6.774709612358828181, -18.29578255718776703 ) ) ;
#4339=CARTESIAN_POINT ( 'NONE',  ( 22.40466763571637543, -1.191653471825661059, -14.65485681160645548 ) ) ;
#4343=CARTESIAN_POINT ( 'NONE',  ( 17.78134717446047119, 9.288666448780150020, -20.14505390916605521 ) ) ;
#4344=CARTESIAN_POINT ( 'NONE',  ( 29.03550452591436937, -6.934775515252377787, -18.27713033076000215 ) ) ;
#4345=ORIENTED_EDGE ( 'NONE', *, *, #2685, .F. ) ;
#4356=CARTESIAN_POINT ( 'NONE',  ( 25.25756851182965335, -6.311239348595019116, -19.54001279501058264 ) ) ;
#4357=CARTESIAN_POINT ( 'NONE',  ( 16.37314578033188894, 3.237113944496374351, -18.86778596048347723 ) ) ;
#4359=CARTESIAN_POINT ( 'NONE',  ( 34.14034160798153295, -12.36551392957089135, -20.90432844665832590 ) ) ;
#4360=CARTESIAN_POINT ( 'NONE',  ( 11.82447321682112751, 8.672047275158794477, -15.63808403058127006 ) ) ;
#4366=CARTESIAN_POINT ( 'NONE',  ( 9.668188843004273281, 16.22590751635418371, -17.88494344602179709 ) ) ;
#4370=CARTESIAN_POINT ( 'NONE',  ( 10.33811693838771717, 18.38618951776012267, -23.00000000000000711 ) ) ;
#4380=CARTESIAN_POINT ( 'NONE',  ( 9.631286188771861489, 13.80229212302790920, -16.84020087884530881 ) ) ;
#4381=CARTESIAN_POINT ( 'NONE',  ( 35.54859390953723164, -23.18451583373416014, -14.99999999999999822 ) ) ;
#4382=CARTESIAN_POINT ( 'NONE',  ( 19.77430725462212635, 0.2453161447429414443, -14.21425550582737074 ) ) ;
#4383=CARTESIAN_POINT ( 'NONE',  ( 14.82995595102070752, 5.192148136363496036, -18.54057990209784634 ) ) ;
#4386=CARTESIAN_POINT ( 'NONE',  ( 24.47917272657372223, 1.093256025350008542, -14.89707007128618699 ) ) ;
#4396=CARTESIAN_POINT ( 'NONE',  ( 13.77718166750865869, 8.859676595473324312, -15.39100258941132182 ) ) ;
#4398=CARTESIAN_POINT ( 'NONE',  ( 34.39665924806198660, -11.72086467124742981, -18.77862448471655199 ) ) ;
#4399=CARTESIAN_POINT ( 'NONE',  ( 10.66363677402306287, 9.067800744973538940, -16.41328759676781246 ) ) ;
#4403=CARTESIAN_POINT ( 'NONE',  ( 24.78692427941192733, -9.284778175067517125, -17.23615439686343720 ) ) ;
#4406=CARTESIAN_POINT ( 'NONE',  ( 10.47204342302745417, 16.45208460095963687, -17.33479495221483901 ) ) ;
#4414=CARTESIAN_POINT ( 'NONE',  ( 12.52778158092594474, 8.582979361647906202, -15.10803260229456946 ) ) ;
#4419=CARTESIAN_POINT ( 'NONE',  ( 9.663058643182488083, 16.24943526668553062, -17.89776827055807118 ) ) ;
#4420=CARTESIAN_POINT ( 'NONE',  ( 20.92570677221209507, 1.074447142478794470, -13.03661572703551919 ) ) ;
#4421=CARTESIAN_POINT ( 'NONE',  ( 20.98456156242603754, -1.805893270886621327, -19.41059277335735089 ) ) ;
#4422=CARTESIAN_POINT ( 'NONE',  ( 18.97628335640213493, 0.9430780577607489334, -14.77698032187241850 ) ) ;
#4423=DIRECTION ( 'NONE',  ( -0.06678507476159963041, 0.9947851038922184141, -0.07708664516786083165 ) ) ;
#4425=CARTESIAN_POINT ( 'NONE',  ( 25.45462155318426767, -0.2439708902934435431, -15.99927030562601438 ) ) ;
#4430=CARTESIAN_POINT ( 'NONE',  ( 10.35864918915110877, 16.97212501191939538, -17.91928203681695564 ) ) ;
#4437=CARTESIAN_POINT ( 'NONE',  ( 15.78240017141095741, 4.038647184180326200, -18.77507866864583619 ) ) ;
#4439=CARTESIAN_POINT ( 'NONE',  ( 11.05544237569323762, 17.68929929418238700, -17.89823164173536441 ) ) ;
#4444=CARTESIAN_POINT ( 'NONE',  ( 9.641354186875979337, 17.66887565656821124, -17.90893343548146177 ) ) ;
#4445=CARTESIAN_POINT ( 'NONE',  ( 12.75684812230466925, 7.626178201396932366, -14.92546252573342258 ) ) ;
#4452=CARTESIAN_POINT ( 'NONE',  ( 10.35864918915110877, 16.97212501191939538, -17.97192418671891190 ) ) ;
#4455=CARTESIAN_POINT ( 'NONE',  ( 33.49783966318349115, -10.45910432307822902, -18.51641766868578287 ) ) ;
#4457=CARTESIAN_POINT ( 'NONE',  ( 26.84970692451943819, -5.812874930055231815, -14.04107299160273037 ) ) ;
#4461=CARTESIAN_POINT ( 'NONE',  ( 14.77364001808635585, 4.929448384924057791, -16.82930887520970131 ) ) ;
#4462=CARTESIAN_POINT ( 'NONE',  ( 22.71651454236177514, -3.376241010138071541, -20.62701743264632270 ) ) ;
#4467=ORIENTED_EDGE ( 'NONE', *, *, #3821, .F. ) ;
#4473=CARTESIAN_POINT ( 'NONE',  ( 10.72001338896670397, 16.63476371493014128, -15.95452473000899118 ) ) ;
#4474=CARTESIAN_POINT ( 'NONE',  ( 26.95082352492110189, -12.40836276091286194, -17.97502949936508898 ) ) ;
#4478=CARTESIAN_POINT ( 'NONE',  ( 9.913797604922770290, 16.41941541294738727, -16.50570979788118464 ) ) ;
#4479=CARTESIAN_POINT ( 'NONE',  ( 15.22094575638775282, 5.866722348926807662, -16.67377462076821715 ) ) ;
#4486=CARTESIAN_POINT ( 'NONE',  ( 12.35402573141577598, 9.564223303342972216, -15.24651908135525957 ) ) ;
#4488=CARTESIAN_POINT ( 'NONE',  ( 35.02155038278115740, -19.81678845073966500, -20.19863594638463411 ) ) ;
#4492=CARTESIAN_POINT ( 'NONE',  ( 22.98313442454129429, 1.505266882216666158, -15.27805348665062546 ) ) ;
#4496=CARTESIAN_POINT ( 'NONE',  ( 28.19717681610909210, -11.01075670644066662, -19.96981485020118541 ) ) ;
#4497=CARTESIAN_POINT ( 'NONE',  ( 25.16264305761801268, -10.69278474016982727, -17.18274900023375906 ) ) ;
#4508=CARTESIAN_POINT ( 'NONE',  ( 19.73758642798775753, -1.564653675968832314, -13.27997001701493041 ) ) ;
#4509=CARTESIAN_POINT ( 'NONE',  ( 19.14470263920462401, 1.819183656627200829, -19.33730474122706866 ) ) ;
#4510=CARTESIAN_POINT ( 'NONE',  ( 32.74140904187309786, -11.17293925747269867, -20.20304766317806866 ) ) ;
#4512=CARTESIAN_POINT ( 'NONE',  ( 11.69419402147360110, 8.800013620902292999, -15.72776802682527730 ) ) ;
#4515=CARTESIAN_POINT ( 'NONE',  ( 16.75072914628186282, 8.771658487634226731, -19.67538163746542779 ) ) ;
#4519=CARTESIAN_POINT ( 'NONE',  ( 12.50481220565295004, 8.572828783776230921, -15.12633959982445653 ) ) ;
#4524=CARTESIAN_POINT ( 'NONE',  ( 17.85084670134855145, 5.929878015568476712, -20.08862479909851828 ) ) ;
#4527=CARTESIAN_POINT ( 'NONE',  ( 9.113084692838755885, 16.17883023870341930, -17.05449542622726966 ) ) ;
#4528=CARTESIAN_POINT ( 'NONE',  ( 35.54859390953724585, -23.18451583373416014, -17.99055332684694974 ) ) ;
#4529=CARTESIAN_POINT ( 'NONE',  ( 20.44834407054411685, 8.573499863981592028, -15.78670165415130100 ) ) ;
#4530=CARTESIAN_POINT ( 'NONE',  ( 27.39958189869922123, -12.72506959635235368, -13.65552181841346524 ) ) ;
#4533=CARTESIAN_POINT ( 'NONE',  ( 21.02038916656773182, -4.531596735700774481, -13.49074533895851147 ) ) ;
#4544=CARTESIAN_POINT ( 'NONE',  ( 36.41702210941816986, -20.59343343131470050, -19.35259392719279603 ) ) ;
#4545=CARTESIAN_POINT ( 'NONE',  ( 12.62682997171803123, 7.576475742438638861, -15.02849783152220908 ) ) ;
#4550=CARTESIAN_POINT ( 'NONE',  ( 10.49225533350670858, 16.35939020308235925, -17.32643665990597981 ) ) ;
#4557=VERTEX_POINT ( 'NONE', #15510 ) ;
#4560=CARTESIAN_POINT ( 'NONE',  ( 9.668122305056073174, 16.22621266786625327, -17.88497096177859191 ) ) ;
#4561=CARTESIAN_POINT ( 'NONE',  ( 22.18457322443145330, -2.050108300791262828, -13.94172724511641448 ) ) ;
#4562=CARTESIAN_POINT ( 'NONE',  ( 21.24065112674864864, -1.570060580458334965, -19.57950003236798864 ) ) ;
#4564=CARTESIAN_POINT ( 'NONE',  ( 16.05281274719596496, 2.901206577426825639, -17.92093306952238407 ) ) ;
#4568=CARTESIAN_POINT ( 'NONE',  ( 27.51942754507220812, -5.605608590038333006, -14.64806962472005658 ) ) ;
#4574=ADVANCED_FACE ( 'NONE', ( #25434 ), #21946, .T. ) ;
#4583=CARTESIAN_POINT ( 'NONE',  ( 11.15915788317279578, 9.388133443793682531, -17.26837529997955301 ) ) ;
#4586=CARTESIAN_POINT ( 'NONE',  ( 19.52227536296714305, 7.868296793410291201, -18.00468392081665669 ) ) ;
#4587=CARTESIAN_POINT ( 'NONE',  ( 11.27564905058850719, 16.67940341329043363, -16.78475148866115774 ) ) ;
#4588=CARTESIAN_POINT ( 'NONE',  ( 34.93238815599637803, -19.41622979634004764, -20.17168434421570922 ) ) ;
#4591=CARTESIAN_POINT ( 'NONE',  ( 9.641350810849047548, 17.66889113945805789, -17.94384837343789485 ) ) ;
#4593=CARTESIAN_POINT ( 'NONE',  ( 9.641350810849047548, 17.66889113945805789, -17.95086732675817132 ) ) ;
#4599=CARTESIAN_POINT ( 'NONE',  ( 10.41412541532089620, 16.71770396712979689, -17.42473314453425814 ) ) ;
#4601=CARTESIAN_POINT ( 'NONE',  ( 34.39307579391925174, -12.50091474996580487, -19.93840237985029162 ) ) ;
#4602=CARTESIAN_POINT ( 'NONE',  ( 23.77086030874127687, -7.150112426529108944, -14.59934731766091431 ) ) ;
#4607=CARTESIAN_POINT ( 'NONE',  ( 19.16431125762126442, 9.782083453288988650, -17.54400000489614087 ) ) ;
#4608=CARTESIAN_POINT ( 'NONE',  ( 27.49606495187617128, -9.167791027049197794, -14.03786016821673677 ) ) ;
#4618=CARTESIAN_POINT ( 'NONE',  ( 10.34111691064986438, 18.37243126255838988, -17.67295385331717483 ) ) ;
#4622=CARTESIAN_POINT ( 'NONE',  ( 11.45256130090833935, 9.362448956408465861, -15.86931324879919991 ) ) ;
#4623=CARTESIAN_POINT ( 'NONE',  ( 14.03260640687251204, 7.914523597318124715, -15.18742456358547521 ) ) ;
#4626=CARTESIAN_POINT ( 'NONE',  ( 27.76312469413510442, -10.32446017237915648, -18.80420148706337358 ) ) ;
#4630=CARTESIAN_POINT ( 'NONE',  ( 11.28624536866114347, 16.63080734789289750, -16.78036754607827064 ) ) ;
#4633=CARTESIAN_POINT ( 'NONE',  ( 33.37634376253905089, -12.42895282922877342, -19.69946502924221932 ) ) ;
#4637=CARTESIAN_POINT ( 'NONE',  ( 26.42637521690935998, -6.951663299830703302, -19.91275981816901464 ) ) ;
#4641=CARTESIAN_POINT ( 'NONE',  ( 19.54522145393098498, 6.247755356217567169, -19.64858106251988801 ) ) ;
#4642=CARTESIAN_POINT ( 'NONE',  ( 25.61980203353413543, -10.24193911033393256, -18.22380977611897990 ) ) ;
#4650=CARTESIAN_POINT ( 'NONE',  ( 9.915538251416846194, 16.41143258624473233, -16.50493629029764264 ) ) ;
#4651=CARTESIAN_POINT ( 'NONE',  ( 27.35978538551520245, -3.059420540688277956, -14.62525642202852971 ) ) ;
#4652=CARTESIAN_POINT ( 'NONE',  ( 22.75707610144304383, -3.504958924507949991, -13.40925247317622571 ) ) ;
#4653=CARTESIAN_POINT ( 'NONE',  ( 33.35113679096266992, -13.31250502539155534, -20.73603153870848104 ) ) ;
#4658=CARTESIAN_POINT ( 'NONE',  ( 14.79111372287554715, 6.954724682967856175, -19.27298399620107361 ) ) ;
#4660=CARTESIAN_POINT ( 'NONE',  ( 10.72208662246453770, 16.62525560183325624, -15.95366392025685620 ) ) ;
#4669=CARTESIAN_POINT ( 'NONE',  ( 19.91209246711783010, 5.411768277715644615, -14.29674560697521457 ) ) ;
#4672=CARTESIAN_POINT ( 'NONE',  ( 35.51409509342218485, -23.02953092745895347, -19.29936871477319826 ) ) ;
#4673=CARTESIAN_POINT ( 'NONE',  ( 24.34695368780276681, -2.542362794815061999, -14.38654857168906886 ) ) ;
#4675=CARTESIAN_POINT ( 'NONE',  ( 15.13914318552241056, 5.040073780016904870, -15.86576734333453764 ) ) ;
#4676=CARTESIAN_POINT ( 'NONE',  ( 23.88957251509086888, -3.236156964677408876, -12.29669325917074829 ) ) ;
#4684=CARTESIAN_POINT ( 'NONE',  ( 36.54006368622684420, -21.14619405898047688, -18.64381572867062076 ) ) ;
#4686=CARTESIAN_POINT ( 'NONE',  ( 9.641350944112486943, 17.66889052829492002, -17.91441860517739215 ) ) ;
#4690=CARTESIAN_POINT ( 'NONE',  ( 10.47452605456472696, 16.44069893626776491, -17.33376834041267145 ) ) ;
#4703=CARTESIAN_POINT ( 'NONE',  ( 9.667620158929956631, 16.22851557400931455, -17.88520075955172572 ) ) ;
#4704=CARTESIAN_POINT ( 'NONE',  ( 19.89307947303188229, -2.966738011908462092, -16.73278295482091949 ) ) ;
#4705=CARTESIAN_POINT ( 'NONE',  ( 20.12919692000023986, -2.949910412001375715, -15.69023992059449846 ) ) ;
#4707=CARTESIAN_POINT ( 'NONE',  ( 19.54522145393098498, 6.247755356217567169, -19.64858106251988801 ) ) ;
#4713=CARTESIAN_POINT ( 'NONE',  ( 26.31132954256896639, -3.159408024760113509, -14.81636702655834803 ) ) ;
#4724=CARTESIAN_POINT ( 'NONE',  ( 11.18347232286468440, 9.276624323996792043, -17.25832042385608389 ) ) ;
#4728=CARTESIAN_POINT ( 'NONE',  ( 19.91209246711783010, 5.411768277715644615, -14.29674560697521457 ) ) ;
#4729=CARTESIAN_POINT ( 'NONE',  ( 11.29637638519941589, 16.58434521464408817, -16.77617801436024081 ) ) ;
#4735=CARTESIAN_POINT ( 'NONE',  ( 9.917205744531459644, 16.40378525026516243, -16.50423678068149869 ) ) ;
#4738=CARTESIAN_POINT ( 'NONE',  ( 9.917965570771830386, 16.40030059027150600, -16.50392256580263606 ) ) ;
#4745=CARTESIAN_POINT ( 'NONE',  ( 10.47195275365909595, 16.45250042224058618, -17.33483252618548676 ) ) ;
#4747=CARTESIAN_POINT ( 'NONE',  ( 36.53271160917758209, -22.11316507130252873, -18.90714217169671230 ) ) ;
#4748=CARTESIAN_POINT ( 'NONE',  ( 23.29338531092689735, -7.078548041224526521, -17.51562821661096336 ) ) ;
#4751=ORIENTED_EDGE ( 'NONE', *, *, #9754, .F. ) ;
#4754=CARTESIAN_POINT ( 'NONE',  ( 19.52759782329482263, 6.073010510103808990, -18.47256557099433394 ) ) ;
#4755=CARTESIAN_POINT ( 'NONE',  ( 25.90061519764796572, -9.523157571424881951, -17.57609359838447816 ) ) ;
#4764=CARTESIAN_POINT ( 'NONE',  ( 10.72132679622416696, 16.62874026182691267, -15.95397813513572061 ) ) ;
#4769=CARTESIAN_POINT ( 'NONE',  ( 9.916637298967875935, 16.40639221407973380, -16.50447193873893781 ) ) ;
#4774=CARTESIAN_POINT ( 'NONE',  ( 27.20859382114707614, -12.49599901988731077, -15.99530080614381511 ) ) ;
#4779=CARTESIAN_POINT ( 'NONE',  ( 24.62590367393082502, -9.567571807129121808, -15.85044010117769098 ) ) ;
#4783=CARTESIAN_POINT ( 'NONE',  ( 11.05542614047498873, 17.68937375096277265, -17.90480922774079175 ) ) ;
#4785=CARTESIAN_POINT ( 'NONE',  ( 33.29128644620831778, -11.81988703332123691, -18.18190324972602667 ) ) ;
#4786=CARTESIAN_POINT ( 'NONE',  ( 17.17204249742301059, 10.23148044644768362, -15.96021614775051667 ) ) ;
#4788=CARTESIAN_POINT ( 'NONE',  ( 27.97271982581976957, -5.335442005784750918, -18.83880583778296725 ) ) ;
#4791=CARTESIAN_POINT ( 'NONE',  ( 22.84118038848623655, 1.850029439873439152, -18.07216660426987431 ) ) ;
#4792=CARTESIAN_POINT ( 'NONE',  ( 18.71812633715165575, 6.658065805436550910, -18.41436643113302551 ) ) ;
#4801=CARTESIAN_POINT ( 'NONE',  ( 9.916118674515717046, 16.40877069192658055, -16.50468880802031890 ) ) ;
#4803=CARTESIAN_POINT ( 'NONE',  ( 27.85231147893869874, -3.451530096863186792, -17.11803778117090857 ) ) ;
#4804=CARTESIAN_POINT ( 'NONE',  ( 18.75392633456350922, 0.8452085672475394551, -14.97946080469353447 ) ) ;
#4805=CARTESIAN_POINT ( 'NONE',  ( 30.78206665311622459, -10.11802168058175511, -15.10569088962643036 ) ) ;
#4807=CARTESIAN_POINT ( 'NONE',  ( 36.54859390953723874, -22.18451583373416014, -15.00000000000000000 ) ) ;
#4810=CARTESIAN_POINT ( 'NONE',  ( 14.17177033308128031, 6.273687421093853800, -17.36430109743762173 ) ) ;
#4814=CARTESIAN_POINT ( 'NONE',  ( 10.48326151898216452, 17.72053796952357985, -16.40639007392780258 ) ) ;
#4818=CARTESIAN_POINT ( 'NONE',  ( 18.55171814111300321, 6.637122934506423988, -19.73184648383247364 ) ) ;
#4820=CARTESIAN_POINT ( 'NONE',  ( 30.38377115645388571, -7.011354780429720712, -16.65419678813778503 ) ) ;
#4822=CARTESIAN_POINT ( 'NONE',  ( 33.24414211882076842, -12.83183464011245967, -20.70368961610576264 ) ) ;
#4825=CARTESIAN_POINT ( 'NONE',  ( 20.97270766892557603, 0.7925772802953747753, -14.00178974354743033 ) ) ;
#4826=CARTESIAN_POINT ( 'NONE',  ( 20.59924605810746101, 4.422246688411098248, -17.72709849028201035 ) ) ;
#4828=CARTESIAN_POINT ( 'NONE',  ( 26.40217035250003974, -9.511505991202637844, -18.98702918838447573 ) ) ;
#4837=CARTESIAN_POINT ( 'NONE',  ( 36.29797175594614345, -20.05860325589622661, -19.47188034632657150 ) ) ;
#4839=CARTESIAN_POINT ( 'NONE',  ( 12.75639466810640776, 7.625977817552541005, -14.92582393630036108 ) ) ;
#4843=CARTESIAN_POINT ( 'NONE',  ( 10.47262648896379922, 16.44941058625191133, -17.33455387760982447 ) ) ;
#4852=CARTESIAN_POINT ( 'NONE',  ( 9.669898452045105230, 16.21806703136846295, -17.88423646254436861 ) ) ;
#4854=CARTESIAN_POINT ( 'NONE',  ( 25.86774690167791135, -3.337865513817628749, -16.68124922160397006 ) ) ;
#4855=CARTESIAN_POINT ( 'NONE',  ( 16.37314578033188894, 3.237113944496374351, -18.86778596048347723 ) ) ;
#4861=CARTESIAN_POINT ( 'NONE',  ( 25.97256211245905533, -8.171536508395311316, -18.54953510021574559 ) ) ;
#4871=CARTESIAN_POINT ( 'NONE',  ( 10.47151541139924547, 16.45450612959241354, -17.33501744001014444 ) ) ;
#4873=CARTESIAN_POINT ( 'NONE',  ( 35.54859390954303677, -22.18451583373416014, -15.55638201429745848 ) ) ;
#4874=CARTESIAN_POINT ( 'NONE',  ( 33.57712230886461668, -13.32773824946660923, -19.76201999124979736 ) ) ;
#4876=CARTESIAN_POINT ( 'NONE',  ( 13.65148492087865151, 7.746099194123166498, -15.49118511517110619 ) ) ;
#4879=CARTESIAN_POINT ( 'NONE',  ( 19.50856600871340873, -1.908691058934758100, -18.90332006808282728 ) ) ;
#4880=CARTESIAN_POINT ( 'NONE',  ( 11.27378865171844602, 16.68793543965420767, -16.78556983912737621 ) ) ;
#4885=CARTESIAN_POINT ( 'NONE',  ( 9.649959050778257108, 17.62941265384766254, -17.56860460898032628 ) ) ;
#4888=CARTESIAN_POINT ( 'NONE',  ( 9.776119957569173735, 17.05082265352876547, -16.72288386497739765 ) ) ;
#4894=CARTESIAN_POINT ( 'NONE',  ( 11.12037835888041393, 13.47873794165536410, -17.06668569338069830 ) ) ;
#4896=CARTESIAN_POINT ( 'NONE',  ( 33.94449656094377588, -11.59990251341361933, -20.77871222707083376 ) ) ;
#4897=CARTESIAN_POINT ( 'NONE',  ( 15.30534275580653869, 10.60631812597827839, -15.20037037882373987 ) ) ;
#4898=CARTESIAN_POINT ( 'NONE',  ( 24.81358459371387326, -5.676498915796258871, -18.90393244824272756 ) ) ;
#4901=CARTESIAN_POINT ( 'NONE',  ( 34.36632712588347260, -12.38074715364594347, -19.93031689919964222 ) ) ;
#4903=CARTESIAN_POINT ( 'NONE',  ( 15.96850636225579656, 5.405031054132949819, -14.95518105802344344 ) ) ;
#4905=CARTESIAN_POINT ( 'NONE',  ( 14.34656430690936624, 9.113120221615268690, -15.03016663717492563 ) ) ;
#4916=CARTESIAN_POINT ( 'NONE',  ( 10.74108227847380448, 16.53813910199176007, -15.94580854828543437 ) ) ;
#4923=CARTESIAN_POINT ( 'NONE',  ( 9.915973561396301150, 16.40943619918981256, -16.50475030878699556 ) ) ;
#4925=CARTESIAN_POINT ( 'NONE',  ( 9.670405002872021427, 16.21574392470601467, -17.88402698595844598 ) ) ;
#4926=CARTESIAN_POINT ( 'NONE',  ( 18.89276694006714052, 5.271756288042509730, -14.92826338805148190 ) ) ;
#4929=CARTESIAN_POINT ( 'NONE',  ( 27.01132674553606350, -11.00696853675122711, -18.49859303458091730 ) ) ;
#4932=CARTESIAN_POINT ( 'NONE',  ( 11.26126983089308098, 16.74534834773793790, -16.79273533431442900 ) ) ;
#4934=CARTESIAN_POINT ( 'NONE',  ( 35.34747194004189907, -20.28098136206135749, -19.25482875754748946 ) ) ;
#4937=CARTESIAN_POINT ( 'NONE',  ( 26.79503139269368006, -8.611318205148688065, -11.94858980718629304 ) ) ;
#4941=CARTESIAN_POINT ( 'NONE',  ( 18.23802153489769751, 0.9697156596711644649, -18.35043786425562828 ) ) ;
#4942=CARTESIAN_POINT ( 'NONE',  ( 16.58324305800299925, 4.586402732284541095, -18.38077023430394163 ) ) ;
#4956=CARTESIAN_POINT ( 'NONE',  ( 9.916953853453376766, 16.40494045485788632, -16.50434094533541085 ) ) ;
#4957=CARTESIAN_POINT ( 'NONE',  ( 25.48002462322397577, -3.608900787083736184, -12.74538502395823691 ) ) ;
#4958=CARTESIAN_POINT ( 'NONE',  ( 24.47846259200217034, 0.2319951948203725633, -15.89054235832688278 ) ) ;
#4959=CARTESIAN_POINT ( 'NONE',  ( 36.45689639539443050, -22.77256747621617095, -19.95163700058902734 ) ) ;
#4962=CARTESIAN_POINT ( 'NONE',  ( 12.93612603019711571, 8.763434079353435990, -14.78257486846209545 ) ) ;
#4965=CARTESIAN_POINT ( 'NONE',  ( 17.69365662292968366, 10.27476822432933545, -17.01437286930526227 ) ) ;
#4967=CARTESIAN_POINT ( 'NONE',  ( 10.70471194873291410, 16.70493807032227451, -15.96226385378574264 ) ) ;
#4971=CARTESIAN_POINT ( 'NONE',  ( 16.79143122783437292, 7.330551994622505063, -14.54187356113185103 ) ) ;
#4973=CARTESIAN_POINT ( 'NONE',  ( 13.62270618888621776, 10.12723052195839024, -14.35540206260209573 ) ) ;
#4975=CARTESIAN_POINT ( 'NONE',  ( 33.38708106686501509, -12.47399286361455850, -19.70456970583452616 ) ) ;
#4976=CARTESIAN_POINT ( 'NONE',  ( 23.02024704684396283, -2.230829994151436679, -18.49515006079944612 ) ) ;
#4978=CARTESIAN_POINT ( 'NONE',  ( 21.97327598498023704, 3.176719406474355800, -15.71098195781089046 ) ) ;
#4979=CARTESIAN_POINT ( 'NONE',  ( 28.61171173311277016, -11.12923776720465874, -18.00325214586577971 ) ) ;
#4990=CARTESIAN_POINT ( 'NONE',  ( 34.47095863366522650, -11.93304594944324926, -18.87179757263150037 ) ) ;
#4991=CARTESIAN_POINT ( 'NONE',  ( 9.641352920869014298, 17.66888146263751125, -17.91030124961049097 ) ) ;
#4996=CARTESIAN_POINT ( 'NONE',  ( 12.67163634847678644, 8.538173360731750705, -16.25940050138558135 ) ) ;
#5009=CARTESIAN_POINT ( 'NONE',  ( 9.670405002872021427, 16.21574392470601467, -17.88402698595844598 ) ) ;
#5011=CARTESIAN_POINT ( 'NONE',  ( 25.47886751038978304, -3.221426504603704277, -15.37741025701318698 ) ) ;
#5012=CARTESIAN_POINT ( 'NONE',  ( 19.47299019774181161, -1.479546722229555744, -17.51644493673600067 ) ) ;
#5016=CARTESIAN_POINT ( 'NONE',  ( 22.09544204423535874, -4.864148257255451746, -14.35781331922719772 ) ) ;
#5022=CARTESIAN_POINT ( 'NONE',  ( 10.63408956504272140, 15.70892033759881734, -17.26778321585235787 ) ) ;
#5024=CARTESIAN_POINT ( 'NONE',  ( 34.39741479528305490, -17.01287786994462792, -20.00997473120332515 ) ) ;
#5026=CARTESIAN_POINT ( 'NONE',  ( 8.944586743066221146, 16.95158331485313852, -17.91159992548655566 ) ) ;
#5029=CARTESIAN_POINT ( 'NONE',  ( 17.18819971663578272, 0.8441372818425427749, -18.45219435416397502 ) ) ;
#5030=CARTESIAN_POINT ( 'NONE',  ( 11.34095285796786712, 16.37991182834946713, -16.75774407480071559 ) ) ;
#5035=CARTESIAN_POINT ( 'NONE',  ( 9.641350810849047548, 17.66889113945805789, -17.93331994345748370 ) ) ;
#5037=CARTESIAN_POINT ( 'NONE',  ( 9.918725397012197575, 16.39681593027784956, -16.50360835092378409 ) ) ;
#5042=CARTESIAN_POINT ( 'NONE',  ( 10.48820292689142519, 16.37797505638186735, -17.32811247259324716 ) ) ;
#5045=CARTESIAN_POINT ( 'NONE',  ( 33.72790161547175103, -10.96501189107364738, -20.51660325596433765 ) ) ;
#5046=CARTESIAN_POINT ( 'NONE',  ( 26.87449084144840938, -11.88902188497427481, -13.49525739704605343 ) ) ;
#5047=CARTESIAN_POINT ( 'NONE',  ( 13.75440121443578079, 9.907639265912045801, -15.40915901261088905 ) ) ;
#5052=CARTESIAN_POINT ( 'NONE',  ( 34.39307579391925174, -12.50091474996580487, -19.93840237985029162 ) ) ;
#5054=CARTESIAN_POINT ( 'NONE',  ( 13.40933447586352578, 7.914523597318124715, -14.40541938456405369 ) ) ;
#5055=CARTESIAN_POINT ( 'NONE',  ( 29.11570147443254797, -8.594497869595446815, -15.09001435577217087 ) ) ;
#5061=( BOUNDED_SURFACE ( )  B_SPLINE_SURFACE ( 3, 3, ( 
 ( #25118, #10913, #1782, #29608, #4062, #6200, #15647, #13356, #11067, #4208, #13505, #11503, #83, #23577, #7253, #2833, #27893, #12118, #7548, #18695, #2673, #20818, #7408, #18539, #16709, #9673, #18995, #26179, #28353, #14246, #6955, #21434, #25719, #23272, #16243, #28500, #9515, #28198, #16852, #13796, #11959, #26030, #14094, #23122, #5104, #18837, #9364, #25555, #28040, #19142, #7096, #16396, #25876, #20974, #4650, #16553, #4801, #14394, #545, #11660, #23428, #23736, #2385, #4956, #13942, #2231, #2541, #30202, #11811, #21126, #9827, #9212, #238, #21275, #387, #24331, #10275, #3425, #10422, #24040, #14698, #21880, #12716, #17598, #8138, #3139, #10124, #26794, #5866, #15148, #14547, #12413, #24479, #29099, #12562, #17297, #17445, #19433, #10579, #3577, #12267, #19287, #12866, #29255, #28807, #14998, #21586, #22179, #9972, #1290, #1142, #19731, #5260, #19886, #5717, #28643, #8289, #17154, #21730, #7694, #23895, #992, #19584, #2992, #684, #22038, #17006, #5563, #26330, #5413, #28953, #833, #7845, #26483, #14843, #24185, #3287, #26636, #7989, #29418, #11028, #29565, #18195, #4315, #24786, #27263, #1898, #6163, #20332, #1441, #2047, #10875, #11326, #15457, #13171, #15903, #9023, #17883, #8730, #27101, #15754, #1741, #25079, #11178, #3876, #22497, #13319, #4167, #26953, #29874, #1598, #20185, #27555, #6608, #25231, #6010, #8586, #13615, #20486, #4023, #18045, #8882, #6313, #20633, #22947, #3726 ),
 ( #15608, #30013, #15297, #22789, #6462, #29721, #24629, #24941, #10734, #13023, #22643, #13463, #22339, #20046, #8439, #17741, #27411, #18501, #25526, #7369, #20782, #23389, #30168, #18659, #11464, #48, #503, #2642, #16666, #23692, #2505, #23540, #16051, #4618, #28161, #11773, #25988, #9176, #18802, #27856, #13908, #14058, #21091, #11920, #6917, #23235, #28311, #21238, #5065, #353, #16210, #9638, #28004, #25837, #18956, #14355, #4473, #2350, #7063, #25678, #11623, #16356, #2797, #12079, #7216, #4764, #21396, #18348, #23092, #20936, #2195, #16509, #9329, #27704, #200, #9479, #4916, #14211, #6761, #25379, #13763, #7659, #10083, #29058, #15111, #19548, #22000, #28918, #8096, #17408, #26443, #10387, #16965, #12230, #5377, #24442, #5219, #21545, #26754, #649, #26290, #14660, #14959, #10236, #24007, #9934, #19104, #28459, #7509, #24292, #5823, #3387, #7952, #16809, #5677, #19246, #14805, #19395, #3537, #792, #28602, #9786, #12829, #3102, #17261, #24145, #28766, #26590, #5524, #12377, #22143, #12680, #26140, #3249, #1108, #21689, #7810, #17116, #12524, #21842, #19696, #14511, #948, #23853, #2953, #20008, #1706, #29376, #29531, #10841, #15570, #6432, #24904, #20297, #3839, #22299, #26911, #12985, #15724, #11149, #25052, #27380, #18011, #4139, #15868, #10989, #13431, #29685, #20451, #29844, #17851, #1870, #8400, #3684, #27066, #25198, #5973, #1405, #8849, #10698, #17705, #6121, #22758, #8700, #15419, #24753 ),
 ( #18164, #29211, #27525, #13131, #6277, #20149, #6580, #22463, #1561, #1249, #4288, #8548, #13590, #3990, #27227, #10536, #13289, #22607, #19844, #8249, #17560, #15262, #24593, #23062, #27821, #6888, #25346, #4439, #16473, #9601, #16177, #11435, #2017, #20745, #23352, #30134, #20900, #2316, #7031, #28122, #16322, #11741, #25498, #13735, #18311, #2161, #7181, #2612, #25800, #18769, #9444, #4880, #7332, #9141, #2466, #18469, #4587, #18623, #25639, #14176, #13877, #23199, #11887, #23503, #21202, #317, #11586, #18922, #11, #164, #28275, #16630, #8993, #16021, #9298, #27971, #4729, #14023, #25950, #5030, #21059, #22914, #11296, #20600, #27667, #29983, #6730, #14769, #5341, #17230, #12194, #7772, #19072, #28425, #26719, #21652, #21964, #21510, #14626, #3359, #19660, #23974, #7477, #26257, #14321, #28888, #12645, #29025, #19362, #19515, #12045, #617, #24112, #17084, #1078, #16780, #10356, #8063, #19211, #3211, #21359, #7920, #26105, #26557, #10201, #5644, #23657, #14922, #12489, #5183, #17374, #3064, #23816, #14478, #2759, #10048, #28723, #464, #9751, #21812, #24262, #12340, #2914, #9901, #26407, #28568, #7621, #16926, #751, #5487, #910, #17822, #12949, #8214, #20120, #8370, #27346, #13400, #3653, #6090, #10956, #15229, #29500, #10500, #11115, #19972, #20418, #24564, #22262, #25021, #18126, #27033, #27192, #5944, #24871, #10812, #3960, #20266, #1371, #10663, #22426, #13258, #5791, #8669, #29343, #17677 ),
 ( #15386, #15073, #22728, #26880, #6245, #8520, #24719, #15540, #1529, #3806, #29809, #22577, #8818, #1677, #29653, #13097, #17974, #6401, #17525, #15692, #4106, #1832, #24412, #3507, #12800, #22115, #1217, #19812, #29178, #6849, #11546, #2427, #20862, #16284, #30097, #18275, #22878, #8959, #16141, #30245, #11704, #9256, #25595, #9106, #27633, #1983, #6698, #21021, #7139, #126, #23314, #13985, #9410, #11853, #15987, #27936, #25314, #13704, #23162, #18584, #18736, #4406, #23029, #16438, #28082, #25762, #4843, #2131, #14141, #27786, #4690, #23470, #2580, #13551, #20567, #25459, #4550, #11401, #13839, #21167, #277, #6995, #2279, #9561, #27492, #11264, #29950, #20709, #6544, #18435, #15833, #25164, #4255, #23619, #2718, #1040, #26223, #26524, #16749, #19181, #7888, #24230, #28686, #879, #7738, #17197, #5607, #5303, #19482, #26072, #21318, #14441, #3329, #14286, #427, #14884, #9710, #5147, #23780, #24080, #19328, #2874, #19035, #28238, #7292, #16594, #3181, #12608, #12453, #17049, #25919, #14736, #28392, #23938, #28537, #21925, #9868, #7446, #18881, #4996, #12159, #26375, #3029, #7587, #5454, #14589, #21473, #12005, #21779, #583, #12307, #10166, #16891, #21623, #719, #10013, #28850, #3923, #27309, #3620, #29142, #19626, #8179, #10781, #17491, #8338, #29619, #24375, #8633, #4071, #15194, #20090, #17338, #13220, #15041, #22544, #6209, #15501, #22689, #24832, #29466, #3468, #17934, #22226, #19771, #12761 ),
 ( #1642, #10626, #13365, #10922, #15343, #5912, #22082, #26843, #15657, #24529, #12911, #22387, #1336, #1185, #24681, #19935, #20230, #6363, #29304, #17640, #24989, #26997, #3771, #10465, #10318, #6058, #28993, #13064, #1493, #8029, #26684, #8485, #17788, #27146, #5759, #11371, #6809, #23546, #22844, #13515, #22991, #25846, #2804, #11925, #1945, #8926, #359, #9644, #18963, #1790, #11229, #28319, #21246, #2094, #27750, #7378, #18241, #14365, #16673, #8779, #23699, #6658, #5072, #20531, #4366, #20676, #29917, #2650, #25995, #11079, #4925, #9071, #20379, #27598, #25126, #29769, #15950, #18093, #27458, #25277, #6508, #15800, #13667, #30059, #18397, #4217, #16519, #14217, #15296, #29564, #2309, #6461, #15751, #25077, #4583, #4724, #1440, #20331, #29417, #6162, #15607, #29251, #8288, #17597, #13872, #27965, #23195, #29720, #26952, #11582, #20044, #24940, #8585, #25635, #10874, #8438, #19885, #7027, #10732, #8729, #4020, #20183, #18044, #6312, #15456, #14017, #27410, #23348, #13318, #20896, #17739, #24785, #3875, #22337, #27100, #7, #16317, #13170, #22495, #6009, #1597, #9293, #17882, #27262, #22641, #1740, #18618, #11027, #2462, #24628, #3724, #13021, #7177, #21355, #23971, #28564, #7618, #16922, #26252, #26405, #23498, #12191, #21195, #28272, #7474, #26101, #5338, #11883, #18918, #21649, #14623, #747, #3060, #313, #12335, #12040, #19208, #10045, #19358, #28118, #4876, #460, #19066, #9596, #9747, #28720 ),
 ( #14172, #25795, #21507, #2753, #7767, #7326, #5180, #16469, #2608, #24108, #28420, #17081, #16626, #16777, #5484, #14767, #611, #11737, #9898, #21054, #160, #14472, #9438, #25945, #5026, #14317, #18764, #23652, #23814, #2911, #14919, #10353, #19658, #8367, #3650, #29023, #24259, #6084, #12946, #1215, #29497, #6241, #7917, #5639, #17228, #22259, #24410, #15382, #1073, #26877, #26555, #3357, #15537, #10498, #10808, #8060, #3505, #22421, #8517, #1367, #24715, #10658, #1526, #20117, #19809, #3803, #17369, #12643, #26716, #17816, #28885, #21962, #27189, #5789, #15071, #12795, #17673, #19969, #22113, #29172, #12486, #21810, #908, #27030, #3208, #13094, #29340, #10199, #19511, #8211, #17521, #5941, #15225, #24558, #25016, #24868, #2273, #15687, #25310, #29945, #15829, #4399, #11260, #20414, #9252, #23023, #18581, #8955, #9102, #4102, #29805, #8814, #27342, #6397, #18430, #11542, #18121, #13396, #3956, #22723, #13700, #1828, #22871, #4250, #18271, #30093, #27628, #2126, #27486, #11107, #20262, #29647, #13546, #6845, #11397, #20704, #27781, #16134, #27928, #6540, #25455, #25159, #1979, #20561, #6694, #4545, #15982, #13835, #23158, #20857, #30241, #6990, #13254, #22573, #1674, #10954, #8664, #17970, #2424, #9402, #16590, #23615, #4839, #14282, #9864, #26067, #28534, #5142, #5300, #14585, #2711, #16887, #23466, #18731, #11848, #716, #11700, #28078, #23934, #7134, #2575, #21159, #21470, #16745, #273, #16434 ),
 ( #19177, #25756, #9556, #7583, #26217, #3026, #25591, #14137, #12302, #21619, #11999, #28388, #10009, #18877, #19324, #28683, #23309, #16279, #28234, #4686, #7287, #25915, #21314, #4991, #579, #13979, #12156, #14433, #9706, #21017, #423, #121, #19031, #7442, #23776, #2871, #21775, #26994, #26839, #12449, #7885, #14881, #6051, #10163, #12755, #19475, #19932, #876, #15340, #24075, #22222, #24677, #13061, #22079, #12908, #5451, #24227, #17488, #1181, #3768, #28847, #22384, #1489, #12605, #5909, #14732, #1332, #17193, #10623, #3616, #29299, #20087, #8335, #8176, #26520, #10778, #19623, #5602, #3326, #7732, #3465, #10462, #17045, #26372, #15191, #17638, #8026, #3178, #21922, #19767, #1034, #10315, #28989, #17334, #26680, #5756, #29138, #15038, #24371, #24523, #1787, #20672, #20227, #8776, #6505, #17931, #13664, #30056, #25274, #8923, #22839, #9067, #29613, #3919, #11368, #6360, #18237, #6654, #13217, #18394, #27595, #22541, #8630, #15654, #27747, #1639, #4213, #10918, #6806, #27306, #16098, #15498, #22988, #25423, #4512, #13512, #4360, #27142, #24986, #15947, #1942, #13801, #4068, #23128, #2238, #13361, #2091, #6206, #11508, #22686, #29463, #8481, #17782, #24829, #11074, #29914, #20376, #29766, #18090, #27454, #15796, #25123, #11226, #20528, #14555, #23902, #9678, #26036, #21133, #2999, #14401, #25884, #16401, #13948, #7101, #26186, #25726, #23435, #2680, #28046, #23279, #4962, #2547, #12126, #28506, #18700 ) ),
 .UNSPECIFIED., .T., .F., .F. ) 
 B_SPLINE_SURFACE_WITH_KNOTS ( ( 4, 3, 4 ),
 ( 4, 2, 2, 2, 2, 2, 2, 2, 2, 2, 2, 2, 2, 2, 2, 2, 2, 2, 2, 2, 2, 2, 2, 2, 2, 2, 2, 2, 2, 2, 2, 2, 2, 2, 2, 2, 2, 2, 2, 2, 2, 2, 2, 2, 2, 2, 2, 2, 2, 2, 2, 2, 2, 2, 2, 2, 2, 2, 2, 2, 2, 2, 2, 2, 2, 2, 2, 2, 2, 2, 2, 2, 2, 2, 2, 2, 2, 2, 2, 2, 2, 2, 2, 2, 2, 2, 2, 2, 2, 2, 2, 2, 4 ),
 ( 0.000000000000000000, 0.5000000000000000000, 1.000000000000000000 ),
 ( 0.000000000000000000, 0.2329478137359916323, 0.2349098735327962983, 0.2358909034311986175, 0.2363814183803997770, 0.2366266758550003568, 0.2367493045923006467, 0.2368106189609507917, 0.2368719333296009644, 0.2369056680493116240, 0.2369394027690223115, 0.2370068722084436863, 0.2371418110872863805, 0.2374116888449718243, 0.2379514443603427121, 0.2390309553910844875, 0.2411899774525679829, 0.2455080215755349737, 0.2541441098214689553, 0.2714162863133369186, 0.2886884628052048818, 0.2973245510511388634, 0.3016425951741058542, 0.3038016172355893496, 0.3048811282663310696, 0.3054208837817019573, 0.3056907615393874011, 0.3058257004182300953, 0.3058931698576514702, 0.3059269045773621576, 0.3059606392970728450, 0.3060023410584322145, 0.3060440428197915841, 0.3061274463425103787, 0.3062942533879479123, 0.3066278674788229797, 0.3072950956605731143, 0.3086295520240733836, 0.3112984647510739222, 0.3166362902050750550, 0.3273119411130772649, 0.3486632429290816293, 0.3913658465610904136, 0.4767710538251080377, 0.5621762610891256617, 0.6048788647211345015, 0.6262301665371388104, 0.6369058174451409648, 0.6422436428991420421, 0.6449125556261425807, 0.6462470119896428500, 0.6469142401713929846, 0.6472478542622681630, 0.6474146613077056411, 0.6474980648304244912, 0.6475397665917839163, 0.6475814683531432303, 0.6476196945210073164, 0.6476579206888715134, 0.6477343730245996856, 0.6478872776960560298, 0.6481930870389687183, 0.6488047057247940952, 0.6500279430964450711, 0.6524744178397468009, 0.6573673673263502604, 0.6671532662995571794, 0.6769391652727642095, 0.6867250642459712395, 0.6965109632191782696, 0.7062968621923852997, 0.7160827611655922187, 0.7209757106521956782, 0.7234221853954974080, 0.7246454227671483839, 0.7252570414529737608, 0.7255628507958864493, 0.7257157554673427935, 0.7257922078030709656, 0.7258304339709351627, 0.7258686601387992487, 0.7259088784260310234, 0.7259490967132626871, 0.7260295332877260144, 0.7261904064366526690, 0.7265121527345062002, 0.7271556453302130407, 0.7284426305216267217, 0.7310166009044543056, 0.7361645416701092515, 0.7464604232014193652, 0.7670521862640395927, 1.000000000000000000 ),
 .UNSPECIFIED. ) 
 GEOMETRIC_REPRESENTATION_ITEM ( )  RATIONAL_B_SPLINE_SURFACE ( (
 ( 1.000000000000000000, 1.000000000000000000, 1.000000000000000000, 1.000000000000000000, 1.000000000000000000, 1.000000000000000000, 1.000000000000000000, 1.000000000000000000, 1.000000000000000000, 1.000000000000000000, 1.000000000000000000, 1.000000000000000000, 1.000000000000000000, 1.000000000000000000, 1.000000000000000000, 1.000000000000000000, 1.000000000000000000, 1.000000000000000000, 1.000000000000000000, 1.000000000000000000, 1.000000000000000000, 1.000000000000000000, 1.000000000000000000, 1.000000000000000000, 1.000000000000000000, 1.000000000000000000, 1.000000000000000000, 1.000000000000000000, 1.000000000000000000, 1.000000000000000000, 1.000000000000000000, 1.000000000000000000, 1.000000000000000000, 1.000000000000000000, 1.000000000000000000, 1.000000000000000000, 1.000000000000000000, 1.000000000000000000, 1.000000000000000000, 1.000000000000000000, 1.000000000000000000, 1.000000000000000000, 1.000000000000000000, 1.000000000000000000, 1.000000000000000000, 1.000000000000000000, 1.000000000000000000, 1.000000000000000000, 1.000000000000000000, 1.000000000000000000, 1.000000000000000000, 1.000000000000000000, 1.000000000000000000, 1.000000000000000000, 1.000000000000000000, 1.000000000000000000, 1.000000000000000000, 1.000000000000000000, 1.000000000000000000, 1.000000000000000000, 1.000000000000000000, 1.000000000000000000, 1.000000000000000000, 1.000000000000000000, 1.000000000000000000, 1.000000000000000000, 1.000000000000000000, 1.000000000000000000, 1.000000000000000000, 1.000000000000000000, 1.000000000000000000, 1.000000000000000000, 1.000000000000000000, 1.000000000000000000, 1.000000000000000000, 1.000000000000000000, 1.000000000000000000, 1.000000000000000000, 1.000000000000000000, 1.000000000000000000, 1.000000000000000000, 1.000000000000000000, 1.000000000000000000, 1.000000000000000000, 1.000000000000000000, 1.000000000000000000, 1.000000000000000000, 1.000000000000000000, 1.000000000000000000, 1.000000000000000000, 1.000000000000000000, 1.000000000000000000, 1.000000000000000000, 1.000000000000000000, 1.000000000000000000, 1.000000000000000000, 1.000000000000000000, 1.000000000000000000, 1.000000000000000000, 1.000000000000000000, 1.000000000000000000, 1.000000000000000000, 1.000000000000000000, 1.000000000000000000, 1.000000000000000000, 1.000000000000000000, 1.000000000000000000, 1.000000000000000000, 1.000000000000000000, 1.000000000000000000, 1.000000000000000000, 1.000000000000000000, 1.000000000000000000, 1.000000000000000000, 1.000000000000000000, 1.000000000000000000, 1.000000000000000000, 1.000000000000000000, 1.000000000000000000, 1.000000000000000000, 1.000000000000000000, 1.000000000000000000, 1.000000000000000000, 1.000000000000000000, 1.000000000000000000, 1.000000000000000000, 1.000000000000000000, 1.000000000000000000, 1.000000000000000000, 1.000000000000000000, 1.000000000000000000, 1.000000000000000000, 1.000000000000000000, 1.000000000000000000, 1.000000000000000000, 1.000000000000000000, 1.000000000000000000, 1.000000000000000000, 1.000000000000000000, 1.000000000000000000, 1.000000000000000000, 1.000000000000000000, 1.000000000000000000, 1.000000000000000000, 1.000000000000000000, 1.000000000000000000, 1.000000000000000000, 1.000000000000000000, 1.000000000000000000, 1.000000000000000000, 1.000000000000000000, 1.000000000000000000, 1.000000000000000000, 1.000000000000000000, 1.000000000000000000, 1.000000000000000000, 1.000000000000000000, 1.000000000000000000, 1.000000000000000000, 1.000000000000000000, 1.000000000000000000, 1.000000000000000000, 1.000000000000000000, 1.000000000000000000, 1.000000000000000000, 1.000000000000000000, 1.000000000000000000, 1.000000000000000000, 1.000000000000000000, 1.000000000000000000, 1.000000000000000000, 1.000000000000000000, 1.000000000000000000, 1.000000000000000000, 1.000000000000000000, 1.000000000000000000, 1.000000000000000000, 1.000000000000000000, 1.000000000000000000, 1.000000000000000000, 1.000000000000000000, 1.000000000000000000, 1.000000000000000000, 1.000000000000000000, 1.000000000000000000, 1.000000000000000000),
 ( 0.3333333333333333703, 0.3333333333333333703, 0.3333333333333333703, 0.3333333333333333703, 0.3333333333333333703, 0.3333333333333333703, 0.3333333333333333703, 0.3333333333333333703, 0.3333333333333333703, 0.3333333333333333703, 0.3333333333333333703, 0.3333333333333333703, 0.3333333333333333703, 0.3333333333333333703, 0.3333333333333333703, 0.3333333333333333703, 0.3333333333333333703, 0.3333333333333333703, 0.3333333333333333703, 0.3333333333333333703, 0.3333333333333333703, 0.3333333333333333703, 0.3333333333333333703, 0.3333333333333333703, 0.3333333333333333703, 0.3333333333333333703, 0.3333333333333333703, 0.3333333333333333703, 0.3333333333333333703, 0.3333333333333333703, 0.3333333333333333703, 0.3333333333333333703, 0.3333333333333333703, 0.3333333333333333703, 0.3333333333333333703, 0.3333333333333333703, 0.3333333333333333703, 0.3333333333333333703, 0.3333333333333333703, 0.3333333333333333703, 0.3333333333333333703, 0.3333333333333333703, 0.3333333333333333703, 0.3333333333333333703, 0.3333333333333333703, 0.3333333333333333703, 0.3333333333333333703, 0.3333333333333333703, 0.3333333333333333703, 0.3333333333333333703, 0.3333333333333333703, 0.3333333333333333703, 0.3333333333333333703, 0.3333333333333333703, 0.3333333333333333703, 0.3333333333333333703, 0.3333333333333333703, 0.3333333333333333703, 0.3333333333333333703, 0.3333333333333333703, 0.3333333333333333703, 0.3333333333333333703, 0.3333333333333333703, 0.3333333333333333703, 0.3333333333333333703, 0.3333333333333333703, 0.3333333333333333703, 0.3333333333333333703, 0.3333333333333333703, 0.3333333333333333703, 0.3333333333333333703, 0.3333333333333333703, 0.3333333333333333703, 0.3333333333333333703, 0.3333333333333333703, 0.3333333333333333703, 0.3333333333333333703, 0.3333333333333333703, 0.3333333333333333703, 0.3333333333333333703, 0.3333333333333333703, 0.3333333333333333703, 0.3333333333333333703, 0.3333333333333333703, 0.3333333333333333703, 0.3333333333333333703, 0.3333333333333333703, 0.3333333333333333703, 0.3333333333333333703, 0.3333333333333333703, 0.3333333333333333703, 0.3333333333333333703, 0.3333333333333333703, 0.3333333333333333703, 0.3333333333333333703, 0.3333333333333333703, 0.3333333333333333703, 0.3333333333333333703, 0.3333333333333333703, 0.3333333333333333703, 0.3333333333333333703, 0.3333333333333333703, 0.3333333333333333703, 0.3333333333333333703, 0.3333333333333333703, 0.3333333333333333703, 0.3333333333333333703, 0.3333333333333333703, 0.3333333333333333703, 0.3333333333333333703, 0.3333333333333333703, 0.3333333333333333703, 0.3333333333333333703, 0.3333333333333333703, 0.3333333333333333703, 0.3333333333333333703, 0.3333333333333333703, 0.3333333333333333703, 0.3333333333333333703, 0.3333333333333333703, 0.3333333333333333703, 0.3333333333333333703, 0.3333333333333333703, 0.3333333333333333703, 0.3333333333333333703, 0.3333333333333333703, 0.3333333333333333703, 0.3333333333333333703, 0.3333333333333333703, 0.3333333333333333703, 0.3333333333333333703, 0.3333333333333333703, 0.3333333333333333703, 0.3333333333333333703, 0.3333333333333333703, 0.3333333333333333703, 0.3333333333333333703, 0.3333333333333333703, 0.3333333333333333703, 0.3333333333333333703, 0.3333333333333333703, 0.3333333333333333703, 0.3333333333333333703, 0.3333333333333333703, 0.3333333333333333703, 0.3333333333333333703, 0.3333333333333333703, 0.3333333333333333703, 0.3333333333333333703, 0.3333333333333333703, 0.3333333333333333703, 0.3333333333333333703, 0.3333333333333333703, 0.3333333333333333703, 0.3333333333333333703, 0.3333333333333333703, 0.3333333333333333703, 0.3333333333333333703, 0.3333333333333333703, 0.3333333333333333703, 0.3333333333333333703, 0.3333333333333333703, 0.3333333333333333703, 0.3333333333333333703, 0.3333333333333333703, 0.3333333333333333703, 0.3333333333333333703, 0.3333333333333333703, 0.3333333333333333703, 0.3333333333333333703, 0.3333333333333333703, 0.3333333333333333703, 0.3333333333333333703, 0.3333333333333333703, 0.3333333333333333703, 0.3333333333333333703, 0.3333333333333333703, 0.3333333333333333703, 0.3333333333333333703, 0.3333333333333333703, 0.3333333333333333703, 0.3333333333333333703, 0.3333333333333333703, 0.3333333333333333703, 0.3333333333333333703, 0.3333333333333333703),
 ( 0.3333333333333333703, 0.3333333333333333703, 0.3333333333333333703, 0.3333333333333333703, 0.3333333333333333703, 0.3333333333333333703, 0.3333333333333333703, 0.3333333333333333703, 0.3333333333333333703, 0.3333333333333333703, 0.3333333333333333703, 0.3333333333333333703, 0.3333333333333333703, 0.3333333333333333703, 0.3333333333333333703, 0.3333333333333333703, 0.3333333333333333703, 0.3333333333333333703, 0.3333333333333333703, 0.3333333333333333703, 0.3333333333333333703, 0.3333333333333333703, 0.3333333333333333703, 0.3333333333333333703, 0.3333333333333333703, 0.3333333333333333703, 0.3333333333333333703, 0.3333333333333333703, 0.3333333333333333703, 0.3333333333333333703, 0.3333333333333333703, 0.3333333333333333703, 0.3333333333333333703, 0.3333333333333333703, 0.3333333333333333703, 0.3333333333333333703, 0.3333333333333333703, 0.3333333333333333703, 0.3333333333333333703, 0.3333333333333333703, 0.3333333333333333703, 0.3333333333333333703, 0.3333333333333333703, 0.3333333333333333703, 0.3333333333333333703, 0.3333333333333333703, 0.3333333333333333703, 0.3333333333333333703, 0.3333333333333333703, 0.3333333333333333703, 0.3333333333333333703, 0.3333333333333333703, 0.3333333333333333703, 0.3333333333333333703, 0.3333333333333333703, 0.3333333333333333703, 0.3333333333333333703, 0.3333333333333333703, 0.3333333333333333703, 0.3333333333333333703, 0.3333333333333333703, 0.3333333333333333703, 0.3333333333333333703, 0.3333333333333333703, 0.3333333333333333703, 0.3333333333333333703, 0.3333333333333333703, 0.3333333333333333703, 0.3333333333333333703, 0.3333333333333333703, 0.3333333333333333703, 0.3333333333333333703, 0.3333333333333333703, 0.3333333333333333703, 0.3333333333333333703, 0.3333333333333333703, 0.3333333333333333703, 0.3333333333333333703, 0.3333333333333333703, 0.3333333333333333703, 0.3333333333333333703, 0.3333333333333333703, 0.3333333333333333703, 0.3333333333333333703, 0.3333333333333333703, 0.3333333333333333703, 0.3333333333333333703, 0.3333333333333333703, 0.3333333333333333703, 0.3333333333333333703, 0.3333333333333333703, 0.3333333333333333703, 0.3333333333333333703, 0.3333333333333333703, 0.3333333333333333703, 0.3333333333333333703, 0.3333333333333333703, 0.3333333333333333703, 0.3333333333333333703, 0.3333333333333333703, 0.3333333333333333703, 0.3333333333333333703, 0.3333333333333333703, 0.3333333333333333703, 0.3333333333333333703, 0.3333333333333333703, 0.3333333333333333703, 0.3333333333333333703, 0.3333333333333333703, 0.3333333333333333703, 0.3333333333333333703, 0.3333333333333333703, 0.3333333333333333703, 0.3333333333333333703, 0.3333333333333333703, 0.3333333333333333703, 0.3333333333333333703, 0.3333333333333333703, 0.3333333333333333703, 0.3333333333333333703, 0.3333333333333333703, 0.3333333333333333703, 0.3333333333333333703, 0.3333333333333333703, 0.3333333333333333703, 0.3333333333333333703, 0.3333333333333333703, 0.3333333333333333703, 0.3333333333333333703, 0.3333333333333333703, 0.3333333333333333703, 0.3333333333333333703, 0.3333333333333333703, 0.3333333333333333703, 0.3333333333333333703, 0.3333333333333333703, 0.3333333333333333703, 0.3333333333333333703, 0.3333333333333333703, 0.3333333333333333703, 0.3333333333333333703, 0.3333333333333333703, 0.3333333333333333703, 0.3333333333333333703, 0.3333333333333333703, 0.3333333333333333703, 0.3333333333333333703, 0.3333333333333333703, 0.3333333333333333703, 0.3333333333333333703, 0.3333333333333333703, 0.3333333333333333703, 0.3333333333333333703, 0.3333333333333333703, 0.3333333333333333703, 0.3333333333333333703, 0.3333333333333333703, 0.3333333333333333703, 0.3333333333333333703, 0.3333333333333333703, 0.3333333333333333703, 0.3333333333333333703, 0.3333333333333333703, 0.3333333333333333703, 0.3333333333333333703, 0.3333333333333333703, 0.3333333333333333703, 0.3333333333333333703, 0.3333333333333333703, 0.3333333333333333703, 0.3333333333333333703, 0.3333333333333333703, 0.3333333333333333703, 0.3333333333333333703, 0.3333333333333333703, 0.3333333333333333703, 0.3333333333333333703, 0.3333333333333333703, 0.3333333333333333703, 0.3333333333333333703, 0.3333333333333333703, 0.3333333333333333703, 0.3333333333333333703, 0.3333333333333333703, 0.3333333333333333703, 0.3333333333333333703),
 ( 1.000000000000000000, 1.000000000000000000, 1.000000000000000000, 1.000000000000000000, 1.000000000000000000, 1.000000000000000000, 1.000000000000000000, 1.000000000000000000, 1.000000000000000000, 1.000000000000000000, 1.000000000000000000, 1.000000000000000000, 1.000000000000000000, 1.000000000000000000, 1.000000000000000000, 1.000000000000000000, 1.000000000000000000, 1.000000000000000000, 1.000000000000000000, 1.000000000000000000, 1.000000000000000000, 1.000000000000000000, 1.000000000000000000, 1.000000000000000000, 1.000000000000000000, 1.000000000000000000, 1.000000000000000000, 1.000000000000000000, 1.000000000000000000, 1.000000000000000000, 1.000000000000000000, 1.000000000000000000, 1.000000000000000000, 1.000000000000000000, 1.000000000000000000, 1.000000000000000000, 1.000000000000000000, 1.000000000000000000, 1.000000000000000000, 1.000000000000000000, 1.000000000000000000, 1.000000000000000000, 1.000000000000000000, 1.000000000000000000, 1.000000000000000000, 1.000000000000000000, 1.000000000000000000, 1.000000000000000000, 1.000000000000000000, 1.000000000000000000, 1.000000000000000000, 1.000000000000000000, 1.000000000000000000, 1.000000000000000000, 1.000000000000000000, 1.000000000000000000, 1.000000000000000000, 1.000000000000000000, 1.000000000000000000, 1.000000000000000000, 1.000000000000000000, 1.000000000000000000, 1.000000000000000000, 1.000000000000000000, 1.000000000000000000, 1.000000000000000000, 1.000000000000000000, 1.000000000000000000, 1.000000000000000000, 1.000000000000000000, 1.000000000000000000, 1.000000000000000000, 1.000000000000000000, 1.000000000000000000, 1.000000000000000000, 1.000000000000000000, 1.000000000000000000, 1.000000000000000000, 1.000000000000000000, 1.000000000000000000, 1.000000000000000000, 1.000000000000000000, 1.000000000000000000, 1.000000000000000000, 1.000000000000000000, 1.000000000000000000, 1.000000000000000000, 1.000000000000000000, 1.000000000000000000, 1.000000000000000000, 1.000000000000000000, 1.000000000000000000, 1.000000000000000000, 1.000000000000000000, 1.000000000000000000, 1.000000000000000000, 1.000000000000000000, 1.000000000000000000, 1.000000000000000000, 1.000000000000000000, 1.000000000000000000, 1.000000000000000000, 1.000000000000000000, 1.000000000000000000, 1.000000000000000000, 1.000000000000000000, 1.000000000000000000, 1.000000000000000000, 1.000000000000000000, 1.000000000000000000, 1.000000000000000000, 1.000000000000000000, 1.000000000000000000, 1.000000000000000000, 1.000000000000000000, 1.000000000000000000, 1.000000000000000000, 1.000000000000000000, 1.000000000000000000, 1.000000000000000000, 1.000000000000000000, 1.000000000000000000, 1.000000000000000000, 1.000000000000000000, 1.000000000000000000, 1.000000000000000000, 1.000000000000000000, 1.000000000000000000, 1.000000000000000000, 1.000000000000000000, 1.000000000000000000, 1.000000000000000000, 1.000000000000000000, 1.000000000000000000, 1.000000000000000000, 1.000000000000000000, 1.000000000000000000, 1.000000000000000000, 1.000000000000000000, 1.000000000000000000, 1.000000000000000000, 1.000000000000000000, 1.000000000000000000, 1.000000000000000000, 1.000000000000000000, 1.000000000000000000, 1.000000000000000000, 1.000000000000000000, 1.000000000000000000, 1.000000000000000000, 1.000000000000000000, 1.000000000000000000, 1.000000000000000000, 1.000000000000000000, 1.000000000000000000, 1.000000000000000000, 1.000000000000000000, 1.000000000000000000, 1.000000000000000000, 1.000000000000000000, 1.000000000000000000, 1.000000000000000000, 1.000000000000000000, 1.000000000000000000, 1.000000000000000000, 1.000000000000000000, 1.000000000000000000, 1.000000000000000000, 1.000000000000000000, 1.000000000000000000, 1.000000000000000000, 1.000000000000000000, 1.000000000000000000, 1.000000000000000000, 1.000000000000000000, 1.000000000000000000, 1.000000000000000000, 1.000000000000000000, 1.000000000000000000, 1.000000000000000000, 1.000000000000000000, 1.000000000000000000, 1.000000000000000000, 1.000000000000000000, 1.000000000000000000, 1.000000000000000000),
 ( 0.3333333333333333703, 0.3333333333333333703, 0.3333333333333333703, 0.3333333333333333703, 0.3333333333333333703, 0.3333333333333333703, 0.3333333333333333703, 0.3333333333333333703, 0.3333333333333333703, 0.3333333333333333703, 0.3333333333333333703, 0.3333333333333333703, 0.3333333333333333703, 0.3333333333333333703, 0.3333333333333333703, 0.3333333333333333703, 0.3333333333333333703, 0.3333333333333333703, 0.3333333333333333703, 0.3333333333333333703, 0.3333333333333333703, 0.3333333333333333703, 0.3333333333333333703, 0.3333333333333333703, 0.3333333333333333703, 0.3333333333333333703, 0.3333333333333333703, 0.3333333333333333703, 0.3333333333333333703, 0.3333333333333333703, 0.3333333333333333703, 0.3333333333333333703, 0.3333333333333333703, 0.3333333333333333703, 0.3333333333333333703, 0.3333333333333333703, 0.3333333333333333703, 0.3333333333333333703, 0.3333333333333333703, 0.3333333333333333703, 0.3333333333333333703, 0.3333333333333333703, 0.3333333333333333703, 0.3333333333333333703, 0.3333333333333333703, 0.3333333333333333703, 0.3333333333333333703, 0.3333333333333333703, 0.3333333333333333703, 0.3333333333333333703, 0.3333333333333333703, 0.3333333333333333703, 0.3333333333333333703, 0.3333333333333333703, 0.3333333333333333703, 0.3333333333333333703, 0.3333333333333333703, 0.3333333333333333703, 0.3333333333333333703, 0.3333333333333333703, 0.3333333333333333703, 0.3333333333333333703, 0.3333333333333333703, 0.3333333333333333703, 0.3333333333333333703, 0.3333333333333333703, 0.3333333333333333703, 0.3333333333333333703, 0.3333333333333333703, 0.3333333333333333703, 0.3333333333333333703, 0.3333333333333333703, 0.3333333333333333703, 0.3333333333333333703, 0.3333333333333333703, 0.3333333333333333703, 0.3333333333333333703, 0.3333333333333333703, 0.3333333333333333703, 0.3333333333333333703, 0.3333333333333333703, 0.3333333333333333703, 0.3333333333333333703, 0.3333333333333333703, 0.3333333333333333703, 0.3333333333333333703, 0.3333333333333333703, 0.3333333333333333703, 0.3333333333333333703, 0.3333333333333333703, 0.3333333333333333703, 0.3333333333333333703, 0.3333333333333333703, 0.3333333333333333703, 0.3333333333333333703, 0.3333333333333333703, 0.3333333333333333703, 0.3333333333333333703, 0.3333333333333333703, 0.3333333333333333703, 0.3333333333333333703, 0.3333333333333333703, 0.3333333333333333703, 0.3333333333333333703, 0.3333333333333333703, 0.3333333333333333703, 0.3333333333333333703, 0.3333333333333333703, 0.3333333333333333703, 0.3333333333333333703, 0.3333333333333333703, 0.3333333333333333703, 0.3333333333333333703, 0.3333333333333333703, 0.3333333333333333703, 0.3333333333333333703, 0.3333333333333333703, 0.3333333333333333703, 0.3333333333333333703, 0.3333333333333333703, 0.3333333333333333703, 0.3333333333333333703, 0.3333333333333333703, 0.3333333333333333703, 0.3333333333333333703, 0.3333333333333333703, 0.3333333333333333703, 0.3333333333333333703, 0.3333333333333333703, 0.3333333333333333703, 0.3333333333333333703, 0.3333333333333333703, 0.3333333333333333703, 0.3333333333333333703, 0.3333333333333333703, 0.3333333333333333703, 0.3333333333333333703, 0.3333333333333333703, 0.3333333333333333703, 0.3333333333333333703, 0.3333333333333333703, 0.3333333333333333703, 0.3333333333333333703, 0.3333333333333333703, 0.3333333333333333703, 0.3333333333333333703, 0.3333333333333333703, 0.3333333333333333703, 0.3333333333333333703, 0.3333333333333333703, 0.3333333333333333703, 0.3333333333333333703, 0.3333333333333333703, 0.3333333333333333703, 0.3333333333333333703, 0.3333333333333333703, 0.3333333333333333703, 0.3333333333333333703, 0.3333333333333333703, 0.3333333333333333703, 0.3333333333333333703, 0.3333333333333333703, 0.3333333333333333703, 0.3333333333333333703, 0.3333333333333333703, 0.3333333333333333703, 0.3333333333333333703, 0.3333333333333333703, 0.3333333333333333703, 0.3333333333333333703, 0.3333333333333333703, 0.3333333333333333703, 0.3333333333333333703, 0.3333333333333333703, 0.3333333333333333703, 0.3333333333333333703, 0.3333333333333333703, 0.3333333333333333703, 0.3333333333333333703, 0.3333333333333333703, 0.3333333333333333703, 0.3333333333333333703, 0.3333333333333333703, 0.3333333333333333703, 0.3333333333333333703, 0.3333333333333333703),
 ( 0.3333333333333333703, 0.3333333333333333703, 0.3333333333333333703, 0.3333333333333333703, 0.3333333333333333703, 0.3333333333333333703, 0.3333333333333333703, 0.3333333333333333703, 0.3333333333333333703, 0.3333333333333333703, 0.3333333333333333703, 0.3333333333333333703, 0.3333333333333333703, 0.3333333333333333703, 0.3333333333333333703, 0.3333333333333333703, 0.3333333333333333703, 0.3333333333333333703, 0.3333333333333333703, 0.3333333333333333703, 0.3333333333333333703, 0.3333333333333333703, 0.3333333333333333703, 0.3333333333333333703, 0.3333333333333333703, 0.3333333333333333703, 0.3333333333333333703, 0.3333333333333333703, 0.3333333333333333703, 0.3333333333333333703, 0.3333333333333333703, 0.3333333333333333703, 0.3333333333333333703, 0.3333333333333333703, 0.3333333333333333703, 0.3333333333333333703, 0.3333333333333333703, 0.3333333333333333703, 0.3333333333333333703, 0.3333333333333333703, 0.3333333333333333703, 0.3333333333333333703, 0.3333333333333333703, 0.3333333333333333703, 0.3333333333333333703, 0.3333333333333333703, 0.3333333333333333703, 0.3333333333333333703, 0.3333333333333333703, 0.3333333333333333703, 0.3333333333333333703, 0.3333333333333333703, 0.3333333333333333703, 0.3333333333333333703, 0.3333333333333333703, 0.3333333333333333703, 0.3333333333333333703, 0.3333333333333333703, 0.3333333333333333703, 0.3333333333333333703, 0.3333333333333333703, 0.3333333333333333703, 0.3333333333333333703, 0.3333333333333333703, 0.3333333333333333703, 0.3333333333333333703, 0.3333333333333333703, 0.3333333333333333703, 0.3333333333333333703, 0.3333333333333333703, 0.3333333333333333703, 0.3333333333333333703, 0.3333333333333333703, 0.3333333333333333703, 0.3333333333333333703, 0.3333333333333333703, 0.3333333333333333703, 0.3333333333333333703, 0.3333333333333333703, 0.3333333333333333703, 0.3333333333333333703, 0.3333333333333333703, 0.3333333333333333703, 0.3333333333333333703, 0.3333333333333333703, 0.3333333333333333703, 0.3333333333333333703, 0.3333333333333333703, 0.3333333333333333703, 0.3333333333333333703, 0.3333333333333333703, 0.3333333333333333703, 0.3333333333333333703, 0.3333333333333333703, 0.3333333333333333703, 0.3333333333333333703, 0.3333333333333333703, 0.3333333333333333703, 0.3333333333333333703, 0.3333333333333333703, 0.3333333333333333703, 0.3333333333333333703, 0.3333333333333333703, 0.3333333333333333703, 0.3333333333333333703, 0.3333333333333333703, 0.3333333333333333703, 0.3333333333333333703, 0.3333333333333333703, 0.3333333333333333703, 0.3333333333333333703, 0.3333333333333333703, 0.3333333333333333703, 0.3333333333333333703, 0.3333333333333333703, 0.3333333333333333703, 0.3333333333333333703, 0.3333333333333333703, 0.3333333333333333703, 0.3333333333333333703, 0.3333333333333333703, 0.3333333333333333703, 0.3333333333333333703, 0.3333333333333333703, 0.3333333333333333703, 0.3333333333333333703, 0.3333333333333333703, 0.3333333333333333703, 0.3333333333333333703, 0.3333333333333333703, 0.3333333333333333703, 0.3333333333333333703, 0.3333333333333333703, 0.3333333333333333703, 0.3333333333333333703, 0.3333333333333333703, 0.3333333333333333703, 0.3333333333333333703, 0.3333333333333333703, 0.3333333333333333703, 0.3333333333333333703, 0.3333333333333333703, 0.3333333333333333703, 0.3333333333333333703, 0.3333333333333333703, 0.3333333333333333703, 0.3333333333333333703, 0.3333333333333333703, 0.3333333333333333703, 0.3333333333333333703, 0.3333333333333333703, 0.3333333333333333703, 0.3333333333333333703, 0.3333333333333333703, 0.3333333333333333703, 0.3333333333333333703, 0.3333333333333333703, 0.3333333333333333703, 0.3333333333333333703, 0.3333333333333333703, 0.3333333333333333703, 0.3333333333333333703, 0.3333333333333333703, 0.3333333333333333703, 0.3333333333333333703, 0.3333333333333333703, 0.3333333333333333703, 0.3333333333333333703, 0.3333333333333333703, 0.3333333333333333703, 0.3333333333333333703, 0.3333333333333333703, 0.3333333333333333703, 0.3333333333333333703, 0.3333333333333333703, 0.3333333333333333703, 0.3333333333333333703, 0.3333333333333333703, 0.3333333333333333703, 0.3333333333333333703, 0.3333333333333333703, 0.3333333333333333703, 0.3333333333333333703, 0.3333333333333333703, 0.3333333333333333703, 0.3333333333333333703),
 ( 1.000000000000000000, 1.000000000000000000, 1.000000000000000000, 1.000000000000000000, 1.000000000000000000, 1.000000000000000000, 1.000000000000000000, 1.000000000000000000, 1.000000000000000000, 1.000000000000000000, 1.000000000000000000, 1.000000000000000000, 1.000000000000000000, 1.000000000000000000, 1.000000000000000000, 1.000000000000000000, 1.000000000000000000, 1.000000000000000000, 1.000000000000000000, 1.000000000000000000, 1.000000000000000000, 1.000000000000000000, 1.000000000000000000, 1.000000000000000000, 1.000000000000000000, 1.000000000000000000, 1.000000000000000000, 1.000000000000000000, 1.000000000000000000, 1.000000000000000000, 1.000000000000000000, 1.000000000000000000, 1.000000000000000000, 1.000000000000000000, 1.000000000000000000, 1.000000000000000000, 1.000000000000000000, 1.000000000000000000, 1.000000000000000000, 1.000000000000000000, 1.000000000000000000, 1.000000000000000000, 1.000000000000000000, 1.000000000000000000, 1.000000000000000000, 1.000000000000000000, 1.000000000000000000, 1.000000000000000000, 1.000000000000000000, 1.000000000000000000, 1.000000000000000000, 1.000000000000000000, 1.000000000000000000, 1.000000000000000000, 1.000000000000000000, 1.000000000000000000, 1.000000000000000000, 1.000000000000000000, 1.000000000000000000, 1.000000000000000000, 1.000000000000000000, 1.000000000000000000, 1.000000000000000000, 1.000000000000000000, 1.000000000000000000, 1.000000000000000000, 1.000000000000000000, 1.000000000000000000, 1.000000000000000000, 1.000000000000000000, 1.000000000000000000, 1.000000000000000000, 1.000000000000000000, 1.000000000000000000, 1.000000000000000000, 1.000000000000000000, 1.000000000000000000, 1.000000000000000000, 1.000000000000000000, 1.000000000000000000, 1.000000000000000000, 1.000000000000000000, 1.000000000000000000, 1.000000000000000000, 1.000000000000000000, 1.000000000000000000, 1.000000000000000000, 1.000000000000000000, 1.000000000000000000, 1.000000000000000000, 1.000000000000000000, 1.000000000000000000, 1.000000000000000000, 1.000000000000000000, 1.000000000000000000, 1.000000000000000000, 1.000000000000000000, 1.000000000000000000, 1.000000000000000000, 1.000000000000000000, 1.000000000000000000, 1.000000000000000000, 1.000000000000000000, 1.000000000000000000, 1.000000000000000000, 1.000000000000000000, 1.000000000000000000, 1.000000000000000000, 1.000000000000000000, 1.000000000000000000, 1.000000000000000000, 1.000000000000000000, 1.000000000000000000, 1.000000000000000000, 1.000000000000000000, 1.000000000000000000, 1.000000000000000000, 1.000000000000000000, 1.000000000000000000, 1.000000000000000000, 1.000000000000000000, 1.000000000000000000, 1.000000000000000000, 1.000000000000000000, 1.000000000000000000, 1.000000000000000000, 1.000000000000000000, 1.000000000000000000, 1.000000000000000000, 1.000000000000000000, 1.000000000000000000, 1.000000000000000000, 1.000000000000000000, 1.000000000000000000, 1.000000000000000000, 1.000000000000000000, 1.000000000000000000, 1.000000000000000000, 1.000000000000000000, 1.000000000000000000, 1.000000000000000000, 1.000000000000000000, 1.000000000000000000, 1.000000000000000000, 1.000000000000000000, 1.000000000000000000, 1.000000000000000000, 1.000000000000000000, 1.000000000000000000, 1.000000000000000000, 1.000000000000000000, 1.000000000000000000, 1.000000000000000000, 1.000000000000000000, 1.000000000000000000, 1.000000000000000000, 1.000000000000000000, 1.000000000000000000, 1.000000000000000000, 1.000000000000000000, 1.000000000000000000, 1.000000000000000000, 1.000000000000000000, 1.000000000000000000, 1.000000000000000000, 1.000000000000000000, 1.000000000000000000, 1.000000000000000000, 1.000000000000000000, 1.000000000000000000, 1.000000000000000000, 1.000000000000000000, 1.000000000000000000, 1.000000000000000000, 1.000000000000000000, 1.000000000000000000, 1.000000000000000000, 1.000000000000000000, 1.000000000000000000, 1.000000000000000000, 1.000000000000000000, 1.000000000000000000, 1.000000000000000000, 1.000000000000000000, 1.000000000000000000, 1.000000000000000000) ) ) 
 REPRESENTATION_ITEM ( '' )  SURFACE ( )  );
#5065=CARTESIAN_POINT ( 'NONE',  ( 10.70792791965113544, 16.69018921775036546, -15.96040338026158523 ) ) ;
#5070=CARTESIAN_POINT ( 'NONE',  ( 10.07879545831710999, 15.66271422494645904, -16.43741374977755143 ) ) ;
#5072=CARTESIAN_POINT ( 'NONE',  ( 9.668002105539015290, 16.22676391817335784, -17.88502066855795292 ) ) ;
#5073=CARTESIAN_POINT ( 'NONE',  ( 21.92347772697934261, 3.537472258236324052, -14.28107661384214211 ) ) ;
#5076=CARTESIAN_POINT ( 'NONE',  ( 28.47856004806874353, -11.16640101040803401, -12.66155532224275149 ) ) ;
#5079=CARTESIAN_POINT ( 'NONE',  ( 11.27643094638968613, 16.67581753947769130, -16.78442615493024803 ) ) ;
#5084=CARTESIAN_POINT ( 'NONE',  ( 33.69611315462438483, -12.86230108826256924, -18.75566652118837752 ) ) ;
#5085=CARTESIAN_POINT ( 'NONE',  ( 17.63704213852533442, 9.806822523219006271, -18.50018230520716145 ) ) ;
#5088=CARTESIAN_POINT ( 'NONE',  ( 9.760963200462100531, 13.20757681744125911, -16.78657487285272509 ) ) ;
#5090=CARTESIAN_POINT ( 'NONE',  ( 25.30932029414111284, -7.960302465696846852, -19.79224777486898645 ) ) ;
#5093=CARTESIAN_POINT ( 'NONE',  ( 19.85388831290292799, 7.668379621071204078, -15.62993620635094061 ) ) ;
#5094=CARTESIAN_POINT ( 'NONE',  ( 17.11242430243909141, 7.828829022555451544, -19.39938683153768295 ) ) ;
#5104=CARTESIAN_POINT ( 'NONE',  ( 9.879812780108833792, 16.57527415160161510, -16.52987074417163527 ) ) ;
#5105=CARTESIAN_POINT ( 'NONE',  ( 27.04162508513615393, -6.753966733322825711, -13.61186222264828771 ) ) ;
#5106=CARTESIAN_POINT ( 'NONE',  ( 20.59283418570449697, -4.290598171560842111, -16.90930062131523215 ) ) ;
#5107=CARTESIAN_POINT ( 'NONE',  ( 36.54859390953723874, -23.18451583373416014, -14.99999999999999822 ) ) ;
#5114=CARTESIAN_POINT ( 'NONE',  ( 15.39489021548154568, 6.697694061803245447, -14.95590323207311734 ) ) ;
#5116=CARTESIAN_POINT ( 'NONE',  ( 10.33811693838771717, 18.38618951776012267, -17.91796598306941135 ) ) ;
#5117=DIRECTION ( 'NONE',  ( -1.000000000000000000, 0.000000000000000000, 0.000000000000000000 ) ) ;
#5120=CARTESIAN_POINT ( 'NONE',  ( 14.29829396236512729, 6.476847147513518088, -18.28004444394726491 ) ) ;
#5123=CARTESIAN_POINT ( 'NONE',  ( 14.70433163182692482, 6.391443753141328621, -13.74806202935933541 ) ) ;
#5126=CARTESIAN_POINT ( 'NONE',  ( 33.57712230886461668, -13.32773824946660923, -19.76201999124979736 ) ) ;
#5128=CARTESIAN_POINT ( 'NONE',  ( 22.26732294003774015, -3.469656073077215463, -14.71322089325822624 ) ) ;
#5130=CARTESIAN_POINT ( 'NONE',  ( 22.34502977332646978, 2.679400364154326919, -18.33342593408658061 ) ) ;
#5131=CARTESIAN_POINT ( 'NONE',  ( 27.40270966038060152, -12.25096941946872953, -16.90735844088681006 ) ) ;
#5141=CARTESIAN_POINT ( 'NONE',  ( 34.56382110058589774, -12.26799042007339757, -18.94768870749412315 ) ) ;
#5142=CARTESIAN_POINT ( 'NONE',  ( 12.75938622741416140, 7.627299838292535661, -14.92343961094405103 ) ) ;
#5147=CARTESIAN_POINT ( 'NONE',  ( 12.02859841272590735, 9.313533661810568631, -16.69110409223909741 ) ) ;
#5162=CARTESIAN_POINT ( 'NONE',  ( 12.27065153619900961, 7.644304191818388716, -16.55295716654172722 ) ) ;
#5163=CARTESIAN_POINT ( 'NONE',  ( 23.69966960967911973, -9.104540460734687812, -16.16703237251472558 ) ) ;
#5164=CARTESIAN_POINT ( 'NONE',  ( 26.20148740379470453, -2.166401353139026487, -14.75472287570676322 ) ) ;
#5176=CARTESIAN_POINT ( 'NONE',  ( 12.02748425217687789, 9.318634685891279190, -16.69156549717016702 ) ) ;
#5178=CARTESIAN_POINT ( 'NONE',  ( 35.09336438560361415, -20.13941072448723801, -20.22035334018532637 ) ) ;
#5180=CARTESIAN_POINT ( 'NONE',  ( 8.944584683310379702, 16.95159276115599667, -17.94384837343789130 ) ) ;
#5182=CARTESIAN_POINT ( 'NONE',  ( 16.94076125623460527, 0.4124075662712927692, -16.40086227390004936 ) ) ;
#5183=CARTESIAN_POINT ( 'NONE',  ( 12.83348778413740376, 9.536125428572121976, -16.14043921975381934 ) ) ;
#5186=CARTESIAN_POINT ( 'NONE',  ( 11.58682163191119230, 8.958038730125363003, -15.79767441425272345 ) ) ;
#5189=CARTESIAN_POINT ( 'NONE',  ( 11.14863080475985591, 10.75631295387255548, -15.99499920034263489 ) ) ;
#5196=CARTESIAN_POINT ( 'NONE',  ( 12.02805304935487563, 9.316025821727821565, -16.69133030147860453 ) ) ;
#5199=CARTESIAN_POINT ( 'NONE',  ( 36.02474454408307736, -19.83113812547715682, -20.43161669954002591 ) ) ;
#5200=CARTESIAN_POINT ( 'NONE',  ( 16.07247723200118372, 10.90037199175087324, -15.55898442674143745 ) ) ;
#5201=CARTESIAN_POINT ( 'NONE',  ( 27.01132674553606350, -11.00696853675122711, -18.49859303458091730 ) ) ;
#5207=CARTESIAN_POINT ( 'NONE',  ( 34.06228043176686526, -11.34293828116054037, -19.64761387034043949 ) ) ;
#5208=CARTESIAN_POINT ( 'NONE',  ( 22.34502977332646978, 2.679400364154326919, -18.33342593408658061 ) ) ;
#5209=CARTESIAN_POINT ( 'NONE',  ( 27.28761988882141765, -9.265112451392095494, -14.04413049427448001 ) ) ;
#5219=CARTESIAN_POINT ( 'NONE',  ( 12.24452513275510235, 9.643158527868859409, -15.32408204131529317 ) ) ;
#5223=CARTESIAN_POINT ( 'NONE',  ( 12.50906579366657390, 8.574708520419219937, -15.12294941509656354 ) ) ;
#5225=CARTESIAN_POINT ( 'NONE',  ( 16.80134558234102471, 1.491865220098682387, -17.16076555717535257 ) ) ;
#5231=CARTESIAN_POINT ( 'NONE',  ( 11.27599706080618525, 16.67780739407118062, -16.78460567626121502 ) ) ;
#5233=CARTESIAN_POINT ( 'NONE',  ( 35.35024494905714221, -20.29343902266242239, -19.25407150246939736 ) ) ;
#5234=CARTESIAN_POINT ( 'NONE',  ( 16.89369580670022941, 0.5033910033923695293, -17.32063897790030893 ) ) ;
#5238=CARTESIAN_POINT ( 'NONE',  ( 9.117643650280985668, 16.15792227874146292, -17.05261013695411165 ) ) ;
#5239=CARTESIAN_POINT ( 'NONE',  ( 23.25962485557060688, -10.00107805802020167, -16.29084171305886386 ) ) ;
#5242=CARTESIAN_POINT ( 'NONE',  ( 17.94193213664724951, 0.5400182743772068417, -16.55803501089447849 ) ) ;
#5244=CARTESIAN_POINT ( 'NONE',  ( 18.17852402710872894, 9.427450501112501158, -16.79750701094832266 ) ) ;
#5260=CARTESIAN_POINT ( 'NONE',  ( 11.47276097331165623, 9.269810413962238371, -15.86095999428340697 ) ) ;
#5261=CARTESIAN_POINT ( 'NONE',  ( 27.97039215263694345, -10.38370070276099710, -17.82092013489567606 ) ) ;
#5262=CARTESIAN_POINT ( 'NONE',  ( 24.70156281743647142, 0.04986695427254615731, -17.03102378627558977 ) ) ;
#5263=CARTESIAN_POINT ( 'NONE',  ( 31.15806985163746390, -10.82494328065958911, -14.16671120874331358 ) ) ;
#5271=CARTESIAN_POINT ( 'NONE',  ( 21.41025690189560748, 5.821651141963339882, -16.00656683556521998 ) ) ;
#5274=CARTESIAN_POINT ( 'NONE',  ( 10.66955227599643408, 16.86618481130757630, -15.98952479117537173 ) ) ;
#5277=CARTESIAN_POINT ( 'NONE',  ( 20.51249478307574847, 1.942573248051725709, -13.31196225760961838 ) ) ;
#5278=CARTESIAN_POINT ( 'NONE',  ( 17.55932102202221046, 11.64018535857498193, -15.95102284318303276 ) ) ;
#5280=CARTESIAN_POINT ( 'NONE',  ( 32.52799721746220740, -11.03300674309804386, -18.03857687357939099 ) ) ;
#5281=CARTESIAN_POINT ( 'NONE',  ( 20.39818463913025681, -2.063888138892570723, -16.18016139629216354 ) ) ;
#5282=CARTESIAN_POINT ( 'NONE',  ( 19.90313213008900206, 2.415960287222779890, -14.54935787103550560 ) ) ;
#5285=CARTESIAN_POINT ( 'NONE',  ( 29.44447141382201139, -6.373630389881236091, -17.32815070419105297 ) ) ;
#5299=CARTESIAN_POINT ( 'NONE',  ( 35.97124720801268438, -19.59080293283771823, -20.41544573823858144 ) ) ;
#5300=CARTESIAN_POINT ( 'NONE',  ( 12.76023694501680517, 7.627675785621035764, -14.92276157399860281 ) ) ;
#5303=CARTESIAN_POINT ( 'NONE',  ( 12.02748425217687789, 9.318634685891279190, -16.69156549717016702 ) ) ;
#5314=CARTESIAN_POINT ( 'NONE',  ( 11.22387317355479475, 9.091340879052031809, -17.24161325043666082 ) ) ;
#5315=CARTESIAN_POINT ( 'NONE',  ( 25.84319962709097140, -7.021413190281159622, -18.98986798778381058 ) ) ;
#5316=CARTESIAN_POINT ( 'NONE',  ( 23.07678757892180244, -0.1267571646896241688, -14.23703129728563965 ) ) ;
#5334=CARTESIAN_POINT ( 'NONE',  ( 12.02805304935487563, 9.316025821727821565, -16.69133030147860453 ) ) ;
#5336=CARTESIAN_POINT ( 'NONE',  ( 32.68951927270060764, -11.07419627511998605, -18.48540492261787449 ) ) ;
#5338=CARTESIAN_POINT ( 'NONE',  ( 13.38138208201938895, 7.626735917299793499, -15.70646184538344770 ) ) ;
#5340=CARTESIAN_POINT ( 'NONE',  ( 25.73595588610537277, -4.826321120321507507, -18.84379041344559269 ) ) ;
#5341=CARTESIAN_POINT ( 'NONE',  ( 12.31353044564305499, 11.91954703646417713, -16.35554902986205761 ) ) ;
#5344=CARTESIAN_POINT ( 'NONE',  ( 11.34314632229486364, 9.864239995495806212, -15.91456019135469013 ) ) ;
#5346=CARTESIAN_POINT ( 'NONE',  ( 9.917332382238186028, 16.40320447359955125, -16.50418441153501448 ) ) ;
#5351=CARTESIAN_POINT ( 'NONE',  ( 12.02710433905669341, 9.320377015888107408, -16.69172260460959478 ) ) ;
#5354=CARTESIAN_POINT ( 'NONE',  ( 34.13391181137448882, -12.33661648534566524, -20.90239171999057888 ) ) ;
#5355=CARTESIAN_POINT ( 'NONE',  ( 15.47706244943930010, 8.830671366982906889, -20.22835218371243471 ) ) ;
#5356=CARTESIAN_POINT ( 'NONE',  ( 17.20878921875063838, 11.12208594754616975, -17.23123872766219833 ) ) ;
#5364=CARTESIAN_POINT ( 'NONE',  ( 17.81405000127377747, 1.596365152898254980, -17.08637312321770096 ) ) ;
#5365=CARTESIAN_POINT ( 'NONE',  ( 15.70491959545049987, 3.570626008024105680, -15.63470537622339229 ) ) ;
#5377=CARTESIAN_POINT ( 'NONE',  ( 12.21210587983259366, 9.791837354264822935, -15.33748854281299323 ) ) ;
#5381=CARTESIAN_POINT ( 'NONE',  ( 11.50832337395308436, 9.139936167900076569, -15.84372008594036885 ) ) ;
#5382=CARTESIAN_POINT ( 'NONE',  ( 16.25879716139461095, 4.256374150336979412, -17.55500201710977137 ) ) ;
#5388=CARTESIAN_POINT ( 'NONE',  ( 12.83223741744420288, 9.540690758033102625, -16.14104544935691976 ) ) ;
#5390=CARTESIAN_POINT ( 'NONE',  ( 35.32370156268159178, -20.17419364810216109, -19.24765216636316723 ) ) ;
#5392=CARTESIAN_POINT ( 'NONE',  ( 17.66155849027303049, 7.702290371990539342, -14.74052880078125760 ) ) ;
#5395=CARTESIAN_POINT ( 'NONE',  ( 14.50439321891314925, 5.533609182599570353, -15.17065254761420512 ) ) ;
#5400=CARTESIAN_POINT ( 'NONE',  ( 20.49605984403359216, -1.259233478192978373, -14.44550164344372511 ) ) ;
#5401=CARTESIAN_POINT ( 'NONE',  ( 18.26505246421942275, 9.297698622231314047, -17.43849025199569169 ) ) ;
#5413=CARTESIAN_POINT ( 'NONE',  ( 11.50832337395308436, 9.139936167900076569, -15.84372008594036885 ) ) ;
#5414=CARTESIAN_POINT ( 'NONE',  ( 25.59095072769168766, -7.385909681514642777, -13.40699837787023618 ) ) ;
#5415=CARTESIAN_POINT ( 'NONE',  ( 30.27313844582349489, -8.115497507854934511, -14.41531361995715876 ) ) ;
#5416=CARTESIAN_POINT ( 'NONE',  ( 35.54859390953724585, -23.18451583373416014, -16.94733705004010105 ) ) ;
#5424=CARTESIAN_POINT ( 'NONE',  ( 17.36512755686010934, 0.5347363583120325892, -15.24149349723765390 ) ) ;
#5426=CARTESIAN_POINT ( 'NONE',  ( 12.27567800861033120, 9.500287468128719937, -15.31119923128196625 ) ) ;
#5429=CARTESIAN_POINT ( 'NONE',  ( 17.18819971663578272, 0.8441372818425427749, -18.45219435416397502 ) ) ;
#5430=CARTESIAN_POINT ( 'NONE',  ( 13.23210690081759111, 9.952263081781872245, -14.54667289943505004 ) ) ;
#5432=CARTESIAN_POINT ( 'NONE',  ( 33.47012763672258728, -12.84706786418751534, -19.72967806864707541 ) ) ;
#5435=CARTESIAN_POINT ( 'NONE',  ( 0.000000000000000000, 0.000000000000000000, 0.000000000000000000 ) ) ;
#5436=CARTESIAN_POINT ( 'NONE',  ( 24.24063474714532873, -9.755679120534059834, -13.19378374426895206 ) ) ;
#5439=CARTESIAN_POINT ( 'NONE',  ( 17.06466135374324011, 3.680263393506696179, -18.28590298471088005 ) ) ;
#5450=CARTESIAN_POINT ( 'NONE',  ( 36.30362226317071617, -21.08398799169651738, -20.22680612736627026 ) ) ;
#5451=CARTESIAN_POINT ( 'NONE',  ( 9.915973561396301150, 16.40943619918981256, -16.50475030878699556 ) ) ;
#5454=CARTESIAN_POINT ( 'NONE',  ( 13.01452397926061089, 8.532813591658360508, -15.99807864679971026 ) ) ;
#5464=CARTESIAN_POINT ( 'NONE',  ( 13.31307029362551475, 7.598550302509940124, -15.76075481184169647 ) ) ;
#5467=CARTESIAN_POINT ( 'NONE',  ( 15.41555982967951444, 8.269517134526982005, -21.14450021912286104 ) ) ;
#5469=CARTESIAN_POINT ( 'NONE',  ( 26.68716238812262631, -2.792712658874448639, -18.04699283665395981 ) ) ;
#5481=CARTESIAN_POINT ( 'NONE',  ( 10.47212132250356120, 16.45172734403231729, -17.33476278219207956 ) ) ;
#5482=CARTESIAN_POINT ( 'NONE',  ( 35.54502023521215648, -22.16846120802060938, -18.59538644662325524 ) ) ;
#5484=CARTESIAN_POINT ( 'NONE',  ( 8.944584683310379702, 16.95159276115599667, -17.91752729848688830 ) ) ;
#5486=CARTESIAN_POINT ( 'NONE',  ( 26.87257363757477435, -3.324124212371978082, -16.68573618535388547 ) ) ;
#5487=CARTESIAN_POINT ( 'NONE',  ( 12.86785267122296794, 9.515866005961482799, -16.11575320936711364 ) ) ;
#5491=CARTESIAN_POINT ( 'NONE',  ( 11.47288049726737214, 9.269262779257836371, -15.86091052746238184 ) ) ;
#5493=CARTESIAN_POINT ( 'NONE',  ( 12.43696608443014284, 8.546664718661613591, -15.18012293544581226 ) ) ;
#5498=CARTESIAN_POINT ( 'NONE',  ( 12.02859841272590735, 9.313533661810568631, -16.69110409223909741 ) ) ;
#5501=CARTESIAN_POINT ( 'NONE',  ( 36.40320260674921116, -22.53134972621836241, -20.30234751949853589 ) ) ;
#5502=CARTESIAN_POINT ( 'NONE',  ( 29.66490191837812773, -8.365349891895018430, -17.62461620872172574 ) ) ;
#5503=CARTESIAN_POINT ( 'NONE',  ( 15.47706244943930010, 8.830671366982906889, -20.22835218371243471 ) ) ;
#5515=CARTESIAN_POINT ( 'NONE',  ( 21.26848695057635297, 1.468789200266592099, -19.53654423682621299 ) ) ;
#5516=CARTESIAN_POINT ( 'NONE',  ( 17.78594395145776019, 10.14170102421038422, -17.68001733040774681 ) ) ;
#5524=CARTESIAN_POINT ( 'NONE',  ( 12.27630411038995106, 9.497004473356668086, -15.31097170929839812 ) ) ;
#5528=CARTESIAN_POINT ( 'NONE',  ( 12.52778158092594474, 8.582979361647906202, -15.10803260229456946 ) ) ;
#5531=CARTESIAN_POINT ( 'NONE',  ( 17.18298215709098287, 1.908350159885260799, -18.42911670940388902 ) ) ;
#5539=CARTESIAN_POINT ( 'NONE',  ( 12.83236877538120524, 9.540106609504201529, -16.14098973436422568 ) ) ;
#5540=CARTESIAN_POINT ( 'NONE',  ( 34.75280465199809043, -13.11698595563971459, -19.00481823564506101 ) ) ;
#5541=CARTESIAN_POINT ( 'NONE',  ( 15.94478687392618355, 4.193953704849600506, -19.05305658475056063 ) ) ;
#5548=CARTESIAN_POINT ( 'NONE',  ( 17.27944038698359464, 10.59897317215052226, -14.78577975581568360 ) ) ;
#5554=CARTESIAN_POINT ( 'NONE',  ( 26.84208138670940968, -2.489200896322508516, -17.35162900556907317 ) ) ;
#5555=CARTESIAN_POINT ( 'NONE',  ( 18.23559491442917135, -2.176271773050306724, -15.57877364869929515 ) ) ;
#5563=CARTESIAN_POINT ( 'NONE',  ( 11.48890098693651396, 9.204103201752445784, -15.85365151319587440 ) ) ;
#5564=CARTESIAN_POINT ( 'NONE',  ( 28.68006932781580076, -6.484681432979621185, -16.07205306641353104 ) ) ;
#5565=CARTESIAN_POINT ( 'NONE',  ( 28.56280713547801398, -4.978584871567802494, -14.74258920993753641 ) ) ;
#5567=CARTESIAN_POINT ( 'NONE',  ( 34.99076264053043417, -20.67847543353016349, -21.19169145379677488 ) ) ;
#5575=CARTESIAN_POINT ( 'NONE',  ( 21.63873165585565417, 2.424707942738766331, -13.54651715722292060 ) ) ;
#5578=CARTESIAN_POINT ( 'NONE',  ( 12.26883957244698387, 9.531649408071682927, -15.31402716519172635 ) ) ;
#5579=CARTESIAN_POINT ( 'NONE',  ( 32.89062095351589932, -11.25267498498577723, -18.96775996542842435 ) ) ;
#5581=CARTESIAN_POINT ( 'NONE',  ( 25.45462155318426767, -0.2439708902934435431, -15.99927030562601438 ) ) ;
#5583=CARTESIAN_POINT ( 'NONE',  ( 22.15888525254269581, 3.701285330253634154, -19.09944157575669621 ) ) ;
#5586=CARTESIAN_POINT ( 'NONE',  ( 33.37634376253905089, -12.42895282922877342, -19.69946502924221932 ) ) ;
#5588=CARTESIAN_POINT ( 'NONE',  ( 25.30932029414111284, -7.960302465696846852, -19.79224777486898645 ) ) ;
#5589=CARTESIAN_POINT ( 'NONE',  ( 23.51547714073238282, 0.8170344765809651744, -13.87895193235286051 ) ) ;
#5590=CARTESIAN_POINT ( 'NONE',  ( 24.52797215547132836, -1.897736678990579184, -19.26084780660264073 ) ) ;
#5601=CARTESIAN_POINT ( 'NONE',  ( 34.31936231504242585, -12.17391896401218609, -19.91370162440023250 ) ) ;
#5602=CARTESIAN_POINT ( 'NONE',  ( 9.949118446627077006, 16.25742953053141804, -16.49103975576934644 ) ) ;
#5607=CARTESIAN_POINT ( 'NONE',  ( 12.02710433905669341, 9.320377015888107408, -16.69172260460959478 ) ) ;
#5617=CARTESIAN_POINT ( 'NONE',  ( 11.19157713609530269, 9.239454617397717229, -17.25496879848155629 ) ) ;
#5619=CARTESIAN_POINT ( 'NONE',  ( 28.46611200899306127, -11.40119892829609327, -11.67154496650716666 ) ) ;
#5620=CARTESIAN_POINT ( 'NONE',  ( 19.60850488237918654, -1.635242255716521820, -15.65509664672261003 ) ) ;
#5633=CARTESIAN_POINT ( 'NONE',  ( 13.13063628947021755, 8.573956625762026107, -15.90631066800904669 ) ) ;
#5637=CARTESIAN_POINT ( 'NONE',  ( 33.29128644620831778, -11.81988703332123691, -18.18190324972602667 ) ) ;
#5639=CARTESIAN_POINT ( 'NONE',  ( 9.084523633786250940, 16.30981489620654301, -17.07623073379102507 ) ) ;
#5643=CARTESIAN_POINT ( 'NONE',  ( 24.36497833745277930, -6.082191617938494055, -18.74521747929614435 ) ) ;
#5644=CARTESIAN_POINT ( 'NONE',  ( 12.83250652484248633, 9.539529735957493983, -16.14092858578357337 ) ) ;
#5649=CARTESIAN_POINT ( 'NONE',  ( 11.82447321682112751, 8.672047275158794477, -15.63808403058127006 ) ) ;
#5654=CARTESIAN_POINT ( 'NONE',  ( 12.02835731808789355, 9.314632867394664117, -16.69120428796748357 ) ) ;
#5657=CARTESIAN_POINT ( 'NONE',  ( 14.45328171724474231, 7.053988074037379263, -14.59236433646538522 ) ) ;
#5658=CARTESIAN_POINT ( 'NONE',  ( 13.93547621865856634, 6.828337171336619882, -15.16703734247451507 ) ) ;
#5662=CARTESIAN_POINT ( 'NONE',  ( 36.54859390954303677, -22.18451583373416014, -15.55638201429745848 ) ) ;
#5664=CARTESIAN_POINT ( 'NONE',  ( 19.31105547890425100, 3.022890346832332042, -18.89353813576326857 ) ) ;
#5665=CARTESIAN_POINT ( 'NONE',  ( 14.29829396236512729, 6.476847147513518088, -18.28004444394726491 ) ) ;
#5672=CARTESIAN_POINT ( 'NONE',  ( 13.52175692454036415, 9.804829592035652297, -15.59458061810998331 ) ) ;
#5677=CARTESIAN_POINT ( 'NONE',  ( 12.27693553943969818, 9.494520259125854622, -15.31067919898749352 ) ) ;
#5680=CARTESIAN_POINT ( 'NONE',  ( 31.81434894052502571, -10.04473835610349397, -15.03854332269495764 ) ) ;
#5683=CARTESIAN_POINT ( 'NONE',  ( 11.65548303173490652, 8.849831895876286936, -15.75351705932409985 ) ) ;
#5685=CARTESIAN_POINT ( 'NONE',  ( 11.89457502915311160, 7.563359933683480918, -15.58843798323820096 ) ) ;
#5692=CARTESIAN_POINT ( 'NONE',  ( 12.83250652484248633, 9.539529735957493983, -16.14092858578357337 ) ) ;
#5693=CARTESIAN_POINT ( 'NONE',  ( 33.85795792134603488, -11.10969635406632072, -17.56389463281766439 ) ) ;
#5694=CARTESIAN_POINT ( 'NONE',  ( 15.78240017141095741, 4.038647184180326200, -18.77507866864583619 ) ) ;
#5697=CARTESIAN_POINT ( 'NONE',  ( 20.01918758985507196, 7.682949113293006782, -15.97060347488303123 ) ) ;
#5700=CARTESIAN_POINT ( 'NONE',  ( 24.59824444495380646, -5.013944910511990649, -19.70109713935865514 ) ) ;
#5701=CARTESIAN_POINT ( 'NONE',  ( 18.38621934312857320, -2.136830130942094730, -15.12482301043797683 ) ) ;
#5717=CARTESIAN_POINT ( 'NONE',  ( 11.47293561586387867, 9.269010148984008879, -15.86088772249501666 ) ) ;
#5719=CARTESIAN_POINT ( 'NONE',  ( 28.47173825316771101, -6.366402965996883268, -15.18523185298700007 ) ) ;
#5720=CARTESIAN_POINT ( 'NONE',  ( 28.73289915209718615, -4.972737245092835323, -15.12275039236161689 ) ) ;
#5727=CARTESIAN_POINT ( 'NONE',  ( 19.12501085131992085, -2.578449613843157184, -15.80510918775627438 ) ) ;
#5730=CARTESIAN_POINT ( 'NONE',  ( 12.27669453124947552, 9.495625565821059766, -15.31077886340536942 ) ) ;
#5734=CARTESIAN_POINT ( 'NONE',  ( 23.76365953361780470, 2.837943588559999508, -16.54419024451982168 ) ) ;
#5736=CARTESIAN_POINT ( 'NONE',  ( 16.03284225665507279, 2.387151393075086059, -14.54955438622115338 ) ) ;
#5739=CARTESIAN_POINT ( 'NONE',  ( 31.24625831705917278, -7.622123577322120980, -17.00257116200763008 ) ) ;
#5740=CARTESIAN_POINT ( 'NONE',  ( 21.92900763033978251, 0.1816185532145172810, -13.27135403042708717 ) ) ;
#5743=CARTESIAN_POINT ( 'NONE',  ( 29.30346499805017757, -7.722527705200430859, -14.56292402596598556 ) ) ;
#5754=CARTESIAN_POINT ( 'NONE',  ( 14.59671049609067950, 6.266606045730605423, -20.00302036566705155 ) ) ;
#5755=CARTESIAN_POINT ( 'NONE',  ( 35.77509030908504428, -18.70957389315904962, -20.35615221346758474 ) ) ;
#5756=CARTESIAN_POINT ( 'NONE',  ( 11.43229926783177497, 9.455373222906182207, -15.87769231223556332 ) ) ;
#5759=CARTESIAN_POINT ( 'NONE',  ( 9.661958148507006072, 16.25448227554711167, -17.91102859374088752 ) ) ;
#5770=CARTESIAN_POINT ( 'NONE',  ( 13.36280753930113363, 7.618652675320872980, -15.72125653641924892 ) ) ;
#5772=CARTESIAN_POINT ( 'NONE',  ( 30.27995308908331751, -6.828448725465094959, -15.78586218199752622 ) ) ;
#5773=CARTESIAN_POINT ( 'NONE',  ( 29.02390443993225588, -5.138988301204332920, -16.36505798003706857 ) ) ;
#5785=CARTESIAN_POINT ( 'NONE',  ( 13.13233772467555660, 8.574708520419219937, -15.90495459411799395 ) ) ;
#5786=CARTESIAN_POINT ( 'NONE',  ( 35.54859390953724585, -22.18451583373416014, -16.94733705004010460 ) ) ;
#5789=CARTESIAN_POINT ( 'NONE',  ( 9.120682955242472190, 16.14398363876680520, -17.05135327743868245 ) ) ;
#5790=CARTESIAN_POINT ( 'NONE',  ( 25.67262840375075328, -3.322766148301121714, -14.04542551033457798 ) ) ;
#5791=CARTESIAN_POINT ( 'NONE',  ( 13.41286507499157388, 9.756708335562493062, -15.68136934427840856 ) ) ;
#5797=CARTESIAN_POINT ( 'NONE',  ( 12.49860086554322436, 8.570087612320898884, -15.13128986298120537 ) ) ;
#5802=CARTESIAN_POINT ( 'NONE',  ( 12.90142504057275197, 8.513187104919181181, -16.08590544042818493 ) ) ;
#5804=CARTESIAN_POINT ( 'NONE',  ( 17.82530828565625214, 4.245919164363588294, -12.95079069805369443 ) ) ;
#5805=CARTESIAN_POINT ( 'NONE',  ( 20.92570677221209507, 1.074447142478794470, -13.03661572703551919 ) ) ;
#5809=CARTESIAN_POINT ( 'NONE',  ( 36.54779501103016770, -22.18092680593016652, -18.48200341583098449 ) ) ;
#5816=CARTESIAN_POINT ( 'NONE',  ( 17.66155849027303049, 7.702290371990539342, -14.74052880078125760 ) ) ;
#5820=CARTESIAN_POINT ( 'NONE',  ( 33.43446274600908907, -12.68684440242773448, -19.71889742777951327 ) ) ;
#5823=CARTESIAN_POINT ( 'NONE',  ( 12.27669453124947552, 9.495625565821059766, -15.31077886340536942 ) ) ;
#5829=CARTESIAN_POINT ( 'NONE',  ( 12.29195110325218288, 8.516770644378290456, -15.29309475950548958 ) ) ;
#5831=CARTESIAN_POINT ( 'NONE',  ( 12.65299103417153681, 7.585129394224154886, -15.00786874580416530 ) ) ;
#5839=CARTESIAN_POINT ( 'NONE',  ( 12.75119036009696316, 9.912382880115339745, -16.17456125963731850 ) ) ;
#5841=CARTESIAN_POINT ( 'NONE',  ( 36.19723272591463115, -19.60603615691276858, -19.44143419077989421 ) ) ;
#5842=CARTESIAN_POINT ( 'NONE',  ( 18.80472905218952917, 2.352968372735388503, -20.19605574946481497 ) ) ;
#5845=CARTESIAN_POINT ( 'NONE',  ( 17.83091951040035283, 10.74857467630938501, -15.40187535130914753 ) ) ;
#5849=CARTESIAN_POINT ( 'NONE',  ( 24.14852421541024441, 0.2028892341458684023, -15.23052705399570428 ) ) ;
#5851=CARTESIAN_POINT ( 'NONE',  ( 21.72387110042699376, 1.401658020055618792, -20.45241765577301152 ) ) ;
#5866=CARTESIAN_POINT ( 'NONE',  ( 10.95411528722473626, 11.64838591225006859, -16.07543820933196699 ) ) ;
#5867=CARTESIAN_POINT ( 'NONE',  ( 15.70491959545049987, 3.570626008024105680, -15.63470537622339229 ) ) ;
#5868=CARTESIAN_POINT ( 'NONE',  ( 24.51672896724849338, -10.45039314358892035, -14.45231470433035170 ) ) ;
#5878=CARTESIAN_POINT ( 'NONE',  ( 18.04049687913209610, 0.8262538513465327306, -14.27019888128743297 ) ) ;
#5881=CARTESIAN_POINT ( 'NONE',  ( 10.80186837770346919, 16.25936630249904269, -15.92067135797631217 ) ) ;
#5887=CARTESIAN_POINT ( 'NONE',  ( 20.14386580841007657, 1.771853782379294140, -13.30505882909219295 ) ) ;
#5889=CARTESIAN_POINT ( 'NONE',  ( 20.33560388840259137, 1.841519175196629998, -20.14887626749220217 ) ) ;
#5892=CARTESIAN_POINT ( 'NONE',  ( 23.37849240255853189, -5.075553540114302820, -18.86401745356084447 ) ) ;
#5893=CARTESIAN_POINT ( 'NONE',  ( 22.85243615162648112, -7.655412890396200432, -19.01377894019457315 ) ) ;
#5905=CARTESIAN_POINT ( 'NONE',  ( 25.86320101420157158, -8.291784280105535032, -12.84902276017926859 ) ) ;
#5907=CARTESIAN_POINT ( 'NONE',  ( 34.18187006836440389, -11.68445768601494628, -19.79758194388510972 ) ) ;
#5909=CARTESIAN_POINT ( 'NONE',  ( 9.917015787971365626, 16.40465641526357743, -16.50431533440121257 ) ) ;
#5912=CARTESIAN_POINT ( 'NONE',  ( 9.661883061612440926, 16.25482663361732705, -17.95086732675816776 ) ) ;
#5923=CARTESIAN_POINT ( 'NONE',  ( 8.944584683310379702, 16.95159276115599667, -21.33333333332589632 ) ) ;
#5924=CARTESIAN_POINT ( 'NONE',  ( 13.70585326225313771, 5.953887885347688425, -14.73188983601744617 ) ) ;
#5926=CARTESIAN_POINT ( 'NONE',  ( 24.19195398915606532, -10.47609993289601427, -15.85356615136800151 ) ) ;
#5938=CARTESIAN_POINT ( 'NONE',  ( 13.12404665403065707, 8.571044468271947991, -15.91156272984762765 ) ) ;
#5939=CARTESIAN_POINT ( 'NONE',  ( 35.54859390953724585, -22.18451583373416014, -17.64281456791166036 ) ) ;
#5941=CARTESIAN_POINT ( 'NONE',  ( 10.50660601767968139, 9.787963810330234438, -16.47822533839871539 ) ) ;
#5943=CARTESIAN_POINT ( 'NONE',  ( 21.16681283796276603, -5.103637247178538061, -17.00692323485822754 ) ) ;
#5944=CARTESIAN_POINT ( 'NONE',  ( 12.89562877257107054, 9.528132359803098694, -16.09361580714184825 ) ) ;
#5950=CARTESIAN_POINT ( 'NONE',  ( 11.46471852075427478, 9.306694396509932687, -15.86428581073749378 ) ) ;
#5956=CARTESIAN_POINT ( 'NONE',  ( 9.661883061612440926, 16.25482663361732705, -17.91664992932185996 ) ) ;
#5958=CARTESIAN_POINT ( 'NONE',  ( 20.05201200715256249, 8.675301412908657639, -18.33989206490851842 ) ) ;
#5959=CARTESIAN_POINT ( 'NONE',  ( 17.82530828565625214, 4.245919164363588294, -12.95079069805369443 ) ) ;
#5963=CARTESIAN_POINT ( 'NONE',  ( 16.79143122783437292, 7.330551994622505063, -14.54187356113185103 ) ) ;
#5970=CARTESIAN_POINT ( 'NONE',  ( 33.54145741815126058, -13.16751478770765793, -19.75123935038191192 ) ) ;
#5973=CARTESIAN_POINT ( 'NONE',  ( 12.31319128649213646, 9.546177831575306527, -15.27906485473354792 ) ) ;
#5980=CARTESIAN_POINT ( 'NONE',  ( 12.73046782819888989, 7.614823354231524455, -14.94646497050939793 ) ) ;
#5985=CARTESIAN_POINT ( 'NONE',  ( 12.83348778413740376, 9.536125428572121976, -16.14043921975381934 ) ) ;
#5987=CARTESIAN_POINT ( 'NONE',  ( 35.54859390953724585, -21.18451583373416014, -16.11276402859391510 ) ) ;
#5988=CARTESIAN_POINT ( 'NONE',  ( 20.51249478307574847, 1.942573248051725709, -13.31196225760961838 ) ) ;
#5993=CARTESIAN_POINT ( 'NONE',  ( 27.50131297508284334, -11.63919202702402167, -19.74788458503752864 ) ) ;
#5996=CARTESIAN_POINT ( 'NONE',  ( 28.73289915209718615, -4.972737245092835323, -15.12275039236161689 ) ) ;
#5997=CARTESIAN_POINT ( 'NONE',  ( 23.26502027940742678, 3.673231887600847845, -16.77589761210995789 ) ) ;
#6009=CARTESIAN_POINT ( 'NONE',  ( 12.48979292151040177, 7.561326536588189207, -16.39201226339353212 ) ) ;
#6010=CARTESIAN_POINT ( 'NONE',  ( 12.55500454421123457, 8.595009676161804890, -15.08633542003848049 ) ) ;
#6011=CARTESIAN_POINT ( 'NONE',  ( 28.96558774451377971, -5.053040458581501859, -15.93506438242870971 ) ) ;
#6023=CARTESIAN_POINT ( 'NONE',  ( 25.77659985377941254, -6.250509680199615836, -13.67467641272277312 ) ) ;
#6027=CARTESIAN_POINT ( 'NONE',  ( 12.27679999902766284, 9.495116139066881900, -15.31073721177884650 ) ) ;
#6028=CARTESIAN_POINT ( 'NONE',  ( 32.62126879184269512, -11.04717877266006987, -18.30218954475424908 ) ) ;
#6030=CARTESIAN_POINT ( 'NONE',  ( 27.51942754507220812, -5.605608590038333006, -14.64806962472005658 ) ) ;
#6032=CARTESIAN_POINT ( 'NONE',  ( 15.68163020692053422, 2.793964495486057409, -19.44966893625607085 ) ) ;
#6037=CARTESIAN_POINT ( 'NONE',  ( 25.84292692831908766, -2.469955994367391661, -17.24682881138801704 ) ) ;
#6038=CARTESIAN_POINT ( 'NONE',  ( 25.33177305468611351, -7.180647579645999201, -12.45679661262278870 ) ) ;
#6047=CARTESIAN_POINT ( 'NONE',  ( 23.04322939705109974, -6.346999004730295546, -16.23111451206203881 ) ) ;
#6048=CARTESIAN_POINT ( 'NONE',  ( 17.78134717446047119, 9.288666448780150020, -20.14505390916605521 ) ) ;
#6049=CARTESIAN_POINT ( 'NONE',  ( 35.79875902618127270, -19.81590490140210647, -21.40562824699871314 ) ) ;
#6051=CARTESIAN_POINT ( 'NONE',  ( 9.843778300897430000, 16.74053286659246709, -16.57516421589427225 ) ) ;
#6052=EDGE_CURVE ( 'NONE', #22459, #8937, #3432, .T. ) ;
#6058=CARTESIAN_POINT ( 'NONE',  ( 9.661883245193708447, 16.25482579169019459, -17.91553454599451101 ) ) ;
#6061=CARTESIAN_POINT ( 'NONE',  ( 11.45256130090833935, 9.362448956408465861, -15.86931324879919991 ) ) ;
#6068=CARTESIAN_POINT ( 'NONE',  ( 13.38031868501602872, 7.626265983139092874, -15.70730939156535655 ) ) ;
#6069=CARTESIAN_POINT ( 'NONE',  ( 36.54859390953724585, -23.18451583373416014, -17.22552805718784441 ) ) ;
#6070=CARTESIAN_POINT ( 'NONE',  ( 25.08912532741139501, -12.86307741315042108, -14.91192194027685147 ) ) ;
#6071=CARTESIAN_POINT ( 'NONE',  ( 24.27430760268559595, -10.23567508289028716, -17.26834523416827949 ) ) ;
#6082=CARTESIAN_POINT ( 'NONE',  ( 13.15105351193492744, 8.582979361647906202, -15.89003778131599098 ) ) ;
#6083=CARTESIAN_POINT ( 'NONE',  ( 33.61336211056222112, -12.49217533051321993, -18.72970452740151970 ) ) ;
#6084=CARTESIAN_POINT ( 'NONE',  ( 8.965340528640792783, 16.85640380871598509, -17.50303937619785444 ) ) ;
#6088=CARTESIAN_POINT ( 'NONE',  ( 29.72799312938100513, -7.689056491358781997, -15.42978383025728384 ) ) ;
#6090=CARTESIAN_POINT ( 'NONE',  ( 12.86840956200995301, 9.516103707707461723, -16.11530999810414500 ) ) ;
#6096=CARTESIAN_POINT ( 'NONE',  ( 11.46269231744662420, 9.315986823159681407, -15.86512371708112212 ) ) ;
#6101=CARTESIAN_POINT ( 'NONE',  ( 13.12299649507002464, 8.570581087883812899, -15.91239967140973022 ) ) ;
#6103=CARTESIAN_POINT ( 'NONE',  ( 15.09088459799990822, 3.595497735170159803, -19.35696164441904443 ) ) ;
#6104=CARTESIAN_POINT ( 'NONE',  ( 22.44359388949645151, 4.989503210053415572, -18.93028356096972686 ) ) ;
#6107=CARTESIAN_POINT ( 'NONE',  ( 36.13838427452936486, -20.34166123773320578, -20.43658233646779365 ) ) ;
#6109=CARTESIAN_POINT ( 'NONE',  ( 25.57370974413349884, -0.4222200280313516685, -16.88676729435558599 ) ) ;
#6116=CARTESIAN_POINT ( 'NONE',  ( 35.03938282813840743, -19.89690018161999419, -20.20402626681843117 ) ) ;
#6121=CARTESIAN_POINT ( 'NONE',  ( 12.68070129083326236, 9.708587077508630259, -14.98615289428795094 ) ) ;
#6122=CARTESIAN_POINT ( 'NONE',  ( 35.54859125455464408, -23.18450390630307822, -18.42126094939176895 ) ) ;
#6130=CARTESIAN_POINT ( 'NONE',  ( 10.68833914101186444, 8.961267084878116407, -16.40255713880337751 ) ) ;
#6135=CARTESIAN_POINT ( 'NONE',  ( 12.93646321750111916, 9.546177831575306527, -16.06107003375496944 ) ) ;
#6138=CARTESIAN_POINT ( 'NONE',  ( 35.57309713841538468, -16.80212557611773505, -19.25277297559858525 ) ) ;
#6139=CARTESIAN_POINT ( 'NONE',  ( 24.66978787416869068, -0.3063955544261361963, -14.42797892638687784 ) ) ;
#6146=CARTESIAN_POINT ( 'NONE',  ( 26.53548354394225228, -12.81408696708834860, -17.07385457597708367 ) ) ;
#6148=CARTESIAN_POINT ( 'NONE',  ( 19.77054944300549622, 4.331964111641410042, -19.42026316723860901 ) ) ;
#6162=CARTESIAN_POINT ( 'NONE',  ( 11.21386537247953363, 9.137237924250291243, -17.24575182870169598 ) ) ;
#6163=CARTESIAN_POINT ( 'NONE',  ( 12.46899830068120352, 8.557956911948249257, -15.15481108270911825 ) ) ;
#6164=CARTESIAN_POINT ( 'NONE',  ( 26.53548354394225228, -12.81408696708834860, -17.07385457597708367 ) ) ;
#6169=CARTESIAN_POINT ( 'NONE',  ( 9.641350810849047548, 17.66889113945805789, -17.91796598306941135 ) ) ;
#6172=CARTESIAN_POINT ( 'NONE',  ( 23.61827771231835982, -0.6465389018800060672, -13.57143891608981612 ) ) ;
#6175=CARTESIAN_POINT ( 'NONE',  ( 11.05541531668977662, 17.68942339022145305, -17.97192418671890835 ) ) ;
#6179=CARTESIAN_POINT ( 'NONE',  ( 25.77659985377941254, -6.250509680199615836, -13.67467641272277312 ) ) ;
#6181=CARTESIAN_POINT ( 'NONE',  ( 15.35879474092683594, 2.467707791974911302, -18.63256289774529151 ) ) ;
#6183=CARTESIAN_POINT ( 'NONE',  ( 35.54859390954303677, -22.18451583373416014, -15.55638201429745848 ) ) ;
#6185=CARTESIAN_POINT ( 'NONE',  ( 19.14398323884976350, 7.495936751868839565, -14.71076302495156263 ) ) ;
#6187=CARTESIAN_POINT ( 'NONE',  ( 25.20714760837546464, -2.665945389627573991, -12.53535894516201665 ) ) ;
#6192=CARTESIAN_POINT ( 'NONE',  ( 24.60501232743784783, -9.531698448777172317, -16.22453333552994792 ) ) ;
#6200=CARTESIAN_POINT ( 'NONE',  ( 9.641350810849047548, 17.66889113945805789, -17.95086732675817132 ) ) ;
#6201=CARTESIAN_POINT ( 'NONE',  ( 27.30941123812745275, -4.721684434479056947, -15.35818731037458029 ) ) ;
#6202=CARTESIAN_POINT ( 'NONE',  ( 13.93479307118181509, 9.207276677253689812, -14.11477394318545286 ) ) ;
#6203=CARTESIAN_POINT ( 'NONE',  ( 34.69314741404605229, -14.84897758684750890, -21.07142838010442176 ) ) ;
#6206=CARTESIAN_POINT ( 'NONE',  ( 12.46899830068120352, 8.557956911948249257, -15.15481108270911825 ) ) ;
#6209=CARTESIAN_POINT ( 'NONE',  ( 13.19188795686497429, 8.601024833420110483, -15.85749200792911573 ) ) ;
#6213=CARTESIAN_POINT ( 'NONE',  ( 10.17605321708455257, 15.21667774575863419, -16.39719424528293246 ) ) ;
#6219=CARTESIAN_POINT ( 'NONE',  ( 8.944584683310379702, 16.95159276115599667, -17.91752729848688830 ) ) ;
#6220=CARTESIAN_POINT ( 'NONE',  ( 35.69176435403931436, -19.33523451612313693, -21.37328632439622922 ) ) ;
#6221=CARTESIAN_POINT ( 'NONE',  ( 22.63682584648026008, 4.680144189823682410, -16.86151017930854223 ) ) ;
#6222=CARTESIAN_POINT ( 'NONE',  ( 27.50962693642323131, -9.092369620780022643, -12.61635453147917474 ) ) ;
#6227=CARTESIAN_POINT ( 'NONE',  ( 17.76107737582129431, 3.703408080355245158, -15.36634439411934316 ) ) ;
#6238=CARTESIAN_POINT ( 'NONE',  ( 12.22285885739602662, 8.868278133530205665, -16.57678160000113721 ) ) ;
#6239=CARTESIAN_POINT ( 'NONE',  ( 35.40392844931823646, -20.53461055239511879, -19.22110946685632271 ) ) ;
#6241=CARTESIAN_POINT ( 'NONE',  ( 9.057417708256320310, 16.43412612588882027, -17.11704294810955318 ) ) ;
#6244=CARTESIAN_POINT ( 'NONE',  ( 27.44219139316946965, -6.774709612358828181, -18.29578255718776703 ) ) ;
#6245=CARTESIAN_POINT ( 'NONE',  ( 10.35864918915110877, 16.97212501191939538, -17.97192418671891190 ) ) ;
#6255=CARTESIAN_POINT ( 'NONE',  ( 13.23272240178861381, 8.619070305187777947, -15.82494623455082916 ) ) ;
#6256=CARTESIAN_POINT ( 'NONE',  ( 15.83402620853355636, 4.298615461832955731, -20.35054180922590916 ) ) ;
#6257=CARTESIAN_POINT ( 'NONE',  ( 21.88956083454650781, 5.816198478639956093, -14.73130718433538178 ) ) ;
#6262=CARTESIAN_POINT ( 'NONE',  ( 24.92864811393110358, -0.2441600445015326137, -14.78813717129899885 ) ) ;
#6273=CARTESIAN_POINT ( 'NONE',  ( 32.54305136433941215, -11.03529315477374517, -18.08112484791816499 ) ) ;
#6277=CARTESIAN_POINT ( 'NONE',  ( 11.05541531668977662, 17.68942339022145305, -17.97192418671890835 ) ) ;
#6278=CARTESIAN_POINT ( 'NONE',  ( 33.10952763335142635, -11.62914684427059697, -19.38687730282833499 ) ) ;
#6281=CARTESIAN_POINT ( 'NONE',  ( 10.66984875114861886, 9.039338215604900029, -16.41071671300888823 ) ) ;
#6287=CARTESIAN_POINT ( 'NONE',  ( 13.08618951557147803, 9.612344561400664844, -15.94173553134588595 ) ) ;
#6289=CARTESIAN_POINT ( 'NONE',  ( 36.54517214193456454, -21.16914364445853280, -18.53042016804813841 ) ) ;
#6290=CARTESIAN_POINT ( 'NONE',  ( 23.61827771231835982, -0.6465389018800060672, -13.57143891608981612 ) ) ;
#6297=CARTESIAN_POINT ( 'NONE',  ( 28.56280713547801398, -4.978584871567802494, -14.74258920993753641 ) ) ;
#6298=CARTESIAN_POINT ( 'NONE',  ( 26.30156876094583396, -3.312801620251602852, -13.23872229457767169 ) ) ;
#6312=CARTESIAN_POINT ( 'NONE',  ( 11.23176012633392595, 9.056260211165422902, -17.23826859254635835 ) ) ;
#6313=CARTESIAN_POINT ( 'NONE',  ( 13.04501788334644630, 8.811555337407297017, -14.69578613943112799 ) ) ;
#6320=CARTESIAN_POINT ( 'NONE',  ( 9.641351654859628084, 17.66888726871794191, -17.91235298298990841 ) ) ;
#6324=CARTESIAN_POINT ( 'NONE',  ( 22.16846437878366061, -4.107540447007581363, -19.06500358040360865 ) ) ;
#6328=CARTESIAN_POINT ( 'NONE',  ( 12.24562038388194551, 9.516309650702005740, -15.33292062045688908 ) ) ;
#6330=CARTESIAN_POINT ( 'NONE',  ( 33.41663030065195272, -12.60673267154789201, -19.71350710734569134 ) ) ;
#6332=CARTESIAN_POINT ( 'NONE',  ( 27.95388715220626707, -5.541385876428546631, -15.41148221666858831 ) ) ;
#6334=CARTESIAN_POINT ( 'NONE',  ( 20.77099883799555258, -1.523348603316126981, -18.27480029096593839 ) ) ;
#6338=CARTESIAN_POINT ( 'NONE',  ( 16.96387855261641775, 8.441957738943033362, -20.67322241009641814 ) ) ;
#6339=CARTESIAN_POINT ( 'NONE',  ( 29.18140637672732396, -9.206484972055292815, -13.74645275385354815 ) ) ;
#6345=CARTESIAN_POINT ( 'NONE',  ( 29.82081855766934453, -7.722587238354316597, -15.76009366473342332 ) ) ;
#6355=CARTESIAN_POINT ( 'NONE',  ( 26.37829838608531219, -4.974601419860719353, -14.31557877768424092 ) ) ;
#6356=CARTESIAN_POINT ( 'NONE',  ( 20.37871551743239351, 7.600776799596193456, -17.08157252577618479 ) ) ;
#6357=CARTESIAN_POINT ( 'NONE',  ( 32.66938126488236804, -9.629547215342803668, -18.20796273874843507 ) ) ;
#6360=CARTESIAN_POINT ( 'NONE',  ( 11.47304865262203499, 9.268493388164605662, -15.86084085272616484 ) ) ;
#6363=CARTESIAN_POINT ( 'NONE',  ( 9.661883062008595147, 16.25482663180050835, -17.91564816060341769 ) ) ;
#6366=CARTESIAN_POINT ( 'NONE',  ( 10.33811693838771717, 18.38618951776012267, -17.92015940598198753 ) ) ;
#6376=CARTESIAN_POINT ( 'NONE',  ( 8.944586743066221146, 16.95158331485313852, -17.91159992548655566 ) ) ;
#6377=CARTESIAN_POINT ( 'NONE',  ( 32.03687507811291368, -10.31171301082699543, -18.65038288416666390 ) ) ;
#6379=CARTESIAN_POINT ( 'NONE',  ( 16.03284225665507279, 2.387151393075086059, -14.54955438622115338 ) ) ;
#6381=CARTESIAN_POINT ( 'NONE',  ( 30.76698452600511402, -8.440788201038053273, -16.67119366161266925 ) ) ;
#6384=CARTESIAN_POINT ( 'NONE',  ( 24.07185007603571592, -6.521566527568181115, -20.06683206624251525 ) ) ;
#6394=CARTESIAN_POINT ( 'NONE',  ( 33.78268718695997563, -11.09826429569044670, -17.35115476112383348 ) ) ;
#6397=CARTESIAN_POINT ( 'NONE',  ( 10.66878845912243534, 9.044174962973633214, -16.41115715542894193 ) ) ;
#6399=CARTESIAN_POINT ( 'NONE',  ( 25.97851742199650005, -11.98992670343847244, -16.97112261376066655 ) ) ;
#6401=CARTESIAN_POINT ( 'NONE',  ( 10.35864919664826900, 16.97212497753646687, -17.91558149794984445 ) ) ;
#6413=CARTESIAN_POINT ( 'NONE',  ( 15.00903923349565972, 9.404056492746565965, -14.40919036548495669 ) ) ;
#6414=CARTESIAN_POINT ( 'NONE',  ( 21.76882177598054113, -1.089445278190608102, -19.78435629462099854 ) ) ;
#6415=CARTESIAN_POINT ( 'NONE',  ( 19.90219557808113038, 2.290409793443704878, -20.93543687874882053 ) ) ;
#6421=CARTESIAN_POINT ( 'NONE',  ( 18.04049687913209610, 0.8262538513465327306, -14.27019888128743297 ) ) ;
#6427=CARTESIAN_POINT ( 'NONE',  ( 31.62102023406892215, -10.89525581102303420, -15.47516137550896609 ) ) ;
#6431=CARTESIAN_POINT ( 'NONE',  ( 14.03850921439652311, 8.975161913830900673, -15.18271992443145635 ) ) ;
#6432=CARTESIAN_POINT ( 'NONE',  ( 12.24537663854593816, 9.516207477791880365, -15.33311446707169701 ) ) ;
#6433=CARTESIAN_POINT ( 'NONE',  ( 35.54859390953724585, -22.18451583373416014, -17.99055332684694974 ) ) ;
#6437=CARTESIAN_POINT ( 'NONE',  ( 12.75200725638203281, 7.624046516185085665, -14.92932020320056452 ) ) ;
#6445=CARTESIAN_POINT ( 'NONE',  ( 10.35864940629342890, 16.97212401607702148, -17.91464645457531191 ) ) ;
#6446=CARTESIAN_POINT ( 'NONE',  ( 33.54536560287652946, -10.49856191242287373, -18.63199441812703583 ) ) ;
#6447=CARTESIAN_POINT ( 'NONE',  ( 18.98200677837107264, -2.562081333921657933, -16.63161468174866187 ) ) ;
#6451=CARTESIAN_POINT ( 'NONE',  ( 22.24201797625671517, -7.474445146391827777, -15.38054711335415803 ) ) ;
#6452=CARTESIAN_POINT ( 'NONE',  ( 23.18557557936948044, -8.345241077663208884, -16.42592668061853800 ) ) ;
#6457=CARTESIAN_POINT ( 'NONE',  ( 9.641350810849047548, 17.66889113945805789, -23.00000000000000711 ) ) ;
#6461=CARTESIAN_POINT ( 'NONE',  ( 11.06190012440529102, 9.834169922982590961, -17.30859480447365328 ) ) ;
#6462=CARTESIAN_POINT ( 'NONE',  ( 10.33811693838771717, 18.38618951776012267, -17.97192418671890835 ) ) ;
#6463=CARTESIAN_POINT ( 'NONE',  ( 28.40444427461093113, -11.06999723682266179, -18.98653349803348078 ) ) ;
#6467=CARTESIAN_POINT ( 'NONE',  ( 9.644802874473198173, 17.65305953564175567, -17.69767226479352118 ) ) ;
#6471=CARTESIAN_POINT ( 'NONE',  ( 15.60359850163179551, 6.442352727238609411, -18.97839103356167101 ) ) ;
#6475=CARTESIAN_POINT ( 'NONE',  ( 23.29338531092689735, -7.078548041224526521, -17.51562821661096336 ) ) ;
#6480=CARTESIAN_POINT ( 'NONE',  ( 12.25874535991881764, 9.522117202545773651, -15.32245921924925902 ) ) ;
#6481=CARTESIAN_POINT ( 'NONE',  ( 33.47012763672258728, -12.84706786418751534, -19.72967806864707541 ) ) ;
#6483=CARTESIAN_POINT ( 'NONE',  ( 26.72181814967143509, -3.137724904577397389, -15.69709663067708050 ) ) ;
#6485=CARTESIAN_POINT ( 'NONE',  ( 24.85091453934022709, -2.360935040140837771, -14.69038261433388293 ) ) ;
#6488=CARTESIAN_POINT ( 'NONE',  ( 16.94700227795405212, 10.49100606271714931, -14.51747230701220559 ) ) ;
#6489=CARTESIAN_POINT ( 'NONE',  ( 27.29378187812181267, -6.326311925282933402, -12.73600023524891967 ) ) ;
#6501=CARTESIAN_POINT ( 'NONE',  ( 23.72538513773186608, -9.146839435613468794, -15.72061189943629600 ) ) ;
#6502=CARTESIAN_POINT ( 'NONE',  ( 16.03657434348277633, 2.746931742562784162, -16.83325620853174698 ) ) ;
#6503=CARTESIAN_POINT ( 'NONE',  ( 36.19022241692326247, -21.57454255207833071, -21.10101832753974449 ) ) ;
#6505=CARTESIAN_POINT ( 'NONE',  ( 11.47079713067724782, 9.278817116560638567, -15.86177209170659275 ) ) ;
#6508=CARTESIAN_POINT ( 'NONE',  ( 9.748920381043669536, 15.85566239202790406, -17.85155811514292878 ) ) ;
#6514=CARTESIAN_POINT ( 'NONE',  ( 13.04501788334644630, 8.811555337407297017, -14.69578613943112799 ) ) ;
#6522=CARTESIAN_POINT ( 'NONE',  ( 13.44731269622883296, 7.655871835264917102, -15.65391398210326201 ) ) ;
#6523=CARTESIAN_POINT ( 'NONE',  ( 34.81339731023632567, -19.88166695754494384, -21.17803781427711840 ) ) ;
#6524=CARTESIAN_POINT ( 'NONE',  ( 17.99875044999096119, -0.3805832805143671838, -17.40611996466761369 ) ) ;
#6525=CARTESIAN_POINT ( 'NONE',  ( 15.11341857612343809, 8.679638894638937785, -13.66094189273949056 ) ) ;
#6527=CARTESIAN_POINT ( 'NONE',  ( 24.79321154704742725, 0.1008434151899674086, -19.04223803188042652 ) ) ;
#6538=CARTESIAN_POINT ( 'NONE',  ( 34.04598001273328833, -11.17175086900407166, -18.07582794505754364 ) ) ;
#6540=CARTESIAN_POINT ( 'NONE',  ( 11.89457502915311160, 7.563359933683480918, -15.58843798323820096 ) ) ;
#6542=CARTESIAN_POINT ( 'NONE',  ( 27.11191462667604313, -11.78482644060662743, -13.28705938033944989 ) ) ;
#6544=CARTESIAN_POINT ( 'NONE',  ( 11.50940939395034768, 11.69459202490242689, -16.90580767540677343 ) ) ;
#6554=CARTESIAN_POINT ( 'NONE',  ( 13.12553198385420927, 8.571700941790735939, -15.91037888968202552 ) ) ;
#6556=CARTESIAN_POINT ( 'NONE',  ( 20.42254326673722531, -2.835881520377886655, -15.10989100197473789 ) ) ;
#6557=CARTESIAN_POINT ( 'NONE',  ( 19.88518670226333995, -2.923732859705698850, -17.09422515135678111 ) ) ;
#6559=CARTESIAN_POINT ( 'NONE',  ( 18.23802153489769751, 0.9697156596711644649, -18.35043786425562828 ) ) ;
#6564=CARTESIAN_POINT ( 'NONE',  ( 17.96884874826282186, 1.586046385177752871, -19.67104016136476119 ) ) ;
#6579=CARTESIAN_POINT ( 'NONE',  ( 17.66155849027303049, 7.702290371990539342, -14.74052880078125760 ) ) ;
#6580=CARTESIAN_POINT ( 'NONE',  ( 11.05541531668977662, 17.68942339022145305, -17.94384837343789130 ) ) ;
#6581=CARTESIAN_POINT ( 'NONE',  ( 35.54859390953724585, -22.18451583373416014, -18.06010107863414405 ) ) ;
#6584=CARTESIAN_POINT ( 'NONE',  ( 12.76959483864652611, 7.631811206235384226, -14.91530316759754982 ) ) ;
#6590=CARTESIAN_POINT ( 'NONE',  ( 12.86833691348896203, 9.516071730297785081, -16.11536789055087837 ) ) ;
#6591=CARTESIAN_POINT ( 'NONE',  ( 36.54859390953724585, -21.18451583373416014, -17.64281456791166391 ) ) ;
#6592=CARTESIAN_POINT ( 'NONE',  ( 21.18945582756405344, -5.194394521544061227, -16.21196392551894405 ) ) ;
#6596=CARTESIAN_POINT ( 'NONE',  ( 24.19195398915606532, -10.47609993289601427, -15.85356615136800151 ) ) ;
#6597=CARTESIAN_POINT ( 'NONE',  ( 27.85231147893869874, -3.451530096863186792, -17.11803778117090857 ) ) ;
#6608=CARTESIAN_POINT ( 'NONE',  ( 12.52778158092594474, 8.582979361647906202, -15.10803260229456946 ) ) ;
#6613=CARTESIAN_POINT ( 'NONE',  ( 9.641350829061996919, 17.66889105593114806, -17.91548090047172437 ) ) ;
#6615=CARTESIAN_POINT ( 'NONE',  ( 28.93285792728966044, -11.80516759558957673, -13.86517224201260134 ) ) ;
#6619=CARTESIAN_POINT ( 'NONE',  ( 21.79935899731381710, -1.430375723040585356, -13.25318265510616733 ) ) ;
#6623=CARTESIAN_POINT ( 'NONE',  ( 12.27916258238306746, 9.531139938431367753, -15.30618633255685879 ) ) ;
#6625=CARTESIAN_POINT ( 'NONE',  ( 35.13870703111577143, -20.34311121210408757, -20.23074448643712486 ) ) ;
#6627=CARTESIAN_POINT ( 'NONE',  ( 22.34083945069921739, -4.755659482961629436, -14.12236044035638116 ) ) ;
#6629=CARTESIAN_POINT ( 'NONE',  ( 25.80045869113294543, -2.244538201703065283, -16.37342509101419807 ) ) ;
#6632=CARTESIAN_POINT ( 'NONE',  ( 27.15828739042733631, -11.95405637977086677, -19.54710185400437794 ) ) ;
#6633=CARTESIAN_POINT ( 'NONE',  ( 30.81871029749655477, -11.10956723898439868, -14.94490981684777431 ) ) ;
#6649=CARTESIAN_POINT ( 'NONE',  ( 27.00045552667489446, -4.635344809676953837, -19.07524480842047510 ) ) ;
#6650=CARTESIAN_POINT ( 'NONE',  ( 13.86827785273622737, 5.312354197023893221, -16.63408457058017120 ) ) ;
#6651=CARTESIAN_POINT ( 'NONE',  ( 32.85377328814971065, -9.687349299063408026, -18.71178847241494481 ) ) ;
#6654=CARTESIAN_POINT ( 'NONE',  ( 11.47327446659168615, 9.267463859335506982, -15.86074700677745852 ) ) ;
#6655=CIRCLE ( 'NONE', #9552, 0.5000000000000004441 ) ;
#6658=CARTESIAN_POINT ( 'NONE',  ( 9.667904883771802460, 16.22720978959070592, -17.88506087084571305 ) ) ;
#6662=CARTESIAN_POINT ( 'NONE',  ( 12.13006862794127017, 8.527244997094612700, -15.41586291625151972 ) ) ;
#6672=CARTESIAN_POINT ( 'NONE',  ( 9.106918858820071350, 16.20710753947419747, -17.05743340929950946 ) ) ;
#6673=CARTESIAN_POINT ( 'NONE',  ( 35.52699606538937616, -23.08748816067360465, -19.11185354855568619 ) ) ;
#6674=CARTESIAN_POINT ( 'NONE',  ( 19.69411524970139737, 8.437195840132273972, -14.56566581881308409 ) ) ;
#6675=CARTESIAN_POINT ( 'NONE',  ( 19.85258860919307367, 6.732389232436280402, -16.96582824858274208 ) ) ;
#6677=CARTESIAN_POINT ( 'NONE',  ( 27.84123584509972815, -2.508445798277625371, -17.45642919975013285 ) ) ;
#6684=DIRECTION ( 'NONE',  ( -0.06678507476159963041, 0.9947851038922184141, -0.07708664516786083165 ) ) ;
#6692=CARTESIAN_POINT ( 'NONE',  ( 34.98004922032874475, -18.63034571161586683, -19.14376959241974774 ) ) ;
#6694=CARTESIAN_POINT ( 'NONE',  ( 12.54775956925048774, 7.553149829897631840, -15.09063234640338003 ) ) ;
#6696=CARTESIAN_POINT ( 'NONE',  ( 29.46565128511723586, -7.689737916804423534, -14.82739468409561567 ) ) ;
#6698=CARTESIAN_POINT ( 'NONE',  ( 10.46436961932593945, 16.48727764291732711, -17.33901581970886241 ) ) ;
#6709=CARTESIAN_POINT ( 'NONE',  ( 10.70528834225764392, 11.46963701334067842, -17.45606632095149280 ) ) ;
#6712=CARTESIAN_POINT ( 'NONE',  ( 23.66883837772530441, 2.046813550970532969, -14.77838854720118000 ) ) ;
#6713=CARTESIAN_POINT ( 'NONE',  ( 23.59026362060683724, -1.443753810951279082, -14.18444229111703514 ) ) ;
#6714=CARTESIAN_POINT ( 'NONE',  ( 20.13607245741800611, 4.456688099076253629, -14.49627829575511129 ) ) ;
#6717=CARTESIAN_POINT ( 'NONE',  ( 25.31619048431776875, -0.2099727537683927225, -15.56338435260822628 ) ) ;
#6723=CARTESIAN_POINT ( 'NONE',  ( 35.49237112349044310, -21.93193663806729887, -19.32748734164077931 ) ) ;
#6729=CARTESIAN_POINT ( 'NONE',  ( 14.39533340154967433, 6.572929804808670617, -18.54476805420031837 ) ) ;
#6730=CARTESIAN_POINT ( 'NONE',  ( 11.92449941057312124, 13.70369295321711256, -16.51642704783386506 ) ) ;
#6731=CARTESIAN_POINT ( 'NONE',  ( 35.49237112349044310, -21.93193663806729887, -19.32748734164077931 ) ) ;
#6734=CARTESIAN_POINT ( 'NONE',  ( 9.641350810849047548, 17.66889113945805789, -17.92454625180715766 ) ) ;
#6735=CARTESIAN_POINT ( 'NONE',  ( 9.641350835837977584, 17.66889102485563612, -17.91507476468484938 ) ) ;
#6741=CARTESIAN_POINT ( 'NONE',  ( 17.21732962576914616, 11.43796928512929867, -12.64914394394206454 ) ) ;
#6743=CARTESIAN_POINT ( 'NONE',  ( 33.28625081342995884, -10.37305140221732991, -17.94975064729133862 ) ) ;
#6744=CARTESIAN_POINT ( 'NONE',  ( 24.43075134246613800, -6.859861339260811874, -14.00379227226492951 ) ) ;
#6751=CARTESIAN_POINT ( 'NONE',  ( 15.92010713857317938, 6.231155140105813395, -20.15531274222559333 ) ) ;
#6753=CARTESIAN_POINT ( 'NONE',  ( 20.36141319467227362, -5.793038086071195636, -16.11598603859005507 ) ) ;
#6761=CARTESIAN_POINT ( 'NONE',  ( 10.76134431155039373, 16.44521483549405971, -15.93742948484896615 ) ) ;
#6767=CARTESIAN_POINT ( 'NONE',  ( 9.641350810849047548, 17.66889113945805789, -17.92015940598198753 ) ) ;
#6768=CARTESIAN_POINT ( 'NONE',  ( 17.65249788084269511, 8.387921445357553907, -19.05198057976592452 ) ) ;
#6771=CARTESIAN_POINT ( 'NONE',  ( 28.16462234717350199, -5.661059359726887230, -16.30864077692347536 ) ) ;
#6776=CARTESIAN_POINT ( 'NONE',  ( 12.26214823032917778, 9.523620991859985452, -15.31974707146758341 ) ) ;
#6780=CARTESIAN_POINT ( 'NONE',  ( 35.37764311538968087, -21.41652447078215005, -19.89511094362359955 ) ) ;
#6786=CARTESIAN_POINT ( 'NONE',  ( 20.82085833995528290, -1.902372073343062908, -15.34044165217533617 ) ) ;
#6789=( NAMED_UNIT ( * ) PLANE_ANGLE_UNIT ( ) SI_UNIT ( $, .RADIAN. ) );
#6790=CARTESIAN_POINT ( 'NONE',  ( 13.15390973649967599, 8.859676595473322536, -14.60899741038990562 ) ) ;
#6791=CARTESIAN_POINT ( 'NONE',  ( 28.34689840388910653, -5.967659833748593101, -13.48819167749268644 ) ) ;
#6803=CARTESIAN_POINT ( 'NONE',  ( 25.92522129715230506, 0.6472387150544522960, -15.98534533675435299 ) ) ;
#6804=CARTESIAN_POINT ( 'NONE',  ( 17.40782953567980229, 3.270613820851801190, -14.52895612053623609 ) ) ;
#6805=CARTESIAN_POINT ( 'NONE',  ( 36.54859682288668665, -23.18452892187019643, -18.24988411864624993 ) ) ;
#6806=CARTESIAN_POINT ( 'NONE',  ( 11.49350937636955372, 9.187954247928445284, -15.85136552863131421 ) ) ;
#6809=CARTESIAN_POINT ( 'NONE',  ( 9.662182123323882266, 16.25345509848694547, -17.90638241064055336 ) ) ;
#6814=CARTESIAN_POINT ( 'NONE',  ( 12.49271550807400999, 8.567542729147559655, -15.13597632865050535 ) ) ;
#6823=ADVANCED_FACE ( 'NONE', ( #15664 ), #4224, .F. ) ;
#6827=CARTESIAN_POINT ( 'NONE',  ( 9.113591243665672081, 16.17650713204097102, -17.05428594964136835 ) ) ;
#6828=CARTESIAN_POINT ( 'NONE',  ( 32.84381624265927968, -11.41053889131397980, -20.36336433681493929 ) ) ;
#6829=CARTESIAN_POINT ( 'NONE',  ( 21.03983889671009422, 4.536326888612346231, -13.89983168792289270 ) ) ;
#6830=CARTESIAN_POINT ( 'NONE',  ( 19.47111902912460124, 6.782054727477878409, -15.90798308235397407 ) ) ;
#6832=CARTESIAN_POINT ( 'NONE',  ( 26.15289264771154620, -4.614421047071551207, -20.21764904625508663 ) ) ;
#6844=CARTESIAN_POINT ( 'NONE',  ( 35.53758243340352863, -21.13504710440451007, -18.64505253599016044 ) ) ;
#6845=CARTESIAN_POINT ( 'NONE',  ( 11.03967536873724242, 8.192193740582544237, -16.19303379925286279 ) ) ;
#6849=CARTESIAN_POINT ( 'NONE',  ( 10.35870477237433818, 16.97187010017241349, -17.89775757279876700 ) ) ;
#6863=CARTESIAN_POINT ( 'NONE',  ( 9.666286124033039329, 16.23463362809610899, -17.88661257689534878 ) ) ;
#6865=CARTESIAN_POINT ( 'NONE',  ( 22.25649556587329414, -4.532042753231527499, -15.61575944733927024 ) ) ;
#6866=CARTESIAN_POINT ( 'NONE',  ( 22.01749846045582970, -4.595750957016929483, -16.30794181244783303 ) ) ;
#6867=CARTESIAN_POINT ( 'NONE',  ( 22.84118038848623655, 1.850029439873439152, -18.07216660426987431 ) ) ;
#6871=CARTESIAN_POINT ( 'NONE',  ( 21.69765170278760280, -5.035756590920279940, -14.89200278627170881 ) ) ;
#6880=CARTESIAN_POINT ( 'NONE',  ( 10.45680941692980959, 16.52194969480735764, -17.34528143170414083 ) ) ;
#6887=CARTESIAN_POINT ( 'NONE',  ( 16.53342136567307108, 10.04554801986687629, -15.32032680638607047 ) ) ;
#6888=CARTESIAN_POINT ( 'NONE',  ( 11.05542208158282769, 17.68939236555957706, -17.90700183802944778 ) ) ;
#6889=CARTESIAN_POINT ( 'NONE',  ( 35.54859390953724585, -22.18451583373416014, -17.22552805718784441 ) ) ;
#6893=CARTESIAN_POINT ( 'NONE',  ( 9.641364314812712166, 17.66882920855936590, -17.90209449470656722 ) ) ;
#6894=CARTESIAN_POINT ( 'NONE',  ( 13.02821298986966703, 7.746099194123166498, -14.70917993614958519 ) ) ;
#6900=CARTESIAN_POINT ( 'NONE',  ( 11.37973238226026318, 12.28930733048782642, -16.95943368139929319 ) ) ;
#6902=CARTESIAN_POINT ( 'NONE',  ( 36.54859390953724585, -21.18451583373416014, -17.99055332684694974 ) ) ;
#6904=CARTESIAN_POINT ( 'NONE',  ( 26.31132954256896639, -3.159408024760113509, -14.81636702655834803 ) ) ;
#6908=CARTESIAN_POINT ( 'NONE',  ( 17.37262532792671976, 6.041285449496323068, -14.53661901313261495 ) ) ;
#6909=CARTESIAN_POINT ( 'NONE',  ( 23.72497280669020014, -7.722717790116627512, -18.49470058199314693 ) ) ;
#6917=CARTESIAN_POINT ( 'NONE',  ( 10.66955227599643408, 16.86618481130757630, -15.98952479117537173 ) ) ;
#6922=CARTESIAN_POINT ( 'NONE',  ( 10.04637620539468124, 15.81139305134258599, -16.45082025127570091 ) ) ;
#6924=CARTESIAN_POINT ( 'NONE',  ( 15.60254075764268755, 8.625145012302763092, -14.61600764054077395 ) ) ;
#6927=CARTESIAN_POINT ( 'NONE',  ( 28.01381056668970260, -10.10121741814351459, -18.82353034625045041 ) ) ;
#6931=CARTESIAN_POINT ( 'NONE',  ( 11.30853360504539751, 16.52859065474556033, -16.77115057629831441 ) ) ;
#6932=CARTESIAN_POINT ( 'NONE',  ( 35.32886446602115171, -21.19738783794349857, -20.03221113960638178 ) ) ;
#6937=CARTESIAN_POINT ( 'NONE',  ( 23.62051642037636157, -5.854316150849339984, -13.42181569741374503 ) ) ;
#6941=CARTESIAN_POINT ( 'NONE',  ( 19.82332968365342296, 2.432204761014481242, -19.52120720162773537 ) ) ;
#6942=CARTESIAN_POINT ( 'NONE',  ( 27.32534031592636836, -8.675155620653059785, -19.25315075663615971 ) ) ;
#6955=CARTESIAN_POINT ( 'NONE',  ( 9.641566850259106758, 17.66790035518494051, -17.86107206016944460 ) ) ;
#6956=CARTESIAN_POINT ( 'NONE',  ( 24.71165717419137309, -6.805198111665588634, -19.34662478563667065 ) ) ;
#6957=CARTESIAN_POINT ( 'NONE',  ( 21.50147616854745891, 4.214167280306792662, -18.19698480873994839 ) ) ;
#6958=CARTESIAN_POINT ( 'NONE',  ( 31.91112766891453845, -10.28950255622343946, -18.29678896503644481 ) ) ;
#6966=CARTESIAN_POINT ( 'NONE',  ( 10.33811693838771717, 18.38618951776012267, -17.94384837343789130 ) ) ;
#6971=CARTESIAN_POINT ( 'NONE',  ( 18.69974902744413470, 8.051839821468062652, -15.50866580261103955 ) ) ;
#6974=CARTESIAN_POINT ( 'NONE',  ( 32.98128152813007574, -11.80310687477359188, -20.53574887303233609 ) ) ;
#6975=CARTESIAN_POINT ( 'NONE',  ( 22.08459858401872467, -3.550466661657427636, -14.88928395763347723 ) ) ;
#6976=CARTESIAN_POINT ( 'NONE',  ( 16.98323446405135329, 7.186294067752427850, -20.40390978395066313 ) ) ;
#6978=CARTESIAN_POINT ( 'NONE',  ( 27.64540148246904749, -2.072091111371471506, -15.50399641584551702 ) ) ;
#6989=CARTESIAN_POINT ( 'NONE',  ( 32.83462640711407232, -10.30445905196369516, -16.67331141712644538 ) ) ;
#6990=CARTESIAN_POINT ( 'NONE',  ( 12.74005437760208181, 7.618877980503234504, -14.93883819022932080 ) ) ;
#6995=CARTESIAN_POINT ( 'NONE',  ( 10.60167031212029443, 15.85759916399494607, -17.28118971735050735 ) ) ;
#7005=CARTESIAN_POINT ( 'NONE',  ( 9.668188843004273281, 16.22590751635418371, -17.88494344602179709 ) ) ;
#7006=CARTESIAN_POINT ( 'NONE',  ( 21.31799488982693802, -2.441251725956471219, -14.24326171688714204 ) ) ;
#7007=CARTESIAN_POINT ( 'NONE',  ( 22.25649556587329414, -4.532042753231527499, -15.61575944733927024 ) ) ;
#7008=CARTESIAN_POINT ( 'NONE',  ( 21.19231167106929803, 0.1271100694386541607, -19.24388053421374778 ) ) ;
#7012=CARTESIAN_POINT ( 'NONE',  ( 25.67262840375075328, -3.322766148301121714, -14.04542551033457798 ) ) ;
#7023=CARTESIAN_POINT ( 'NONE',  ( 10.35864918915110877, 16.97212501191939538, -17.91664992932186351 ) ) ;
#7025=CARTESIAN_POINT ( 'NONE',  ( 32.00110207675911767, -10.95298233446834502, -16.54939777171900417 ) ) ;
#7027=CARTESIAN_POINT ( 'NONE',  ( 11.22494245711612848, 9.086454032755447940, -17.24116976563960435 ) ) ;
#7030=CARTESIAN_POINT ( 'NONE',  ( 21.63873165585565417, 2.424707942738766331, -13.54651715722292060 ) ) ;
#7031=CARTESIAN_POINT ( 'NONE',  ( 11.09873500484433606, 17.49075377836879497, -17.25232203421226274 ) ) ;
#7035=CARTESIAN_POINT ( 'NONE',  ( 9.641350810849047548, 17.66889113945805789, -17.91664992932186351 ) ) ;
#7038=CARTESIAN_POINT ( 'NONE',  ( 9.641350944112486943, 17.66889052829492002, -17.91441860517739215 ) ) ;
#7044=CARTESIAN_POINT ( 'NONE',  ( 10.47452605456472696, 16.44069893626776491, -17.33376834041267145 ) ) ;
#7046=CARTESIAN_POINT ( 'NONE',  ( 36.54460969663918490, -22.16661687567949457, -18.62492107750662029 ) ) ;
#7047=CARTESIAN_POINT ( 'NONE',  ( 27.83100014064079275, -5.545984359997562230, -15.13782040115233052 ) ) ;
#7051=CARTESIAN_POINT ( 'NONE',  ( 34.41982446195410716, -12.62108234628556680, -19.94648786050102274 ) ) ;
#7053=CARTESIAN_POINT ( 'NONE',  ( 14.24687995347741420, 8.287322832548987606, -13.87414582376881000 ) ) ;
#7054=CARTESIAN_POINT ( 'NONE',  ( 26.77273401934504093, -11.50074486517209138, -16.59227217106661101 ) ) ;
#7063=CARTESIAN_POINT ( 'NONE',  ( 10.72042364955539284, 16.63288220757436164, -15.95435249082810003 ) ) ;
#7068=CARTESIAN_POINT ( 'NONE',  ( 11.44040408106239326, 9.418203516307107392, -15.87434068686103394 ) ) ;
#7070=CARTESIAN_POINT ( 'NONE',  ( 18.03247465133560468, 8.846858265128714649, -18.47062581007826410 ) ) ;
#7073=CARTESIAN_POINT ( 'NONE',  ( 26.38113052396219516, -11.59678093645141672, -17.84452879788985769 ) ) ;
#7076=CARTESIAN_POINT ( 'NONE',  ( 11.27495124880614163, 16.68260362121340279, -16.78505081266910182 ) ) ;
#7077=CARTESIAN_POINT ( 'NONE',  ( 35.54859477393411993, -21.18451971701249548, -18.28760485896911803 ) ) ;
#7082=CARTESIAN_POINT ( 'NONE',  ( 25.92665957894408280, -9.004797978260709712, -12.14503282074142909 ) ) ;
#7086=CARTESIAN_POINT ( 'NONE',  ( 18.75392633456350922, 0.8452085672475394551, -14.97946080469353447 ) ) ;
#7087=CARTESIAN_POINT ( 'NONE',  ( 16.02697758069565381, 6.204487712298734081, -15.55946274640501237 ) ) ;
#7096=CARTESIAN_POINT ( 'NONE',  ( 9.912057827679275235, 16.42739425315605928, -16.50652470164456531 ) ) ;
#7097=CARTESIAN_POINT ( 'NONE',  ( 23.31633574299079825, -8.368445843159939557, -15.61931793633953980 ) ) ;
#7098=CARTESIAN_POINT ( 'NONE',  ( 19.60850488237918654, -1.635242255716521820, -15.65509664672261003 ) ) ;
#7099=CARTESIAN_POINT ( 'NONE',  ( 32.08869746025642655, -10.33200466608398216, -18.78962723441388150 ) ) ;
#7101=CARTESIAN_POINT ( 'NONE',  ( 12.53458732174692258, 8.585986940276173485, -15.10260830673100330 ) ) ;
#7104=CARTESIAN_POINT ( 'NONE',  ( 17.78594395145776019, 10.14170102421038422, -17.68001733040774681 ) ) ;
#7107=CARTESIAN_POINT ( 'NONE',  ( 10.72113683966407294, 16.62961142682532767, -15.95405668885543982 ) ) ;
#7112=CARTESIAN_POINT ( 'NONE',  ( 15.41431293496917121, 3.575304669039410133, -17.09800041271234150 ) ) ;
#7114=CARTESIAN_POINT ( 'NONE',  ( 17.49446177548951553, 10.34313653870878547, -20.19723249710358104 ) ) ;
#7116=CARTESIAN_POINT ( 'NONE',  ( 35.05385823632300912, -20.96193052275466329, -21.15110683048779805 ) ) ;
#7119=CARTESIAN_POINT ( 'NONE',  ( 21.15397186503396654, -1.756306506132798706, -15.01670888948634364 ) ) ;
#7122=CARTESIAN_POINT ( 'NONE',  ( 19.85629768685782537, 6.556105584440964584, -17.58075288388961965 ) ) ;
#7124=CARTESIAN_POINT ( 'NONE',  ( 29.08439603799166306, -5.802884797086306001, -14.52222230071497755 ) ) ;
#7133=CARTESIAN_POINT ( 'NONE',  ( 36.51492826578181194, -21.03327392953103825, -18.93061234292109063 ) ) ;
#7134=CARTESIAN_POINT ( 'NONE',  ( 12.97376706329020557, 7.722038565090276308, -14.75257430067278719 ) ) ;
#7139=CARTESIAN_POINT ( 'NONE',  ( 10.46817501828509123, 16.46982559821503145, -17.33665662920367723 ) ) ;
#7151=CARTESIAN_POINT ( 'NONE',  ( 9.667840685194843076, 16.22750421244806063, -17.88508776754438401 ) ) ;
#7154=CARTESIAN_POINT ( 'NONE',  ( 26.91914097958202845, -7.808663323052361882, -12.67700453112951209 ) ) ;
#7158=CARTESIAN_POINT ( 'NONE',  ( 17.90640022563237110, 0.6078909361919438981, -17.24624654394265377 ) ) ;
#7163=FACE_OUTER_BOUND ( 'NONE', #9097, .T. ) ;
#7165=CARTESIAN_POINT ( 'NONE',  ( 26.18758235895636233, -4.355437658720127558, -18.53605802859044260 ) ) ;
#7173=CARTESIAN_POINT ( 'NONE',  ( 12.02823749386838514, 9.315180647891255106, -16.69125397286443047 ) ) ;
#7175=CARTESIAN_POINT ( 'NONE',  ( 32.30218501430429967, -10.99871056796995816, -17.40035725849610060 ) ) ;
#7177=CARTESIAN_POINT ( 'NONE',  ( 13.36610298980765776, 7.620062051554192806, -15.71863358442526781 ) ) ;
#7180=CARTESIAN_POINT ( 'NONE',  ( 19.61192361542596529, -2.405681417800469291, -14.70675912396028906 ) ) ;
#7181=CARTESIAN_POINT ( 'NONE',  ( 11.26126983089308098, 16.74534834773793790, -16.79273533431442900 ) ) ;
#7185=CARTESIAN_POINT ( 'NONE',  ( 9.641404825192898542, 17.66864342279195199, -17.88841768828662282 ) ) ;
#7187=CARTESIAN_POINT ( 'NONE',  ( 11.39177520167864266, 9.641221755901229429, -15.89445043910815336 ) ) ;
#7193=CARTESIAN_POINT ( 'NONE',  ( 10.48212431696843439, 16.40585233633115436, -17.33062619162406293 ) ) ;
#7195=CARTESIAN_POINT ( 'NONE',  ( 32.76003276007612186, -9.647047962658168885, -18.46200315532429315 ) ) ;
#7196=CARTESIAN_POINT ( 'NONE',  ( 14.55381231002303188, 10.26819836692386723, -15.14301692386319331 ) ) ;
#7197=CARTESIAN_POINT ( 'NONE',  ( 28.06689949639850212, -8.111051215268487269, -13.49421662364394514 ) ) ;
#7203=CARTESIAN_POINT ( 'NONE',  ( 34.21937970685856101, -11.80343312934236089, -19.83772509046166732 ) ) ;
#7205=CARTESIAN_POINT ( 'NONE',  ( 16.27660620799252911, 9.202420196601492464, -13.74949690087879439 ) ) ;
#7206=CARTESIAN_POINT ( 'NONE',  ( 13.77718166750866224, 8.859676595473322536, -15.39100258941132715 ) ) ;
#7216=CARTESIAN_POINT ( 'NONE',  ( 10.72113683966407294, 16.62961142682532767, -15.95405668885543982 ) ) ;
#7221=CARTESIAN_POINT ( 'NONE',  ( 9.917205744531459644, 16.40378525026516243, -16.50423678068149869 ) ) ;
#7224=CARTESIAN_POINT ( 'NONE',  ( 16.31265859067239532, 4.319332383768222705, -17.78589364095596892 ) ) ;
#7227=CARTESIAN_POINT ( 'NONE',  ( 28.15048769591263067, -5.842385520647848551, -16.89978903947823241 ) ) ;
#7230=CARTESIAN_POINT ( 'NONE',  ( 11.27662090294977837, 16.67494637447927275, -16.78434760121053060 ) ) ;
#7233=CARTESIAN_POINT ( 'NONE',  ( 33.19002920664139111, -11.78337016499817658, -17.90800870513906773 ) ) ;
#7237=CARTESIAN_POINT ( 'NONE',  ( 23.31581686446907398, -5.989474659622321617, -13.63887547363156827 ) ) ;
#7242=CARTESIAN_POINT ( 'NONE',  ( 16.95656709563420250, 3.789241241613106048, -19.64973185778705655 ) ) ;
#7243=CARTESIAN_POINT ( 'NONE',  ( 17.65249788084269511, 8.387921445357553907, -19.05198057976592452 ) ) ;
#7253=CARTESIAN_POINT ( 'NONE',  ( 9.641350810849047548, 17.66889113945805789, -17.91752729848689185 ) ) ;
#7255=CARTESIAN_POINT ( 'NONE',  ( 20.69116929084294298, -5.269815114589342819, -18.46063674707264468 ) ) ;
#7256=CARTESIAN_POINT ( 'NONE',  ( 20.55949567978923298, 1.660703385868308235, -14.27713627412184039 ) ) ;
#7258=CARTESIAN_POINT ( 'NONE',  ( 36.54859390953724585, -23.18451583373416014, -17.22552805718784441 ) ) ;
#7262=CARTESIAN_POINT ( 'NONE',  ( 19.25048709941964376, 7.441878894999256921, -18.84525011105569803 ) ) ;
#7264=CARTESIAN_POINT ( 'NONE',  ( 10.33811767156285555, 18.38618615532545064, -17.91197029530843565 ) ) ;
#7268=CARTESIAN_POINT ( 'NONE',  ( 16.57956996521092918, 4.788269978297743812, -19.71382457362092566 ) ) ;
#7270=CARTESIAN_POINT ( 'NONE',  ( 17.86674704105132605, 10.80914456302241788, -19.54358591003751755 ) ) ;
#7272=CARTESIAN_POINT ( 'NONE',  ( 34.39741479528305490, -17.01287786994462792, -20.00997473120332515 ) ) ;
#7274=CARTESIAN_POINT ( 'NONE',  ( 23.28032035799162358, -0.8411909528121862545, -14.99295998388115869 ) ) ;
#7275=CARTESIAN_POINT ( 'NONE',  ( 18.98834166481877972, 4.258514017552020192, -15.11364409576566459 ) ) ;
#7277=CARTESIAN_POINT ( 'NONE',  ( 29.37945295281542712, -10.41679561567529433, -17.92877087918597212 ) ) ;
#7286=CARTESIAN_POINT ( 'NONE',  ( 36.35319451023849524, -20.30668983862152288, -19.44923342519521370 ) ) ;
#7287=CARTESIAN_POINT ( 'NONE',  ( 9.641351021852148762, 17.66889017177091503, -17.91406276888456617 ) ) ;
#7292=CARTESIAN_POINT ( 'NONE',  ( 12.03309083968702886, 9.293808706017943067, -16.68917936036902105 ) ) ;
#7294=AXIS2_PLACEMENT_3D ( 'NONE', #29796, #27477, #6684 ) ;
#7302=CARTESIAN_POINT ( 'NONE',  ( 9.668378799564367299, 16.22503635135577227, -17.88486489230207965 ) ) ;
#7303=CARTESIAN_POINT ( 'NONE',  ( 24.88525782559502630, -5.606924519715485111, -13.99218633471889817 ) ) ;
#7304=CARTESIAN_POINT ( 'NONE',  ( 21.12965431673027794, -4.223434333162931154, -14.75790768142083031 ) ) ;
#7310=CARTESIAN_POINT ( 'NONE',  ( 23.84106988684860440, -4.080291168153947545, -13.50610408985603250 ) ) ;
#7319=CARTESIAN_POINT ( 'NONE',  ( 10.47401950373780899, 16.44302204293020964, -17.33397781699859053 ) ) ;
#7326=CARTESIAN_POINT ( 'NONE',  ( 8.944584683310379702, 16.95159276115599667, -17.95086732675816776 ) ) ;
#7331=CARTESIAN_POINT ( 'NONE',  ( 18.21616227284554057, 4.699354889203569918, -13.86658597208997179 ) ) ;
#7332=CARTESIAN_POINT ( 'NONE',  ( 11.27425361364269563, 16.68580306500076915, -16.78535843524344173 ) ) ;
#7337=CARTESIAN_POINT ( 'NONE',  ( 9.655099948573186097, 17.60583584124798051, -17.48406748397995614 ) ) ;
#7339=CARTESIAN_POINT ( 'NONE',  ( 9.644802874473198173, 17.65305953564175567, -17.69767226479352118 ) ) ;
#7344=CARTESIAN_POINT ( 'NONE',  ( 10.47103768343372288, 16.45669705093847313, -17.33522727542475295 ) ) ;
#7346=CARTESIAN_POINT ( 'NONE',  ( 36.52322468491136220, -22.07054534594105988, -19.04503427665075321 ) ) ;
#7347=CARTESIAN_POINT ( 'NONE',  ( 26.36224721256908410, -8.875037662531589433, -13.49479840426202948 ) ) ;
#7348=CARTESIAN_POINT ( 'NONE',  ( 16.68567729567724456, 11.07888045854852876, -16.17353378320854418 ) ) ;
#7354=CARTESIAN_POINT ( 'NONE',  ( 26.46413748225140594, -13.10274310649288942, -15.24000415025259692 ) ) ;
#7356=CARTESIAN_POINT ( 'NONE',  ( 28.00362220295478721, -7.540254448315821811, -17.98007619878529439 ) ) ;
#7366=UNCERTAINTY_MEASURE_WITH_UNIT (LENGTH_MEASURE( 1.000000000000000082E-05 ), #25150, 'distance_accuracy_value', 'NONE');
#7369=CARTESIAN_POINT ( 'NONE',  ( 10.33811712360892443, 18.38618866831204102, -17.91390369733608523 ) ) ;
#7376=CARTESIAN_POINT ( 'NONE',  ( 9.957223259857686415, 16.22025982393231303, -16.48768813039480818 ) ) ;
#7378=CARTESIAN_POINT ( 'NONE',  ( 9.667856465286563505, 16.22743184293591057, -17.88508098240584587 ) ) ;
#7379=CARTESIAN_POINT ( 'NONE',  ( 17.47084574460127371, 4.633898707001591788, -15.02533140066315198 ) ) ;
#7382=CARTESIAN_POINT ( 'NONE',  ( 27.20760296572909809, -8.488227175050779394, -13.35743234967312354 ) ) ;
#7385=CARTESIAN_POINT ( 'NONE',  ( 11.05545861061968083, 17.68922483874021978, -17.89384690447096560 ) ) ;
#7387=CARTESIAN_POINT ( 'NONE',  ( 33.63121621376239290, -12.57075016180469262, -18.73605167971255980 ) ) ;
#7388=CARTESIAN_POINT ( 'NONE',  ( 16.53304876882650731, 8.555045913257369961, -19.77053526944897754 ) ) ;
#7390=CARTESIAN_POINT ( 'NONE',  ( 9.113211330545484046, 16.17824946203780456, -17.05444305708079966 ) ) ;
#7391=CARTESIAN_POINT ( 'NONE',  ( 25.62874891556376511, -2.832145142407604510, -18.00902499482074148 ) ) ;
#7394=CARTESIAN_POINT ( 'NONE',  ( 20.07445496384854877, 6.874260549971754841, -18.87959640166664954 ) ) ;
#7395=CARTESIAN_POINT ( 'NONE',  ( 18.99253871878172717, 7.061292173911923875, -17.66947577672478431 ) ) ;
#7408=CARTESIAN_POINT ( 'NONE',  ( 9.641351654859628084, 17.66888726871794191, -17.91235298298990841 ) ) ;
#7410=CARTESIAN_POINT ( 'NONE',  ( 27.16844481176636350, -11.11852963900163438, -17.34443814838110143 ) ) ;
#7411=CARTESIAN_POINT ( 'NONE',  ( 20.75491211191951635, -1.144232541536293946, -14.27023797479654554 ) ) ;
#7412=CARTESIAN_POINT ( 'NONE',  ( 33.15841575409167064, -12.44672528413413026, -20.67776857359057274 ) ) ;
#7418=CARTESIAN_POINT ( 'NONE',  ( 14.24706144987486667, 6.238427219560604087, -16.72753349211556184 ) ) ;
#7421=CARTESIAN_POINT ( 'NONE',  ( 10.38540050948072846, 18.16934103347302454, -16.97553146008864289 ) ) ;
#7424=CARTESIAN_POINT ( 'NONE',  ( 14.73401617531889229, 6.408058468588501810, -15.60580005407095960 ) ) ;
#7425=CARTESIAN_POINT ( 'NONE',  ( 30.75621536574076487, -10.42133643238263829, -12.14063830390948517 ) ) ;
#7427=CARTESIAN_POINT ( 'NONE',  ( 32.89062095351589932, -11.25267498498577723, -18.96775996542842435 ) ) ;
#7428=CARTESIAN_POINT ( 'NONE',  ( 21.61496389699315657, -3.514534563429178249, -17.40323974765788506 ) ) ;
#7429=CARTESIAN_POINT ( 'NONE',  ( 18.57704598647189798, -1.039939211366111005, -17.60664924018008293 ) ) ;
#7431=CARTESIAN_POINT ( 'NONE',  ( 27.65280983889778810, -8.379432582749632985, -19.23476105915534973 ) ) ;
#7441=CARTESIAN_POINT ( 'NONE',  ( 36.53496835490201988, -21.12330343441383818, -18.71787618725911884 ) ) ;
#7442=CARTESIAN_POINT ( 'NONE',  ( 9.643509238790151983, 17.65899231378470446, -17.74106871770035099 ) ) ;
#7446=CARTESIAN_POINT ( 'NONE',  ( 12.50603416232391929, 8.608717614871036261, -16.38042650914619358 ) ) ;
#7456=CARTESIAN_POINT ( 'NONE',  ( 11.18347232286468440, 9.276624323996792043, -17.25832042385608389 ) ) ;
#7457=CARTESIAN_POINT ( 'NONE',  ( 23.39779239333391914, -5.936415184958717894, -17.60678703246490429 ) ) ;
#7458=CARTESIAN_POINT ( 'NONE',  ( 20.61437924707763258, -4.384239709691692966, -16.09784705243023240 ) ) ;
#7470=CARTESIAN_POINT ( 'NONE',  ( 10.47325967749744180, 16.44650670292386607, -17.33429203187744250 ) ) ;
#7472=CARTESIAN_POINT ( 'NONE',  ( 35.03938282813840743, -19.89690018161999419, -20.20402626681843117 ) ) ;
#7474=CARTESIAN_POINT ( 'NONE',  ( 13.38031868501602872, 7.626265983139092874, -15.70730939156535655 ) ) ;
#7476=CARTESIAN_POINT ( 'NONE',  ( 21.19279910686179846, 4.720633506281588510, -19.26595127233560234 ) ) ;
#7477=CARTESIAN_POINT ( 'NONE',  ( 12.82818608578791064, 9.559270667424515366, -16.14272081857926366 ) ) ;
#7480=CARTESIAN_POINT ( 'NONE',  ( 11.47395765415086188, 9.264374527449886543, -15.86046114005151075 ) ) ;
#7482=CARTESIAN_POINT ( 'NONE',  ( 9.643509238790151983, 17.65899231378470446, -17.74106871770035099 ) ) ;
#7487=CARTESIAN_POINT ( 'NONE',  ( 10.47193650065820592, 16.45257496057443802, -17.33483926051624735 ) ) ;
#7489=CARTESIAN_POINT ( 'NONE',  ( 31.73602415849877900, -9.487789691486469223, -15.56998832973926916 ) ) ;
#7490=CARTESIAN_POINT ( 'NONE',  ( 14.03447742461322534, 10.03307406631979326, -15.27079475659193086 ) ) ;
#7491=CARTESIAN_POINT ( 'NONE',  ( 14.55381231002303188, 10.26819836692386723, -15.14301692386319331 ) ) ;
#7499=CARTESIAN_POINT ( 'NONE',  ( 19.13053735399196142, -0.4946192386601480084, -18.78456443592403602 ) ) ;
#7501=CARTESIAN_POINT ( 'NONE',  ( 29.32553208039167458, -8.962988822949116141, -16.84503999589972523 ) ) ;
#7502=ADVANCED_FACE ( 'NONE', ( #11935 ), #20655, .T. ) ;
#7509=CARTESIAN_POINT ( 'NONE',  ( 12.27643783485070372, 9.496802808135052842, -15.31088501640310540 ) ) ;
#7513=CARTESIAN_POINT ( 'NONE',  ( 11.47029057985033340, 9.281140223223081520, -15.86198156829250117 ) ) ;
#7515=CARTESIAN_POINT ( 'NONE',  ( 18.89783927354708837, -1.194421563772924078, -19.46960211947776287 ) ) ;
#7521=CARTESIAN_POINT ( 'NONE',  ( 11.29637638519941589, 16.58434521464408817, -16.77617801436024081 ) ) ;
#7523=CARTESIAN_POINT ( 'NONE',  ( 35.50545599541538877, -20.99072003637593653, -18.92103158260024642 ) ) ;
#7524=CARTESIAN_POINT ( 'NONE',  ( 18.69974902744413470, 8.051839821468062652, -15.50866580261103955 ) ) ;
#7526=CARTESIAN_POINT ( 'NONE',  ( 9.128787768473113573, 16.10681393216777835, -17.04800165206417972 ) ) ;
#7527=CARTESIAN_POINT ( 'NONE',  ( 29.60951380729897764, -9.700310021160106544, -19.83312561509874783 ) ) ;
#7532=CARTESIAN_POINT ( 'NONE',  ( 19.92565466131104301, 6.686648131885553958, -19.16379146452587179 ) ) ;
#7534=CARTESIAN_POINT ( 'NONE',  ( 17.24236049518817282, 9.271217979531970244, -15.28210331290996571 ) ) ;
#7548=CARTESIAN_POINT ( 'NONE',  ( 9.641350835837977584, 17.66889102485563612, -17.91507476468484938 ) ) ;
#7549=CARTESIAN_POINT ( 'NONE',  ( 26.65048721414892086, -11.67344998524500355, -15.88597958324129777 ) ) ;
#7550=CARTESIAN_POINT ( 'NONE',  ( 19.39248696316839116, -1.610358169686434193, -16.91126230894791860 ) ) ;
#7551=CARTESIAN_POINT ( 'NONE',  ( 34.92716911317440065, -20.39278340154575631, -21.20741747040485592 ) ) ;
#7558=CARTESIAN_POINT ( 'NONE',  ( 16.34386185847872142, 4.569898679961749366, -19.52586945278800812 ) ) ;
#7561=CARTESIAN_POINT ( 'NONE',  ( 10.41323547201801958, 18.04168634714536168, -16.76531574090561350 ) ) ;
#7564=CARTESIAN_POINT ( 'NONE',  ( 19.25048709941964376, 7.441878894999256921, -18.84525011105569803 ) ) ;
#7565=CARTESIAN_POINT ( 'NONE',  ( 25.64452216564459164, -12.66255397501067570, -13.70049860994083701 ) ) ;
#7567=CARTESIAN_POINT ( 'NONE',  ( 35.16668739017224965, -20.46881214373840763, -20.22602438870426766 ) ) ;
#7568=CARTESIAN_POINT ( 'NONE',  ( 21.82606822486871323, 1.157895394498012154, -14.17951425939655508 ) ) ;
#7570=CARTESIAN_POINT ( 'NONE',  ( 16.83868323617221208, 3.350830693655540315, -16.91447790370928672 ) ) ;
#7574=CARTESIAN_POINT ( 'NONE',  ( 29.25075025305862653, -5.797754334661411768, -14.89650002867986878 ) ) ;
#7582=CARTESIAN_POINT ( 'NONE',  ( 33.68917633736438688, -10.64779379647620949, -18.96437360758372748 ) ) ;
#7583=CARTESIAN_POINT ( 'NONE',  ( 9.641350810849047548, 17.66889113945805789, -17.98596209335946128 ) ) ;
#7587=CARTESIAN_POINT ( 'NONE',  ( 12.98644063677341798, 8.526496012441747041, -16.01999686492960961 ) ) ;
#7597=CARTESIAN_POINT ( 'NONE',  ( 11.23996880139866761, 9.021883543159612273, -17.23462466665071346 ) ) ;
#7598=CARTESIAN_POINT ( 'NONE',  ( 24.17451698631213475, -5.926886182136407832, -14.25952201372300365 ) ) ;
#7600=CARTESIAN_POINT ( 'NONE',  ( 19.39950943988042553, -1.649204456521256246, -16.58530004841527727 ) ) ;
#7614=CARTESIAN_POINT ( 'NONE',  ( 12.02780084644370007, 9.317182744227245905, -16.69143457430396893 ) ) ;
#7616=CARTESIAN_POINT ( 'NONE',  ( 32.45272648307624053, -11.02157468472264412, -17.82583700188536824 ) ) ;
#7618=CARTESIAN_POINT ( 'NONE',  ( 13.37597118643279970, 7.624349635725309327, -15.71077405172158947 ) ) ;
#7620=CARTESIAN_POINT ( 'NONE',  ( 18.97268594440662426, -2.511067197207834667, -17.06021009607598415 ) ) ;
#7621=CARTESIAN_POINT ( 'NONE',  ( 12.86662121207793241, 9.515397394723519753, -16.11672893869402756 ) ) ;
#7625=CARTESIAN_POINT ( 'NONE',  ( 10.95411528722473626, 11.64838591225006859, -16.07543820933196699 ) ) ;
#7628=CARTESIAN_POINT ( 'NONE',  ( 9.926830210242822972, 16.35964622367879784, -16.50025672554925293 ) ) ;
#7633=CARTESIAN_POINT ( 'NONE',  ( 12.06596557120094992, 9.177570865404522493, -16.67295095431955332 ) ) ;
#7636=CARTESIAN_POINT ( 'NONE',  ( 33.34778169882233811, -10.20066162918134367, -19.85315749909214844 ) ) ;
#7637=CARTESIAN_POINT ( 'NONE',  ( 16.60417661732421735, 9.954854064686266213, -19.72231676211552909 ) ) ;
#7638=CARTESIAN_POINT ( 'NONE',  ( 26.57062215293289498, -11.41726559881178638, -18.09730928560479057 ) ) ;
#7645=CARTESIAN_POINT ( 'NONE',  ( 33.42826320546385688, -10.41623213582910523, -18.33855703361424361 ) ) ;
#7647=CARTESIAN_POINT ( 'NONE',  ( 18.37740474667574730, 3.980509343919368614, -15.11632106699347844 ) ) ;
#7649=CARTESIAN_POINT ( 'NONE',  ( 28.43808809371321189, -7.037065510061861318, -17.41003659457544117 ) ) ;
#7659=CARTESIAN_POINT ( 'NONE',  ( 10.85049725708738855, 16.03634806290433801, -15.90056160573019284 ) ) ;
#7664=CARTESIAN_POINT ( 'NONE',  ( 12.48799528366842360, 8.565546312597838607, -15.13973160209665991 ) ) ;
#7666=CARTESIAN_POINT ( 'NONE',  ( 18.18253756980838531, -1.899343836538245789, -17.94647550410194370 ) ) ;
#7672=CARTESIAN_POINT ( 'NONE',  ( 12.85916040382217318, 9.514151651470600157, -16.12251888295402580 ) ) ;
#7674=CARTESIAN_POINT ( 'NONE',  ( 35.05137900175546406, -18.95079263513605028, -19.16533087415493952 ) ) ;
#7675=CARTESIAN_POINT ( 'NONE',  ( 16.89609864265585060, 4.102175112930991574, -14.31125941877678720 ) ) ;
#7679=CARTESIAN_POINT ( 'NONE',  ( 15.33641899704135980, 5.898237403637139664, -14.35162154369138676 ) ) ;
#7682=CARTESIAN_POINT ( 'NONE',  ( 22.34648740292275093, -2.602002351270185532, -19.46322174391540116 ) ) ;
#7684=CARTESIAN_POINT ( 'NONE',  ( 18.98827506421364575, 7.203492520304279445, -17.17051369180543929 ) ) ;
#7694=CARTESIAN_POINT ( 'NONE',  ( 11.47372892693763902, 9.265404009280679531, -15.86055721330185619 ) ) ;
#7695=CARTESIAN_POINT ( 'NONE',  ( 28.09155340820903390, -11.11649160481613130, -13.74484337247343824 ) ) ;
#7696=CARTESIAN_POINT ( 'NONE',  ( 22.09907825138052218, -7.445301066569870230, -16.29136317631293807 ) ) ;
#7698=CARTESIAN_POINT ( 'NONE',  ( 33.17819505895439391, -11.78846528140086924, -19.49437495119144259 ) ) ;
#7709=CARTESIAN_POINT ( 'NONE',  ( 17.21692058948253035, 4.245457944912791604, -14.13226496128363863 ) ) ;
#7712=CARTESIAN_POINT ( 'NONE',  ( 10.72094366404044408, 16.63049735485946101, -15.95413657539408980 ) ) ;
#7715=CARTESIAN_POINT ( 'NONE',  ( 19.25770813156441008, -2.543370271471735222, -15.40753146551623587 ) ) ;
#7716=CARTESIAN_POINT ( 'NONE',  ( 32.47832896513632761, -9.914179286496517918, -13.92895715894296771 ) ) ;
#7718=CARTESIAN_POINT ( 'NONE',  ( 35.53434814243864537, -22.12051714835155281, -18.84852710552948096 ) ) ;
#7719=CARTESIAN_POINT ( 'NONE',  ( 26.06151603483908019, -7.281686956891486595, -19.93845510724469960 ) ) ;
#7720=CARTESIAN_POINT ( 'NONE',  ( 18.73405575602592776, 1.888441813480535414, -14.99786396448725156 ) ) ;
#7731=CARTESIAN_POINT ( 'NONE',  ( 36.54859390953724585, -22.18451583373416014, -17.99055332684694974 ) ) ;
#7732=CARTESIAN_POINT ( 'NONE',  ( 9.981537699549546616, 16.10875070413535681, -16.47763325427154868 ) ) ;
#7738=CARTESIAN_POINT ( 'NONE',  ( 12.02609123740286101, 9.325023229212996867, -16.69214155778140096 ) ) ;
#7750=CARTESIAN_POINT ( 'NONE',  ( 11.32192133241855103, 8.753083428987814330, -17.19257025691282337 ) ) ;
#7752=CARTESIAN_POINT ( 'NONE',  ( 23.84753192840887337, -5.516882280943989691, -18.03677479665242345 ) ) ;
#7753=CARTESIAN_POINT ( 'NONE',  ( 23.74924978780510898, -3.048960050427876656, -13.27477993493952191 ) ) ;
#7764=CARTESIAN_POINT ( 'NONE',  ( 12.02001262747988797, 9.352900509162292764, -16.69465527681230199 ) ) ;
#7765=CARTESIAN_POINT ( 'NONE',  ( 33.80310782676656345, -13.34297147354166135, -18.78800844379110302 ) ) ;
#7767=CARTESIAN_POINT ( 'NONE',  ( 8.944584683310379702, 16.95159276115599667, -17.97192418671890835 ) ) ;
#7770=CARTESIAN_POINT ( 'NONE',  ( 22.86252235622482587, -0.9498377794471745128, -13.29674124224850118 ) ) ;
#7772=CARTESIAN_POINT ( 'NONE',  ( 12.67014222779069854, 10.28407994610609144, -16.20807751338157843 ) ) ;
#7776=CARTESIAN_POINT ( 'NONE',  ( 9.957223259857686415, 16.22025982393231303, -16.48768813039480818 ) ) ;
#7778=CARTESIAN_POINT ( 'NONE',  ( 9.910898653440767703, 16.43271037397421708, -16.50709950392603531 ) ) ;
#7784=CARTESIAN_POINT ( 'NONE',  ( 11.98759337455738816, 9.501579335558542283, -16.70806177831036976 ) ) ;
#7787=CARTESIAN_POINT ( 'NONE',  ( 36.54859390954302967, -23.18451583373416014, -15.55638201429745848 ) ) ;
#7788=CARTESIAN_POINT ( 'NONE',  ( 29.82081855766934453, -7.722587238354316597, -15.76009366473342332 ) ) ;
#7789=CARTESIAN_POINT ( 'NONE',  ( 17.30683543869610119, 10.98570342618945617, -17.92154440881979482 ) ) ;
#7798=CARTESIAN_POINT ( 'NONE',  ( 19.81827328964134338, 3.502454073897792952, -18.79004964864563476 ) ) ;
#7799=CARTESIAN_POINT ( 'NONE',  ( 17.85084670134855145, 5.929878015568476712, -20.08862479909851828 ) ) ;
#7810=CARTESIAN_POINT ( 'NONE',  ( 12.26606010314042017, 9.512972848517913249, -15.31757320754432605 ) ) ;
#7815=CARTESIAN_POINT ( 'NONE',  ( 12.51757296969303290, 8.578467993704791184, -15.11616904564172792 ) ) ;
#7816=CARTESIAN_POINT ( 'NONE',  ( 19.38139026969670553, 5.460277215109251792, -15.14974238112136540 ) ) ;
#7823=CARTESIAN_POINT ( 'NONE',  ( 12.67014222779069854, 10.28407994610609144, -16.20807751338157843 ) ) ;
#7826=CARTESIAN_POINT ( 'NONE',  ( 36.44623027834506956, -20.72465026231317253, -19.27049969669971929 ) ) ;
#7827=CARTESIAN_POINT ( 'NONE',  ( 21.66440995182641416, 5.535554982823286174, -17.57621636221614025 ) ) ;
#7830=CARTESIAN_POINT ( 'NONE',  ( 26.89114594638229505, -13.18314149429672000, -12.91981678032827041 ) ) ;
#7833=CARTESIAN_POINT ( 'NONE',  ( 26.78588127033857091, -2.187643107580064861, -16.18476928258297676 ) ) ;
#7834=CARTESIAN_POINT ( 'NONE',  ( 20.65939765650831461, 5.541921473274042498, -17.57530766875797568 ) ) ;
#7845=CARTESIAN_POINT ( 'NONE',  ( 11.58682163191119230, 8.958038730125363003, -15.79767441425272345 ) ) ;
#7846=CARTESIAN_POINT ( 'NONE',  ( 29.29611939376944107, -10.57052713796966081, -13.72407686852593400 ) ) ;
#7847=CARTESIAN_POINT ( 'NONE',  ( 28.50411217586706769, -6.135108760518566129, -18.55796808427148648 ) ) ;
#7848=CARTESIAN_POINT ( 'NONE',  ( 35.54859390954303677, -23.18451583373416014, -15.55638201429745848 ) ) ;
#7856=CARTESIAN_POINT ( 'NONE',  ( 16.89609864265585060, 4.102175112930991574, -14.31125941877678720 ) ) ;
#7859=CARTESIAN_POINT ( 'NONE',  ( 12.14726737398757095, 10.08919500705755645, -15.36430154580878593 ) ) ;
#7862=CARTESIAN_POINT ( 'NONE',  ( 24.92864811393110358, -0.2441600445015326137, -14.78813717129899885 ) ) ;
#7863=CARTESIAN_POINT ( 'NONE',  ( 20.91577097522866424, 8.170114823437694795, -18.25116917207579093 ) ) ;
#7865=CARTESIAN_POINT ( 'NONE',  ( 33.96943610671532809, -15.09019632882451134, -19.88060704079178720 ) ) ;
#7867=CARTESIAN_POINT ( 'NONE',  ( 28.50845745928996067, -4.315366227951761502, -16.60164569054668604 ) ) ;
#7869=CARTESIAN_POINT ( 'NONE',  ( 21.02038916656773182, -4.531596735700774481, -13.49074533895851147 ) ) ;
#7873=CARTESIAN_POINT ( 'NONE',  ( 21.54098841764929873, -5.100688324319140321, -15.19385678519978633 ) ) ;
#7884=CARTESIAN_POINT ( 'NONE',  ( 34.33515578781254618, -12.24072284059296933, -19.92088757525016973 ) ) ;
#7885=CARTESIAN_POINT ( 'NONE',  ( 9.776119957569173735, 17.05082265352876547, -16.72288386497739765 ) ) ;
#7888=CARTESIAN_POINT ( 'NONE',  ( 12.02001262747988797, 9.352900509162292764, -16.69465527681230199 ) ) ;
#7899=CARTESIAN_POINT ( 'NONE',  ( 11.22408442728515077, 9.090372555205103566, -17.24152585048573982 ) ) ;
#7900=CARTESIAN_POINT ( 'NONE',  ( 13.78422571733443647, 6.778978001458615843, -20.29761332830707232 ) ) ;
#7901=CARTESIAN_POINT ( 'NONE',  ( 21.56383972367567736, -3.323709001909281202, -18.92284382192250192 ) ) ;
#7914=CARTESIAN_POINT ( 'NONE',  ( 13.12553198385420927, 8.571700941790735939, -15.91037888968202552 ) ) ;
#7915=CARTESIAN_POINT ( 'NONE',  ( 35.52583876341286384, -22.08228901593173177, -18.97221062538168113 ) ) ;
#7917=CARTESIAN_POINT ( 'NONE',  ( 9.068088202150136112, 16.38518988071972871, -17.09785080524718381 ) ) ;
#7919=CARTESIAN_POINT ( 'NONE',  ( 24.43075134246613800, -6.859861339260811874, -14.00379227226492951 ) ) ;
#7920=CARTESIAN_POINT ( 'NONE',  ( 12.83230269852989203, 9.540395929213350001, -16.14101810565610151 ) ) ;
#7924=CARTESIAN_POINT ( 'NONE',  ( 11.47511325496290624, 9.259230714725578792, -15.85997136665693041 ) ) ;
#7929=CARTESIAN_POINT ( 'NONE',  ( 12.02841764901576838, 9.314357472305010432, -16.69117924060192948 ) ) ;
#7931=CARTESIAN_POINT ( 'NONE',  ( 22.08592964957147586, 4.518037853963432049, -19.67680751601638889 ) ) ;
#7932=CARTESIAN_POINT ( 'NONE',  ( 13.34169928452473819, 6.621333031661079005, -16.53230918748570488 ) ) ;
#7936=CARTESIAN_POINT ( 'NONE',  ( 36.54222296954648641, -22.15589457513855010, -18.69601260479128513 ) ) ;
#7938=CARTESIAN_POINT ( 'NONE',  ( 20.59924605810746101, 4.422246688411098248, -17.72709849028201035 ) ) ;
#7939=CARTESIAN_POINT ( 'NONE',  ( 16.75072914628186282, 8.771658487634226731, -19.67538163746542779 ) ) ;
#7952=CARTESIAN_POINT ( 'NONE',  ( 12.27691367651725862, 9.494620545951883983, -15.31068823849801319 ) ) ;
#7956=CARTESIAN_POINT ( 'NONE',  ( 12.60945047077962933, 8.619070305187777947, -15.04294105552940231 ) ) ;
#7959=CARTESIAN_POINT ( 'NONE',  ( 10.66878845912243534, 9.044174962973633214, -16.41115715542894193 ) ) ;
#7966=CARTESIAN_POINT ( 'NONE',  ( 12.83097211533594439, 9.546493580781078236, -16.14156869735677446 ) ) ;
#7968=CARTESIAN_POINT ( 'NONE',  ( 34.47095863366522650, -11.93304594944324926, -18.87179757263150037 ) ) ;
#7969=CARTESIAN_POINT ( 'NONE',  ( 16.21960234321935701, 7.070186740785398882, -14.59618053200276044 ) ) ;
#7973=CARTESIAN_POINT ( 'NONE',  ( 25.64694198568010819, -13.68525919019184300, -15.02544717525507778 ) ) ;
#7977=CARTESIAN_POINT ( 'NONE',  ( 23.93603600111211804, 0.1510904554606163908, -14.93755387302875448 ) ) ;
#7978=CARTESIAN_POINT ( 'NONE',  ( 20.46796597391333350, 5.758383238370681667, -16.38968713894368534 ) ) ;
#7989=CARTESIAN_POINT ( 'NONE',  ( 11.97192087863669663, 8.579774655713777065, -15.53257280409644991 ) ) ;
#7990=CARTESIAN_POINT ( 'NONE',  ( 28.00362220295478721, -7.540254448315821811, -17.98007619878529439 ) ) ;
#7991=CARTESIAN_POINT ( 'NONE',  ( 26.68443370873975340, -2.140902173977853540, -15.79004130932784555 ) ) ;
#7999=CARTESIAN_POINT ( 'NONE',  ( 19.02541433733466647, 1.263421280649871248, -13.57496312174407826 ) ) ;
#8003=CARTESIAN_POINT ( 'NONE',  ( 12.27643783485070372, 9.496802808135052842, -15.31088501640310540 ) ) ;
#8007=CARTESIAN_POINT ( 'NONE',  ( 19.68115760211910725, 3.144890361740488860, -20.29587546762095940 ) ) ;
#8010=CARTESIAN_POINT ( 'NONE',  ( 21.96101381878726500, 3.467707295883769802, -19.37612211972275844 ) ) ;
#8013=CARTESIAN_POINT ( 'NONE',  ( 23.66316133457650750, -10.02594615916883392, -14.11990577516520595 ) ) ;
#8014=CARTESIAN_POINT ( 'NONE',  ( 24.92117679868390923, -7.366661744264540346, -12.55155079749028779 ) ) ;
#8017=CARTESIAN_POINT ( 'NONE',  ( 24.68825858685077179, -9.385095155728059524, -16.92495907518576104 ) ) ;
#8025=CARTESIAN_POINT ( 'NONE',  ( 33.33685173283005554, -10.38074443705513161, -18.09276096107157628 ) ) ;
#8026=CARTESIAN_POINT ( 'NONE',  ( 10.56508425215480074, 13.43253182900300402, -16.23631622730588830 ) ) ;
#8029=CARTESIAN_POINT ( 'NONE',  ( 9.661885998671275289, 16.25481316389105402, -17.91482063482849441 ) ) ;
#8040=ORIENTED_EDGE ( 'NONE', *, *, #1414, .T. ) ;
#8042=CARTESIAN_POINT ( 'NONE',  ( 13.35290877858212255, 7.614465999429414822, -15.72913170295453966 ) ) ;
#8043=CARTESIAN_POINT ( 'NONE',  ( 13.23210690081759111, 9.952263081781872245, -14.54667289943505004 ) ) ;
#8044=CARTESIAN_POINT ( 'NONE',  ( 26.06583011202948441, -9.749651170145462231, -12.94692625511877182 ) ) ;
#8055=CARTESIAN_POINT ( 'NONE',  ( 12.98644063677341798, 8.526496012441747041, -16.01999686492960961 ) ) ;
#8057=CARTESIAN_POINT ( 'NONE',  ( 35.54859390953724585, -22.18451583373416014, -17.99055332684694974 ) ) ;
#8060=CARTESIAN_POINT ( 'NONE',  ( 9.112135424753279977, 16.18318370314694832, -17.05489040841110437 ) ) ;
#8062=CARTESIAN_POINT ( 'NONE',  ( 26.61709978538234012, -3.831456866606135492, -17.85214630790261836 ) ) ;
#8063=CARTESIAN_POINT ( 'NONE',  ( 12.83225436833568089, 9.540613290865683993, -16.14103841883858337 ) ) ;
#8069=CARTESIAN_POINT ( 'NONE',  ( 12.49664108868010182, 8.569232744350554043, -15.13285098609708790 ) ) ;
#8075=CARTESIAN_POINT ( 'NONE',  ( 12.03623766312057519, 9.280706639558555793, -16.68777662621714342 ) ) ;
#8078=CARTESIAN_POINT ( 'NONE',  ( 15.44177808481316383, 7.494736869644298416, -14.00399691429678306 ) ) ;
#8079=CARTESIAN_POINT ( 'NONE',  ( 18.26079443319284934, -0.1287745640203900310, -14.06839115638798354 ) ) ;
#8082=CARTESIAN_POINT ( 'NONE',  ( 36.02474454408307736, -19.83113812547715682, -20.43161669954002591 ) ) ;
#8084=CARTESIAN_POINT ( 'NONE',  ( 20.92249676953290916, 2.861121271339598593, -14.71414025844469720 ) ) ;
#8086=CARTESIAN_POINT ( 'NONE',  ( 19.52227536296714305, 7.868296793410291201, -18.00468392081665669 ) ) ;
#8096=CARTESIAN_POINT ( 'NONE',  ( 11.75823633891744535, 11.87334092381181883, -15.52517956378672359 ) ) ;
#8102=CARTESIAN_POINT ( 'NONE',  ( 11.47652547240386944, 9.253065934422213701, -15.85936358228339316 ) ) ;
#8106=CARTESIAN_POINT ( 'NONE',  ( 10.66857885413002727, 9.045135741668604012, -16.41124387233542592 ) ) ;
#8115=CARTESIAN_POINT ( 'NONE',  ( 12.82210747586494293, 9.587147947373788170, -16.14523453761016825 ) ) ;
#8117=CARTESIAN_POINT ( 'NONE',  ( 36.14373538984320078, -19.36570096427324827, -19.42526322947885475 ) ) ;
#8118=CARTESIAN_POINT ( 'NONE',  ( 19.68115760211910725, 3.144890361740488860, -20.29587546762095940 ) ) ;
#8122=CARTESIAN_POINT ( 'NONE',  ( 26.55441479597953247, -12.51626325376082249, -18.99724541349076645 ) ) ;
#8126=CARTESIAN_POINT ( 'NONE',  ( 20.31878617967674217, -0.6648838724932636390, -18.90140657046049455 ) ) ;
#8127=CARTESIAN_POINT ( 'NONE',  ( 22.27366892561238387, -0.4200048385588530664, -12.54648181008633934 ) ) ;
#8138=CARTESIAN_POINT ( 'NONE',  ( 10.24089172292967298, 14.91932009296530559, -16.37038124228770997 ) ) ;
#8139=CARTESIAN_POINT ( 'NONE',  ( 15.46244301724551740, 3.702889819443702990, -17.82701508041758842 ) ) ;
#8140=CARTESIAN_POINT ( 'NONE',  ( 26.68716238812262631, -2.792712658874448639, -18.04699283665395981 ) ) ;
#8150=CARTESIAN_POINT ( 'NONE',  ( 22.89472691350227507, 1.279074496056108901, -19.72372301458170796 ) ) ;
#8154=CARTESIAN_POINT ( 'NONE',  ( 12.27549906412561675, 9.499463866199420181, -15.31139863700699344 ) ) ;
#8158=CARTESIAN_POINT ( 'NONE',  ( 21.40051611374530793, -0.1690565882708310874, -20.18282279970310000 ) ) ;
#8160=CARTESIAN_POINT ( 'NONE',  ( 19.48958755759471728, 3.937961857331544469, -13.19130291127160959 ) ) ;
#8163=CARTESIAN_POINT ( 'NONE',  ( 25.29949251596307036, -5.094144391296384633, -13.01082609127739076 ) ) ;
#8164=CARTESIAN_POINT ( 'NONE',  ( 22.29950228926167100, 0.3472756386405770335, -13.33132414558515677 ) ) ;
#8165=CARTESIAN_POINT ( 'NONE',  ( 26.92971693216691165, -8.617903733377630715, -13.36642543767191427 ) ) ;
#8175=CARTESIAN_POINT ( 'NONE',  ( 36.21530066971708095, -20.68720585756345187, -20.37220581101806971 ) ) ;
#8176=CARTESIAN_POINT ( 'NONE',  ( 9.924804006935172396, 16.36893865032855899, -16.50109463189289016 ) ) ;
#8179=CARTESIAN_POINT ( 'NONE',  ( 13.12425544150138279, 8.571136816377206813, -15.91139631635614471 ) ) ;
#8192=CARTESIAN_POINT ( 'NONE',  ( 13.51537010444165254, 7.685947621549766851, -15.59967102646339043 ) ) ;
#8194=CARTESIAN_POINT ( 'NONE',  ( 12.96291568738609890, 5.695260009123724210, -16.43886026595064109 ) ) ;
#8195=CARTESIAN_POINT ( 'NONE',  ( 28.73289915209718615, -4.972737245092835323, -15.12275039236161689 ) ) ;
#8206=CARTESIAN_POINT ( 'NONE',  ( 13.11714404544056656, 8.568033937426095648, -15.91706119101506545 ) ) ;
#8208=CARTESIAN_POINT ( 'NONE',  ( 33.71394559998177698, -12.94241281914233355, -18.76105684162217457 ) ) ;
#8211=CARTESIAN_POINT ( 'NONE',  ( 10.34450975306715570, 10.53135794231081057, -16.54525784588868120 ) ) ;
#8213=CARTESIAN_POINT ( 'NONE',  ( 22.90372073960079646, -4.505259139820817715, -13.75793632099288111 ) ) ;
#8214=CARTESIAN_POINT ( 'NONE',  ( 12.86826794643883609, 9.516041646402381815, -16.11542282846662388 ) ) ;
#8221=CARTESIAN_POINT ( 'NONE',  ( 12.49977518293622758, 8.570603418560722275, -15.13035415120363325 ) ) ;
#8226=CARTESIAN_POINT ( 'NONE',  ( 13.06976498004312326, 8.549601185932660385, -15.95463209657921055 ) ) ;
#8228=CARTESIAN_POINT ( 'NONE',  ( 13.97862894411929879, 7.467096638697104716, -19.56757695884047621 ) ) ;
#8229=CARTESIAN_POINT ( 'NONE',  ( 14.77169846916584461, 3.272981165966227568, -18.54959716842853723 ) ) ;
#8232=CARTESIAN_POINT ( 'NONE',  ( 36.44920892064849482, -21.73803172434679354, -19.68085951391205057 ) ) ;
#8234=CARTESIAN_POINT ( 'NONE',  ( 17.95327243003904982, 7.812726124483462264, -14.88485059575767266 ) ) ;
#8245=CARTESIAN_POINT ( 'NONE',  ( 32.12153525177792091, -10.97127362787143312, -16.88978156643115724 ) ) ;
#8249=CARTESIAN_POINT ( 'NONE',  ( 11.05541542350396256, 17.68942290035798237, -17.91468072056456862 ) ) ;
#8255=CARTESIAN_POINT ( 'NONE',  ( 12.62682997171803123, 7.576475742438638861, -15.02849783152220908 ) ) ;
#8262=CARTESIAN_POINT ( 'NONE',  ( 12.83227036137552446, 9.540540802112166929, -16.14103173976383587 ) ) ;
#8263=CARTESIAN_POINT ( 'NONE',  ( 33.90312036197754963, -11.11655558909185615, -17.69153855583423862 ) ) ;
#8264=CARTESIAN_POINT ( 'NONE',  ( 22.90372073960079646, -4.505259139820817715, -13.75793632099288111 ) ) ;
#8268=CARTESIAN_POINT ( 'NONE',  ( 15.17188473929424930, 6.803351907998973935, -20.50413427079521256 ) ) ;
#8272=CARTESIAN_POINT ( 'NONE',  ( 19.60850488237918654, -1.635242255716521820, -15.65509664672261003 ) ) ;
#8273=CARTESIAN_POINT ( 'NONE',  ( 23.16986854814090080, 3.028408164773654931, -18.83379972368585342 ) ) ;
#8288=CARTESIAN_POINT ( 'NONE',  ( 11.21994398240249957, 9.109360644301018439, -17.24323810967081982 ) ) ;
#8289=CARTESIAN_POINT ( 'NONE',  ( 11.47310491742633687, 9.268236560789974376, -15.86081749295074594 ) ) ;
#8290=CARTESIAN_POINT ( 'NONE',  ( 30.07542022419311678, -8.155067017681195907, -14.09159111155252120 ) ) ;
#8300=CARTESIAN_POINT ( 'NONE',  ( 18.34549112274340033, 0.9605221043122941227, -13.99314825615798341 ) ) ;
#8303=CARTESIAN_POINT ( 'NONE',  ( 10.85049725708738855, 16.03634806290433801, -15.90056160573019284 ) ) ;
#8308=CARTESIAN_POINT ( 'NONE',  ( 20.52488529563827058, 3.974637744936419637, -19.97762432673833288 ) ) ;
#8310=CARTESIAN_POINT ( 'NONE',  ( 15.95545008109832530, 6.956385541780823800, -13.20154910664163950 ) ) ;
#8314=CARTESIAN_POINT ( 'NONE',  ( 27.35338705259445646, -4.307586880325415812, -13.99634582963401996 ) ) ;
#8315=CARTESIAN_POINT ( 'NONE',  ( 27.86916612644401425, -2.348388412649441648, -16.97020329177912501 ) ) ;
#8331=CARTESIAN_POINT ( 'NONE',  ( 25.86774690167791135, -3.337865513817628749, -16.68124922160397006 ) ) ;
#8332=CARTESIAN_POINT ( 'NONE',  ( 15.10175627602374249, 9.741420229655037843, -13.89989488922661742 ) ) ;
#8333=CARTESIAN_POINT ( 'NONE',  ( 33.94449656094377588, -11.59990251341361933, -20.77871222707083376 ) ) ;
#8335=CARTESIAN_POINT ( 'NONE',  ( 9.921764701973689426, 16.38287729030320250, -16.50235149140834778 ) ) ;
#8338=CARTESIAN_POINT ( 'NONE',  ( 13.12553198385420927, 8.571700941790735939, -15.91037888968202552 ) ) ;
#8341=CARTESIAN_POINT ( 'NONE',  ( 11.47304865262203499, 9.268493388164605662, -15.86084085272616484 ) ) ;
#8348=CARTESIAN_POINT ( 'NONE',  ( 17.72817910449685996, 9.547663288818908356, -12.24198789229035533 ) ) ;
#8349=CARTESIAN_POINT ( 'NONE',  ( 31.68531546575670532, -10.25520638109567173, -17.65856934995331784 ) ) ;
#8351=CARTESIAN_POINT ( 'NONE',  ( 30.15790919126650138, -6.784097790808209183, -15.35074926656157324 ) ) ;
#8352=CARTESIAN_POINT ( 'NONE',  ( 23.54468722040186890, -6.934586491718037315, -13.40271233150634878 ) ) ;
#8364=CARTESIAN_POINT ( 'NONE',  ( 12.11773132146483789, 9.045882004348337446, -16.64348121447567053 ) ) ;
#8365=CARTESIAN_POINT ( 'NONE',  ( 35.54859569580823830, -22.18452385850428499, -18.27063337037174762 ) ) ;
#8367=CARTESIAN_POINT ( 'NONE',  ( 8.945901566930443138, 16.94555336501101550, -17.80918358208353069 ) ) ;
#8369=CARTESIAN_POINT ( 'NONE',  ( 26.18758235895636233, -4.355437658720127558, -18.53605802859044260 ) ) ;
#8370=CARTESIAN_POINT ( 'NONE',  ( 12.86833691348896203, 9.516071730297785081, -16.11536789055087837 ) ) ;
#8374=CARTESIAN_POINT ( 'NONE',  ( 11.58682163191119230, 8.958038730125363003, -15.79767441425272345 ) ) ;
#8380=CARTESIAN_POINT ( 'NONE',  ( 13.12216094266758581, 8.570213704404382682, -15.91306547940487448 ) ) ;
#8383=CARTESIAN_POINT ( 'NONE',  ( 16.51977620067554042, 7.986930271725532826, -13.83285890266734519 ) ) ;
#8384=CARTESIAN_POINT ( 'NONE',  ( 17.64024190839899120, 8.465516882244152441, -14.08803959672746586 ) ) ;
#8389=CARTESIAN_POINT ( 'NONE',  ( 20.22088415693689356, -1.238650738454883493, -19.72259765018230482 ) ) ;
#8396=CARTESIAN_POINT ( 'NONE',  ( 34.39741479528305490, -17.01287786994462792, -20.00997473120332515 ) ) ;
#8397=CARTESIAN_POINT ( 'NONE',  ( 13.15390973649967599, 8.859676595473322536, -14.60899741038990562 ) ) ;
#8400=CARTESIAN_POINT ( 'NONE',  ( 12.26214823032917778, 9.523620991859985452, -15.31974707146758341 ) ) ;
#8401=CARTESIAN_POINT ( 'NONE',  ( 34.96958981470057637, -20.58335714263341387, -21.20026138435576613 ) ) ;
#8407=CARTESIAN_POINT ( 'NONE',  ( 10.83941243988239833, 8.530520621650927282, -16.32009337531726345 ) ) ;
#8412=CARTESIAN_POINT ( 'NONE',  ( 12.87010724449035415, 9.516853939945930208, -16.11395691550788101 ) ) ;
#8415=CARTESIAN_POINT ( 'NONE',  ( 36.31991209326969283, -20.15716956937155047, -19.46864736847591359 ) ) ;
#8416=CARTESIAN_POINT ( 'NONE',  ( 19.40121574091639189, 1.432572567346982240, -13.43353846741550406 ) ) ;
#8426=CARTESIAN_POINT ( 'NONE',  ( 28.92999000670439713, -5.550862855971650411, -17.57004703619191943 ) ) ;
#8427=CARTESIAN_POINT ( 'NONE',  ( 18.72855672543857608, 2.184447897796080174, -13.82944682127929426 ) ) ;
#8438=CARTESIAN_POINT ( 'NONE',  ( 11.22446318822032296, 9.088639264749929225, -17.24136893309019669 ) ) ;
#8439=CARTESIAN_POINT ( 'NONE',  ( 10.33811693838771717, 18.38618951776012267, -17.91752729848688830 ) ) ;
#8440=CARTESIAN_POINT ( 'NONE',  ( 30.50670359208957905, -8.903545733563623443, -17.67935522427464079 ) ) ;
#8448=CARTESIAN_POINT ( 'NONE',  ( 26.04489551603160180, -6.130266781319400948, -13.71289979607875154 ) ) ;
#8450=CARTESIAN_POINT ( 'NONE',  ( 12.27129069473257239, 9.507470051170034964, -15.31400031939534045 ) ) ;
#8453=CARTESIAN_POINT ( 'NONE',  ( 32.77977724007769211, -11.13765286058784554, -18.71157503069099448 ) ) ;
#8457=CARTESIAN_POINT ( 'NONE',  ( 26.58455406938135468, -5.910422570377376950, -13.89432871846328688 ) ) ;
#8460=CARTESIAN_POINT ( 'NONE',  ( 18.26618351132839280, 3.382507019981081164, -13.19753224271465797 ) ) ;
#8465=( LENGTH_UNIT ( ) NAMED_UNIT ( * ) SI_UNIT ( .MILLI., .METRE. ) );
#8466=CARTESIAN_POINT ( 'NONE',  ( 28.90796184913828171, -12.27476343136570414, -11.88515153054143347 ) ) ;
#8467=CARTESIAN_POINT ( 'NONE',  ( 23.45579420008465732, -3.438291973250592992, -12.29892528769388349 ) ) ;
#8477=CARTESIAN_POINT ( 'NONE',  ( 25.47886751038978304, -3.221426504603704277, -15.37741025701318698 ) ) ;
#8479=CARTESIAN_POINT ( 'NONE',  ( 35.65609946332594404, -19.17501105436304343, -21.36250568352834378 ) ) ;
#8481=CARTESIAN_POINT ( 'NONE',  ( 12.49271550807400999, 8.567542729147559655, -15.13597632865050535 ) ) ;
#8485=CARTESIAN_POINT ( 'NONE',  ( 9.661894807476521407, 16.25477276558749296, -17.91386948909976695 ) ) ;
#8488=CARTESIAN_POINT ( 'NONE',  ( 10.56508425215480074, 13.43253182900300402, -16.23631622730588830 ) ) ;
#8498=CARTESIAN_POINT ( 'NONE',  ( 13.39626964006587428, 7.633314995549595139, -15.69459619883729928 ) ) ;
#8499=CARTESIAN_POINT ( 'NONE',  ( 32.00851579392290347, -10.30430276118739918, -18.57203464379605151 ) ) ;
#8500=CARTESIAN_POINT ( 'NONE',  ( 18.20609423209794642, 11.47008825724650549, -18.02705416172272734 ) ) ;
#8501=CARTESIAN_POINT ( 'NONE',  ( 24.40455984355908114, -10.10244183743681035, -17.68366952546245585 ) ) ;
#8513=CARTESIAN_POINT ( 'NONE',  ( 13.34161425493533315, 8.667191563245470576, -15.73815750552000381 ) ) ;
#8515=CARTESIAN_POINT ( 'NONE',  ( 35.54824714876834690, -21.18295802128256611, -18.40066978570660083 ) ) ;
#8517=CARTESIAN_POINT ( 'NONE',  ( 9.112400085652602399, 16.18196993452624355, -17.05477891849903926 ) ) ;
#8519=CARTESIAN_POINT ( 'NONE',  ( 28.12266609392075267, -5.599633216697744942, -16.00068813756295327 ) ) ;
#8520=CARTESIAN_POINT ( 'NONE',  ( 10.35864918915110877, 16.97212501191939538, -17.95086732675817132 ) ) ;
#8531=CARTESIAN_POINT ( 'NONE',  ( 9.661883355341293722, 16.25482528653935077, -17.91547504436015004 ) ) ;
#8532=CARTESIAN_POINT ( 'NONE',  ( 18.76724195421386554, 7.045283186750163296, -20.62625128596355495 ) ) ;
#8533=CARTESIAN_POINT ( 'NONE',  ( 15.09088459799990822, 3.595497735170159803, -19.35696164441904443 ) ) ;
#8537=CARTESIAN_POINT ( 'NONE',  ( 16.89369580670022941, 0.5033910033923695293, -17.32063897790030893 ) ) ;
#8544=CARTESIAN_POINT ( 'NONE',  ( 35.09336438560361415, -20.13941072448723801, -20.22035334018532637 ) ) ;
#8548=CARTESIAN_POINT ( 'NONE',  ( 11.05541531668977662, 17.68942339022145305, -17.92015940598198753 ) ) ;
#8549=CARTESIAN_POINT ( 'NONE',  ( 35.54859390953723164, -23.18451583373416014, -14.99999999999999822 ) ) ;
#8552=CARTESIAN_POINT ( 'NONE',  ( 12.71834232392635045, 8.667191563245470576, -14.95615232649864090 ) ) ;
#8554=CARTESIAN_POINT ( 'NONE',  ( 10.66915452275446619, 9.042499785519874322, -16.41100549784887619 ) ) ;
#8560=CARTESIAN_POINT ( 'NONE',  ( 12.86729516143382845, 9.515644835462770956, -16.11619563230584973 ) ) ;
#8563=CARTESIAN_POINT ( 'NONE',  ( 36.54859390953724585, -21.18451583373416014, -17.22552805718784441 ) ) ;
#8564=CARTESIAN_POINT ( 'NONE',  ( 17.55424633453837302, 0.6138019359854992585, -14.89346452969079060 ) ) ;
#8570=CARTESIAN_POINT ( 'NONE',  ( 27.71186802668094273, -7.007055141436442369, -19.33373627201896383 ) ) ;
#8571=CARTESIAN_POINT ( 'NONE',  ( 20.32939975687981615, -5.674178230592766603, -17.16996371750385109 ) ) ;
#8585=CARTESIAN_POINT ( 'NONE',  ( 11.22390034614927856, 9.091215689738174177, -17.24160205726399653 ) ) ;
#8586=CARTESIAN_POINT ( 'NONE',  ( 12.56861602585598980, 8.601024833420110483, -15.07548682890769243 ) ) ;
#8591=CARTESIAN_POINT ( 'NONE',  ( 9.641354186875979337, 17.66887565656821124, -17.90893343548146177 ) ) ;
#8595=CARTESIAN_POINT ( 'NONE',  ( 22.90372073960079646, -4.505259139820817715, -13.75793632099288111 ) ) ;
#8599=CARTESIAN_POINT ( 'NONE',  ( 12.24726067228269422, 9.517041913610183812, -15.33161271801373182 ) ) ;
#8603=CARTESIAN_POINT ( 'NONE',  ( 23.60870351872479844, -7.222488552757559077, -14.83554404960226947 ) ) ;
#8605=CARTESIAN_POINT ( 'NONE',  ( 23.81787570424677014, -0.6874775570582684070, -15.56398403670522157 ) ) ;
#8607=CARTESIAN_POINT ( 'NONE',  ( 35.54859390953723874, -22.18451583373416014, -15.00000000000000000 ) ) ;
#8609=CARTESIAN_POINT ( 'NONE',  ( 13.78676817088038931, 5.425489125369224119, -17.89072192914586168 ) ) ;
#8611=CARTESIAN_POINT ( 'NONE',  ( 27.20859382114707614, -12.49599901988731077, -15.99530080614381511 ) ) ;
#8614=CARTESIAN_POINT ( 'NONE',  ( 29.46565128511723586, -7.689737916804423534, -14.82739468409561567 ) ) ;
#8625=CARTESIAN_POINT ( 'NONE',  ( 23.69966960967911973, -9.104540460734687812, -16.16703237251472558 ) ) ;
#8626=CARTESIAN_POINT ( 'NONE',  ( 21.26575470983302196, 3.903880982571942493, -18.68858533207590966 ) ) ;
#8627=CARTESIAN_POINT ( 'NONE',  ( 35.85321554361588170, -20.06054918781481788, -21.42207597224664894 ) ) ;
#8630=CARTESIAN_POINT ( 'NONE',  ( 11.47511325496290624, 9.259230714725578792, -15.85997136665693041 ) ) ;
#8633=CARTESIAN_POINT ( 'NONE',  ( 13.12808413666193275, 8.572828783776230921, -15.90834477884588516 ) ) ;
#8636=CARTESIAN_POINT ( 'NONE',  ( 12.39803340617553928, 8.535179507765855433, -15.21071672276548625 ) ) ;
#8642=CARTESIAN_POINT ( 'NONE',  ( 8.944584683310379702, 16.95159276115599667, -17.95086732675816776 ) ) ;
#8643=CARTESIAN_POINT ( 'NONE',  ( 31.91112766891453845, -10.28950255622343946, -18.29678896503644481 ) ) ;
#8644=CARTESIAN_POINT ( 'NONE',  ( 22.45977841265724351, 4.097634946112983734, -18.47195213137534964 ) ) ;
#8645=CARTESIAN_POINT ( 'NONE',  ( 30.58006126958193249, -8.114715823802763239, -15.12008790671442426 ) ) ;
#8649=CARTESIAN_POINT ( 'NONE',  ( 26.83635784119175938, -3.902057423304301942, -19.75319010936098962 ) ) ;
#8662=CARTESIAN_POINT ( 'NONE',  ( 35.46586886002400263, -20.81287600694606610, -19.09165458252410374 ) ) ;
#8664=CARTESIAN_POINT ( 'NONE',  ( 12.75280283744833376, 7.624395256242640251, -14.92868632776139037 ) ) ;
#8667=CARTESIAN_POINT ( 'NONE',  ( 26.57062215293289498, -11.41726559881178638, -18.09730928560479057 ) ) ;
#8669=CARTESIAN_POINT ( 'NONE',  ( 14.75361449413180637, 10.34920949090176201, -14.61276839131081218 ) ) ;
#8674=CARTESIAN_POINT ( 'NONE',  ( 15.61762486822808604, 9.948436389806387226, -12.64537296286936829 ) ) ;
#8678=CARTESIAN_POINT ( 'NONE',  ( 9.661884236495001943, 16.25482124545614937, -17.91517755594902894 ) ) ;
#8680=CARTESIAN_POINT ( 'NONE',  ( 22.01749846045582970, -4.595750957016929483, -16.30794181244783303 ) ) ;
#8681=CARTESIAN_POINT ( 'NONE',  ( 20.44279466453895822, 5.363259340322034774, -13.44374883282906552 ) ) ;
#8684=CARTESIAN_POINT ( 'NONE',  ( 20.50636976340433293, -0.9757509181830721356, -19.91080244439677571 ) ) ;
#8695=CARTESIAN_POINT ( 'NONE',  ( 35.02155038278115740, -19.81678845073966500, -20.19863594638463411 ) ) ;
#8699=CARTESIAN_POINT ( 'NONE',  ( 16.79143122783437292, 7.330551994622505063, -14.54187356113185103 ) ) ;
#8700=CARTESIAN_POINT ( 'NONE',  ( 14.13034256312282189, 10.34920949090176201, -13.83076321228938887 ) ) ;
#8704=CARTESIAN_POINT ( 'NONE',  ( 12.79001206111077948, 7.640833942120977440, -14.89903028090515136 ) ) ;
#8710=CARTESIAN_POINT ( 'NONE',  ( 10.35864918915110877, 16.97212501191939538, -17.94384837343789485 ) ) ;
#8712=CARTESIAN_POINT ( 'NONE',  ( 36.54859390954302967, -21.18451583373416014, -15.55638201429745848 ) ) ;
#8713=CARTESIAN_POINT ( 'NONE',  ( 18.04049687913209610, 0.8262538513465327306, -14.27019888128743297 ) ) ;
#8719=CARTESIAN_POINT ( 'NONE',  ( 25.01196530022370368, -10.21768535905550124, -13.66937216179565517 ) ) ;
#8720=CARTESIAN_POINT ( 'NONE',  ( 25.25756851182965335, -6.311239348595019116, -19.54001279501058264 ) ) ;
#8729=CARTESIAN_POINT ( 'NONE',  ( 11.22589550380084411, 9.082134330754477958, -17.24077175062176082 ) ) ;
#8730=CARTESIAN_POINT ( 'NONE',  ( 12.49977518293622758, 8.570603418560722275, -15.13035415120363325 ) ) ;
#8731=CARTESIAN_POINT ( 'NONE',  ( 27.39958189869922123, -12.72506959635235368, -13.65552181841346524 ) ) ;
#8738=CARTESIAN_POINT ( 'NONE',  ( 18.26505246421942275, 9.297698622231314047, -17.43849025199569169 ) ) ;
#8741=CARTESIAN_POINT ( 'NONE',  ( 21.54098841764929873, -5.100688324319140321, -15.19385678519978633 ) ) ;
#8745=CARTESIAN_POINT ( 'NONE',  ( 12.24523703128252983, 9.516147632761573050, -15.33322559543412034 ) ) ;
#8746=CARTESIAN_POINT ( 'NONE',  ( 33.43446274600908907, -12.68684440242773448, -19.71889742777951327 ) ) ;
#8748=CARTESIAN_POINT ( 'NONE',  ( 28.09718568327657806, -5.958257988085632562, -17.17874431236187149 ) ) ;
#8750=CARTESIAN_POINT ( 'NONE',  ( 22.68669718693540105, -3.283095500849226411, -14.44170700164887933 ) ) ;
#8757=CARTESIAN_POINT ( 'NONE',  ( 15.02162844583664736, 5.759011576665847620, -14.59661587647459591 ) ) ;
#8758=CARTESIAN_POINT ( 'NONE',  ( 29.92318863513849436, -9.020257460645494163, -14.67793329163371574 ) ) ;
#8771=CARTESIAN_POINT ( 'NONE',  ( 24.97936687747968776, -7.804033356035183999, -18.74018705570338028 ) ) ;
#8772=CARTESIAN_POINT ( 'NONE',  ( 19.85388831290292799, 7.668379621071204078, -15.62993620635094061 ) ) ;
#8773=CARTESIAN_POINT ( 'NONE',  ( 36.01637063434644404, -20.79351858480864124, -21.36424221831693870 ) ) ;
#8776=CARTESIAN_POINT ( 'NONE',  ( 11.47029057985033340, 9.281140223223081520, -15.86198156829250117 ) ) ;
#8779=CARTESIAN_POINT ( 'NONE',  ( 9.667875940510226584, 16.22734252707768832, -17.88507284477129033 ) ) ;
#8783=CARTESIAN_POINT ( 'NONE',  ( 12.50140887008201851, 8.571324787501421127, -15.12905211845398412 ) ) ;
#8789=CARTESIAN_POINT ( 'NONE',  ( 13.41328399211976397, 7.640833942120977440, -15.68103545992656578 ) ) ;
#8790=CARTESIAN_POINT ( 'NONE',  ( 35.85321554361588170, -20.06054918781481788, -21.42207597224664894 ) ) ;
#8794=CARTESIAN_POINT ( 'NONE',  ( 15.57379856253263206, 2.175854586521385858, -15.33309735461106094 ) ) ;
#8797=CARTESIAN_POINT ( 'NONE',  ( 28.35369828010231785, -12.30166555976806464, -13.00196782638265169 ) ) ;
#8801=CARTESIAN_POINT ( 'NONE',  ( 18.47998620531167902, -1.197692507188573785, -16.87724725366775402 ) ) ;
#8806=SURFACE_STYLE_FILL_AREA ( #13087 ) ;
#8811=CARTESIAN_POINT ( 'NONE',  ( 35.54859390953724585, -21.18451583373416014, -17.78191007148576119 ) ) ;
#8814=CARTESIAN_POINT ( 'NONE',  ( 10.66857885413002727, 9.045135741668604012, -16.41124387233542592 ) ) ;
#8816=CARTESIAN_POINT ( 'NONE',  ( 25.71553203045151292, -8.406338935355361031, -18.42709291467145150 ) ) ;
#8818=CARTESIAN_POINT ( 'NONE',  ( 10.35864918915110877, 16.97212501191939538, -17.91928203681695564 ) ) ;
#8828=CARTESIAN_POINT ( 'NONE',  ( 13.13233772467555660, 8.574708520419219937, -15.90495459411799395 ) ) ;
#8830=CARTESIAN_POINT ( 'NONE',  ( 18.58771872311928774, 0.01515834859250781048, -13.77226461354315035 ) ) ;
#8831=CARTESIAN_POINT ( 'NONE',  ( 22.36047763332208405, -4.488847068091893711, -15.41575731358746104 ) ) ;
#8834=CARTESIAN_POINT ( 'NONE',  ( 21.37428249720081297, 2.009508332918806151, -14.44682725892062614 ) ) ;
#8839=CARTESIAN_POINT ( 'NONE',  ( 20.99533150354982070, 4.487273811465053441, -19.54336078777620500 ) ) ;
#8843=CARTESIAN_POINT ( 'NONE',  ( 10.35864918915110877, 16.97212501191939538, -21.33333333332589277 ) ) ;
#8844=CARTESIAN_POINT ( 'NONE',  ( 35.53434814243864537, -22.12051714835155281, -18.84852710552948096 ) ) ;
#8848=CARTESIAN_POINT ( 'NONE',  ( 18.69974902744413470, 8.051839821468062652, -15.50866580261103955 ) ) ;
#8849=CARTESIAN_POINT ( 'NONE',  ( 12.38124869470495781, 9.576253617860157163, -15.22482189909362660 ) ) ;
#8850=CARTESIAN_POINT ( 'NONE',  ( 35.45944968151609800, -21.78403803824750185, -19.54251958818673174 ) ) ;
#8851=VERTEX_POINT ( 'NONE', #602 ) ;
#8854=CARTESIAN_POINT ( 'NONE',  ( 12.74961974476379289, 7.623002797808662301, -14.93122222525392928 ) ) ;
#8860=CARTESIAN_POINT ( 'NONE',  ( 10.35864918915110877, 16.97212501191939538, -17.91928203681695564 ) ) ;
#8861=CARTESIAN_POINT ( 'NONE',  ( 36.53496835490201988, -21.12330343441383818, -18.71787618725911884 ) ) ;
#8862=CARTESIAN_POINT ( 'NONE',  ( 20.39549844898813191, -2.061726703908969505, -13.85117726305786512 ) ) ;
#8864=PRODUCT ( 'Pedal Return Coil Spring', 'Pedal Return Coil Spring', '', ( #2934 ) ) ;
#8872=CARTESIAN_POINT ( 'NONE',  ( 28.12627659338356878, -5.062120396530918498, -14.05642262879015369 ) ) ;
#8873=CARTESIAN_POINT ( 'NONE',  ( 25.74978097135661770, 0.6894738977563982241, -15.43585696046938160 ) ) ;
#8882=CARTESIAN_POINT ( 'NONE',  ( 12.93612603019711571, 8.763434079353435990, -14.78257486846209545 ) ) ;
#8888=CARTESIAN_POINT ( 'NONE',  ( 14.65865118920550714, 8.193166376910747672, -14.78953851775792216 ) ) ;
#8892=CARTESIAN_POINT ( 'NONE',  ( 25.31619048431776875, -0.2099727537683927225, -15.56338435260822628 ) ) ;
#8896=CARTESIAN_POINT ( 'NONE',  ( 11.05541533128794107, 17.68942332327241829, -17.91551483529627120 ) ) ;
#8897=CARTESIAN_POINT ( 'NONE',  ( 32.91905456285188336, -11.74221475484424104, -17.14214516703887980 ) ) ;
#8899=CARTESIAN_POINT ( 'NONE',  ( 26.72358035960067824, -3.685970424986596772, -17.59444040205794835 ) ) ;
#8901=CARTESIAN_POINT ( 'NONE',  ( 20.68883037063079300, -1.960602941680898548, -15.52464631352181001 ) ) ;
#8905=FILL_AREA_STYLE_COLOUR ( '', #26882 ) ;
#8906=CARTESIAN_POINT ( 'NONE',  ( 32.82164812444874968, -10.95096414870911161, -14.63344683186480211 ) ) ;
#8908=CARTESIAN_POINT ( 'NONE',  ( 30.22932097093386261, -9.048247045011217793, -15.48080783641366942 ) ) ;
#8917=CARTESIAN_POINT ( 'NONE',  ( 25.81628275165185116, -0.2054900511636704452, -18.66752024111776009 ) ) ;
#8918=CARTESIAN_POINT ( 'NONE',  ( 17.94193213664724951, 0.5400182743772068417, -16.55803501089447849 ) ) ;
#8921=CARTESIAN_POINT ( 'NONE',  ( 35.94849409650817762, -20.48858525550898335, -21.40790205994406747 ) ) ;
#8923=CARTESIAN_POINT ( 'NONE',  ( 11.47250673971808688, 9.270976631574885829, -15.86106510822916249 ) ) ;
#8926=CARTESIAN_POINT ( 'NONE',  ( 9.667369220937283458, 16.22966640763102220, -17.88537093449073012 ) ) ;
#8929=CARTESIAN_POINT ( 'NONE',  ( 12.49957999542663600, 8.570517509188613658, -15.13050969259218981 ) ) ;
#8937=VERTEX_POINT ( 'NONE', #14908 ) ;
#8938=CARTESIAN_POINT ( 'NONE',  ( 8.965340528640792783, 16.85640380871598509, -17.50303937619785444 ) ) ;
#8939=CARTESIAN_POINT ( 'NONE',  ( 33.15841575409167064, -12.44672528413413026, -20.67776857359057274 ) ) ;
#8940=CARTESIAN_POINT ( 'NONE',  ( 20.63001478507949926, 2.108136148055946180, -20.13827832349858937 ) ) ;
#8941=CARTESIAN_POINT ( 'NONE',  ( 14.69068284915647560, 4.968298739062387170, -17.53091140782979807 ) ) ;
#8943=CARTESIAN_POINT ( 'NONE',  ( 27.64697528205969590, -2.889103667904926898, -18.32829528246118755 ) ) ;
#8954=CARTESIAN_POINT ( 'NONE',  ( 35.54859390953724585, -21.18451583373416014, -17.64281456791166391 ) ) ;
#8955=CARTESIAN_POINT ( 'NONE',  ( 10.66806909375856627, 9.047473561677174203, -16.41145467664113156 ) ) ;
#8957=CARTESIAN_POINT ( 'NONE',  ( 29.22485947447185595, -8.910266539455653501, -18.36689805200119707 ) ) ;
#8959=CARTESIAN_POINT ( 'NONE',  ( 10.37265302513970688, 16.90790163500151166, -17.63730412279738147 ) ) ;
#8965=CARTESIAN_POINT ( 'NONE',  ( 12.63667343406881294, 8.631100619704961119, -15.02124387326777111 ) ) ;
#8970=CARTESIAN_POINT ( 'NONE',  ( 9.661883061612440926, 16.25482663361732705, -17.95086732675816776 ) ) ;
#8972=CARTESIAN_POINT ( 'NONE',  ( 23.89160689111651337, -1.335809292830872241, -14.36923488517323477 ) ) ;
#8973=CARTESIAN_POINT ( 'NONE',  ( 20.42254326673722531, -2.835881520377886655, -15.10989100197473789 ) ) ;
#8974=CARTESIAN_POINT ( 'NONE',  ( 22.83681518364245022, 2.349634567491368564, -16.30468554850739338 ) ) ;
#8978=CARTESIAN_POINT ( 'NONE',  ( 23.61827771231835982, -0.6465389018800060672, -13.57143891608981612 ) ) ;
#8982=CARTESIAN_POINT ( 'NONE',  ( 10.40163623209820365, 16.77498095339038287, -17.46874319472340176 ) ) ;
#8984=CARTESIAN_POINT ( 'NONE',  ( 35.52583876341286384, -22.08228901593173177, -18.97221062538168113 ) ) ;
#8992=CARTESIAN_POINT ( 'NONE',  ( 16.57956996521092918, 4.788269978297743812, -19.71382457362092566 ) ) ;
#8993=CARTESIAN_POINT ( 'NONE',  ( 11.28117986039200815, 16.65403841451731637, -16.78246231193739035 ) ) ;
#8997=CARTESIAN_POINT ( 'NONE',  ( 9.915538251416846194, 16.41143258624473233, -16.50493629029764264 ) ) ;
#8998=CARTESIAN_POINT ( 'NONE',  ( 9.641364314812712166, 17.66882920855936590, -17.90209449470656722 ) ) ;
#9003=CARTESIAN_POINT ( 'NONE',  ( 12.92285173585636215, 9.540162674316999158, -16.07191862488577527 ) ) ;
#9005=CARTESIAN_POINT ( 'NONE',  ( 36.54859390953723874, -21.18451583373416014, -14.99999999999999822 ) ) ;
#9006=CARTESIAN_POINT ( 'NONE',  ( 26.87257363757477435, -3.324124212371978082, -16.68573618535388547 ) ) ;
#9010=CARTESIAN_POINT ( 'NONE',  ( 27.20456514074317056, -5.347416052021189081, -13.22196079581408235 ) ) ;
#9011=CARTESIAN_POINT ( 'NONE',  ( 25.92522129715230506, 0.6472387150544522960, -15.98534533675435299 ) ) ;
#9013=EDGE_LOOP ( 'NONE', ( #11764, #23071, #25959, #4467 ) ) ;
#9023=CARTESIAN_POINT ( 'NONE',  ( 12.49899259368311988, 8.570259324921714494, -15.13097775544467005 ) ) ;
#9025=CARTESIAN_POINT ( 'NONE',  ( 30.62762753239542590, -8.735908549479720620, -17.37160549233551876 ) ) ;
#9029=CARTESIAN_POINT ( 'NONE',  ( 9.641350810849047548, 17.66889113945805789, -17.98596209335946128 ) ) ;
#9031=CARTESIAN_POINT ( 'NONE',  ( 15.15242361522499692, 5.855521407460130057, -16.92275779674541170 ) ) ;
#9034=CARTESIAN_POINT ( 'NONE',  ( 27.31974442496251143, -5.660127319198639206, -14.41990313654811651 ) ) ;
#9038=CARTESIAN_POINT ( 'NONE',  ( 12.24912255266251293, 9.517392596235749735, -15.33016477413064393 ) ) ;
#9040=CARTESIAN_POINT ( 'NONE',  ( 35.54859390953724585, -22.18451583373416014, -18.06010107863414405 ) ) ;
#9041=CARTESIAN_POINT ( 'NONE',  ( 14.79111372287554715, 6.954724682967856175, -19.27298399620107361 ) ) ;
#9044=CARTESIAN_POINT ( 'NONE',  ( 23.12480016457037379, 1.528454477237789488, -15.53356264363713102 ) ) ;
#9047=CARTESIAN_POINT ( 'NONE',  ( 28.15263004948277725, -12.62334012340276779, -12.05588540746726345 ) ) ;
#9048=CARTESIAN_POINT ( 'NONE',  ( 27.67597367917761630, -6.185689562215541670, -12.94745500973225383 ) ) ;
#9063=CARTESIAN_POINT ( 'NONE',  ( 26.30156876094583396, -3.312801620251602852, -13.23872229457767169 ) ) ;
#9064=CARTESIAN_POINT ( 'NONE',  ( 19.42071131597032974, 7.574497315622086724, -15.00200944635056644 ) ) ;
#9065=CARTESIAN_POINT ( 'NONE',  ( 33.88611015167484197, -15.71585695178754882, -20.89774115172086510 ) ) ;
#9067=CARTESIAN_POINT ( 'NONE',  ( 11.47269659055779378, 9.270105954394804115, -15.86098659800193644 ) ) ;
#9071=CARTESIAN_POINT ( 'NONE',  ( 9.671924655352764688, 16.20877460471870535, -17.88339855620073848 ) ) ;
#9075=CARTESIAN_POINT ( 'NONE',  ( 12.48484057295006977, 8.564241722236854315, -15.14223913367768759 ) ) ;
#9082=CARTESIAN_POINT ( 'NONE',  ( 16.53342136567307108, 10.04554801986687629, -15.32032680638607047 ) ) ;
#9085=CARTESIAN_POINT ( 'NONE',  ( 9.112530393872706469, 16.18137232441842954, -17.05472470070859714 ) ) ;
#9086=CARTESIAN_POINT ( 'NONE',  ( 32.41494245136814811, -10.61148775487728813, -19.57799680467864789 ) ) ;
#9088=CARTESIAN_POINT ( 'NONE',  ( 15.90442531705523876, 3.007083446286336947, -19.83189509879157697 ) ) ;
#9089=CARTESIAN_POINT ( 'NONE',  ( 17.75014749421169213, 9.747325538739326944, -14.55496937630740639 ) ) ;
#9091=CARTESIAN_POINT ( 'NONE',  ( 24.13298513268436452, -7.720266465098472253, -12.91035621449759496 ) ) ;
#9097=EDGE_LOOP ( 'NONE', ( #19962, #19464 ) ) ;
#9101=CARTESIAN_POINT ( 'NONE',  ( 34.19542162461613799, -15.10542955289956346, -18.90659549333309286 ) ) ;
#9102=CARTESIAN_POINT ( 'NONE',  ( 10.66819573146529621, 9.046892785011555915, -16.41140230749465800 ) ) ;
#9104=CARTESIAN_POINT ( 'NONE',  ( 26.47511176763426377, -7.718147522161595830, -18.64721581247919602 ) ) ;
#9106=CARTESIAN_POINT ( 'NONE',  ( 10.45306510330410177, 16.53912159438435125, -17.34933906371858114 ) ) ;
#9115=CARTESIAN_POINT ( 'NONE',  ( 9.661901852922078149, 16.25474045427587200, -17.91339448853296901 ) ) ;
#9118=CARTESIAN_POINT ( 'NONE',  ( 22.28228072301589080, -4.238876526682920698, -17.70252831752424427 ) ) ;
#9119=CARTESIAN_POINT ( 'NONE',  ( 22.53049847760648561, -4.001888697258268124, -18.07502562731026075 ) ) ;
#9120=CARTESIAN_POINT ( 'NONE',  ( 22.90957683611224738, 2.308586283387667581, -16.61139769879808625 ) ) ;
#9127=CARTESIAN_POINT ( 'NONE',  ( 26.87257363757477435, -3.324124212371978082, -16.68573618535388547 ) ) ;
#9133=CARTESIAN_POINT ( 'NONE',  ( 10.35953768210033665, 16.96805026999784616, -17.84385765891457254 ) ) ;
#9140=CARTESIAN_POINT ( 'NONE',  ( 16.21960234321935701, 7.070186740785398882, -14.59618053200276044 ) ) ;
#9141=CARTESIAN_POINT ( 'NONE',  ( 11.27495124880614163, 16.68260362121340279, -16.78505081266910182 ) ) ;
#9145=CARTESIAN_POINT ( 'NONE',  ( 9.643509238790151983, 17.65899231378470446, -17.74106871770035099 ) ) ;
#9146=CARTESIAN_POINT ( 'NONE',  ( 12.76023694501680517, 7.627675785621035764, -14.92276157399860281 ) ) ;
#9153=CARTESIAN_POINT ( 'NONE',  ( 10.37265302513970688, 16.90790163500151166, -17.63730412279738147 ) ) ;
#9154=CARTESIAN_POINT ( 'NONE',  ( 36.54859286093297754, -21.18451112290966165, -18.39168789611893118 ) ) ;
#9155=CARTESIAN_POINT ( 'NONE',  ( 25.71553203045151292, -8.406338935355361031, -18.42709291467145150 ) ) ;
#9163=CARTESIAN_POINT ( 'NONE',  ( 17.81745789538532776, 7.988559130291253751, -20.18242036267038841 ) ) ;
#9166=CARTESIAN_POINT ( 'NONE',  ( 25.25929662509423324, 0.6462067467026075818, -14.45468018858982795 ) ) ;
#9176=CARTESIAN_POINT ( 'NONE',  ( 10.38540050948072846, 18.16934103347302454, -16.97553146008864289 ) ) ;
#9181=CARTESIAN_POINT ( 'NONE',  ( 11.47155695691762212, 9.275332456566969697, -15.86145787682774078 ) ) ;
#9183=CARTESIAN_POINT ( 'NONE',  ( 16.42791133306356599, 6.383902638027607601, -15.35376453018263199 ) ) ;
#9186=CARTESIAN_POINT ( 'NONE',  ( 26.07968421886551980, -9.001936657367064498, -13.61655714643126913 ) ) ;
#9191=CARTESIAN_POINT ( 'NONE',  ( 11.05541533671906684, 17.68942329836457361, -17.91521986731755334 ) ) ;
#9194=CARTESIAN_POINT ( 'NONE',  ( 33.33926371295168423, -12.28475995124076903, -19.67523791759492013 ) ) ;
#9197=CARTESIAN_POINT ( 'NONE',  ( 23.02024704684396283, -2.230829994151436679, -18.49515006079944612 ) ) ;
#9200=CARTESIAN_POINT ( 'NONE',  ( 19.54218497767158169, 4.227554098413554229, -14.22708607227295730 ) ) ;
#9201=CARTESIAN_POINT ( 'NONE',  ( 27.56197131007709444, -12.41890123633259435, -14.84244373703855935 ) ) ;
#9212=CARTESIAN_POINT ( 'NONE',  ( 9.920751600319857033, 16.38752350362809551, -16.50277044458016107 ) ) ;
#9213=CARTESIAN_POINT ( 'NONE',  ( 27.68278592340041655, -3.068913841971319112, -15.41105173719521915 ) ) ;
#9214=CARTESIAN_POINT ( 'NONE',  ( 16.02150382621726976, 6.204807860950024789, -14.00014022580063155 ) ) ;
#9215=CARTESIAN_POINT ( 'NONE',  ( 36.51148101492068321, -23.01778725746827803, -19.37219236604238759 ) ) ;
#9220=CARTESIAN_POINT ( 'NONE',  ( 17.32695330507268494, 5.471673316493076200, -20.08600194542987794 ) ) ;
#9223=CARTESIAN_POINT ( 'NONE',  ( 10.33811693838771717, 18.38618951776012267, -17.97192418671890835 ) ) ;
#9228=CARTESIAN_POINT ( 'NONE',  ( 14.57776618122778700, 6.338444840345393239, -15.85465340776532095 ) ) ;
#9232=CARTESIAN_POINT ( 'NONE',  ( 35.54859390953724585, -23.18451583373416014, -18.19919658220850422 ) ) ;
#9233=CARTESIAN_POINT ( 'NONE',  ( 15.68163020692053422, 2.793964495486057409, -19.44966893625607085 ) ) ;
#9234=CARTESIAN_POINT ( 'NONE',  ( 18.31728471214517029, 9.901174664208697962, -15.18855771585127634 ) ) ;
#9238=EDGE_CURVE ( 'NONE', #14962, #24264, #13487, .T. ) ;
#9239=CARTESIAN_POINT ( 'NONE',  ( 20.46682838619579670, -4.770343855991169058, -14.23415315410508342 ) ) ;
#9251=CARTESIAN_POINT ( 'NONE',  ( 35.92974604556026463, -18.40436019371391652, -19.36057938427370217 ) ) ;
#9252=CARTESIAN_POINT ( 'NONE',  ( 10.66667607898454939, 9.053862104998891880, -16.41203073725236905 ) ) ;
#9256=CARTESIAN_POINT ( 'NONE',  ( 10.43477690885096720, 16.62299358534909288, -17.37687480348504820 ) ) ;
#9268=CARTESIAN_POINT ( 'NONE',  ( 9.667846996725693032, 16.22747526696303666, -17.88508502774671882 ) ) ;
#9270=CARTESIAN_POINT ( 'NONE',  ( 23.59026362060683724, -1.443753810951279082, -14.18444229111703514 ) ) ;
#9271=CARTESIAN_POINT ( 'NONE',  ( 24.16235420939608858, 2.058193855977920261, -15.89352170542055198 ) ) ;
#9272=CARTESIAN_POINT ( 'NONE',  ( 16.29141254853644227, 2.771581735061156682, -15.76764191790683611 ) ) ;
#9278=CARTESIAN_POINT ( 'NONE',  ( 23.63863231746517712, -2.790269051896475450, -19.68844555248840678 ) ) ;
#9288=CARTESIAN_POINT ( 'NONE',  ( 10.35864918915110877, 16.97212501191939538, -17.94384837343789485 ) ) ;
#9289=CARTESIAN_POINT ( 'NONE',  ( 35.54787733059053778, -22.18129662410796854, -18.46719521006932396 ) ) ;
#9291=CARTESIAN_POINT ( 'NONE',  ( 32.63711423693117553, -11.05166607373017484, -18.34576405707344549 ) ) ;
#9293=CARTESIAN_POINT ( 'NONE',  ( 12.82830918206423121, 7.509569466653498004, -16.13756579491948173 ) ) ;
#9297=CARTESIAN_POINT ( 'NONE',  ( 20.23291344124205793, 5.521974472852556381, -14.51730806008046137 ) ) ;
#9298=CARTESIAN_POINT ( 'NONE',  ( 11.28624536866114347, 16.63080734789289750, -16.78036754607827064 ) ) ;
#9299=CARTESIAN_POINT ( 'NONE',  ( 35.54502023521215648, -22.16846120802060938, -18.59538644662325524 ) ) ;
#9303=CARTESIAN_POINT ( 'NONE',  ( 9.641350810849047548, 17.66889113945805789, -17.91752729848689185 ) ) ;
#9306=CARTESIAN_POINT ( 'NONE',  ( 9.641351654859628084, 17.66888726871794191, -17.91235298298990841 ) ) ;
#9312=CARTESIAN_POINT ( 'NONE',  ( 10.36219267574928260, 16.95587413069128857, -17.77286471925143019 ) ) ;
#9315=CARTESIAN_POINT ( 'NONE',  ( 36.54859195715578579, -22.18450706271777406, -18.40832622446962930 ) ) ;
#9317=CARTESIAN_POINT ( 'NONE',  ( 26.80628776457338347, -3.176708023846821494, -16.02594779711905559 ) ) ;
#9322=CARTESIAN_POINT ( 'NONE',  ( 18.55323344277375242, 5.040171350539718098, -19.22783755317104237 ) ) ;
#9323=CARTESIAN_POINT ( 'NONE',  ( 27.33932411720343936, -8.205422078888220838, -18.29166945089792407 ) ) ;
#9329=CARTESIAN_POINT ( 'NONE',  ( 10.72588575366639674, 16.60783230186494563, -15.95209284586258214 ) ) ;
#9335=CARTESIAN_POINT ( 'NONE',  ( 11.47250673971808688, 9.270976631574885829, -15.86106510822916249 ) ) ;
#9338=CARTESIAN_POINT ( 'NONE',  ( 17.81918496738754953, 9.416330548141603529, -16.00206777915198586 ) ) ;
#9342=CARTESIAN_POINT ( 'NONE',  ( 29.72799312938100513, -7.689056491358781997, -15.42978383025728384 ) ) ;
#9345=CARTESIAN_POINT ( 'NONE',  ( 11.05610776857519184, 17.68624771760786274, -17.82814161748832760 ) ) ;
#9347=CARTESIAN_POINT ( 'NONE',  ( 35.54859390953724585, -22.18451583373416014, -17.64281456791166036 ) ) ;
#9348=CARTESIAN_POINT ( 'NONE',  ( 14.93287775521291394, 9.378568215907955974, -14.88591063491414168 ) ) ;
#9351=CARTESIAN_POINT ( 'NONE',  ( 25.66261690555348807, -4.931278859741150100, -13.05994810794548933 ) ) ;
#9354=CARTESIAN_POINT ( 'NONE',  ( 17.97606266963480692, 4.724414365053664966, -20.23074386977120298 ) ) ;
#9355=CARTESIAN_POINT ( 'NONE',  ( 16.67011857490315307, 4.279483903030143921, -15.63504347475558198 ) ) ;
#9364=CARTESIAN_POINT ( 'NONE',  ( 9.898178882064430084, 16.49104486689975246, -16.51464960819000893 ) ) ;
#9365=CARTESIAN_POINT ( 'NONE',  ( 24.68698569862014480, -7.792836496385216805, -13.74806253080685359 ) ) ;
#9366=CARTESIAN_POINT ( 'NONE',  ( 22.28231863826031756, 1.183864898644814811, -18.90614694914491167 ) ) ;
#9368=CARTESIAN_POINT ( 'NONE',  ( 31.50466570323033011, -10.22776944099620877, -17.14799365788790553 ) ) ;
#9376=CARTESIAN_POINT ( 'NONE',  ( 15.46244301724551740, 3.702889819443702990, -17.82701508041758842 ) ) ;
#9380=CARTESIAN_POINT ( 'NONE',  ( 10.33812163068573575, 18.38616799828327686, -17.90626694547636433 ) ) ;
#9385=CARTESIAN_POINT ( 'NONE',  ( 16.34386185847872142, 4.569898679961749366, -19.52586945278800812 ) ) ;
#9387=CARTESIAN_POINT ( 'NONE',  ( 27.68941694697105760, -11.75984073208553582, -11.85267853464266352 ) ) ;
#9389=CARTESIAN_POINT ( 'NONE',  ( 34.96958981470057637, -20.58335714263341387, -21.20026138435576613 ) ) ;
#9390=CARTESIAN_POINT ( 'NONE',  ( 25.36902537161520499, -2.228419832982303728, -15.31576610616191481 ) ) ;
#9391=CARTESIAN_POINT ( 'NONE',  ( 14.24687995347741420, 8.287322832548987606, -13.87414582376881000 ) ) ;
#9393=CARTESIAN_POINT ( 'NONE',  ( 29.48152472672500579, -5.877396966218813468, -15.70213184580788379 ) ) ;
#9401=CARTESIAN_POINT ( 'NONE',  ( 36.54859390953724585, -21.18451583373416014, -18.19919658220850422 ) ) ;
#9402=CARTESIAN_POINT ( 'NONE',  ( 12.75517096047518173, 7.625437268557950787, -14.92679923539383680 ) ) ;
#9410=CARTESIAN_POINT ( 'NONE',  ( 10.47103768343372288, 16.45669705093847313, -17.33522727542475295 ) ) ;
#9419=CARTESIAN_POINT ( 'NONE',  ( 11.14294825671155209, 9.462472856991839265, -17.27507855072861176 ) ) ;
#9420=CARTESIAN_POINT ( 'NONE',  ( 27.25745087693901425, -5.581270904725432302, -18.17424208600867175 ) ) ;
#9421=CARTESIAN_POINT ( 'NONE',  ( 17.97606266963480692, 4.724414365053664966, -20.23074386977120298 ) ) ;
#9425=CARTESIAN_POINT ( 'NONE',  ( 23.77086030874127687, -7.150112426529108944, -14.59934731766091431 ) ) ;
#9434=CARTESIAN_POINT ( 'NONE',  ( 10.35887147716723611, 16.97110557074245563, -17.87975733919941845 ) ) ;
#9435=CARTESIAN_POINT ( 'NONE',  ( 35.32886446602115171, -21.19738783794349857, -20.03221113960638178 ) ) ;
#9436=CARTESIAN_POINT ( 'NONE',  ( 33.44337896868773186, -12.72690026786775341, -19.72159258799634074 ) ) ;
#9438=CARTESIAN_POINT ( 'NONE',  ( 8.944585198251687075, 16.95159039956950764, -17.91368623377419667 ) ) ;
#9442=CARTESIAN_POINT ( 'NONE',  ( 20.22088415693689356, -1.238650738454883493, -19.72259765018230482 ) ) ;
#9444=CARTESIAN_POINT ( 'NONE',  ( 11.27239417409149880, 16.69433069180593776, -16.78622300611779750 ) ) ;
#9449=CARTESIAN_POINT ( 'NONE',  ( 9.641351021852148762, 17.66889017177091503, -17.91406276888456617 ) ) ;
#9452=CARTESIAN_POINT ( 'NONE',  ( 9.915248083523094280, 16.41276333319327918, -16.50506225043874409 ) ) ;
#9458=CARTESIAN_POINT ( 'NONE',  ( 10.47401950373780899, 16.44302204293020964, -17.33397781699859053 ) ) ;
#9460=CARTESIAN_POINT ( 'NONE',  ( 36.54859390953724585, -22.18451583373416014, -17.99055332684694974 ) ) ;
#9461=CARTESIAN_POINT ( 'NONE',  ( 31.81434894052502571, -10.04473835610349575, -15.03854332269495764 ) ) ;
#9462=CARTESIAN_POINT ( 'NONE',  ( 26.36224721256908410, -8.875037662531589433, -13.49479840426202948 ) ) ;
#9467=CARTESIAN_POINT ( 'NONE',  ( 33.16581763841239194, -10.35476010881584052, -17.60936685258081624 ) ) ;
#9469=CARTESIAN_POINT ( 'NONE',  ( 18.16542447708646790, 4.701683080007062365, -19.22226433900947029 ) ) ;
#9470=CARTESIAN_POINT ( 'NONE',  ( 27.04128250769109698, -11.23896722199365961, -17.17396923023889244 ) ) ;
#9479=CARTESIAN_POINT ( 'NONE',  ( 10.73702987185851931, 16.55672395529124330, -15.94748436097269817 ) ) ;
#9484=CARTESIAN_POINT ( 'NONE',  ( 11.34314632229486364, 9.864239995495806212, -15.91456019135469013 ) ) ;
#9486=CARTESIAN_POINT ( 'NONE',  ( 19.07048665705943336, 2.338351316274200453, -13.70053041002553407 ) ) ;
#9489=CARTESIAN_POINT ( 'NONE',  ( 26.47511176763426377, -7.718147522161595830, -18.64721581247919602 ) ) ;
#9491=CARTESIAN_POINT ( 'NONE',  ( 11.08268301555968094, 17.56437024738003316, -17.37355016474266733 ) ) ;
#9493=CARTESIAN_POINT ( 'NONE',  ( 35.37054299657279444, -20.38462739797860479, -19.24905200684423789 ) ) ;
#9494=CARTESIAN_POINT ( 'NONE',  ( 17.32873655921053313, 10.26331207550778579, -16.20725374984683143 ) ) ;
#9498=CARTESIAN_POINT ( 'NONE',  ( 27.61464345320196045, -4.235915813641956795, -14.29244051139929894 ) ) ;
#9501=CARTESIAN_POINT ( 'NONE',  ( 21.26575470983302196, 3.903880982571942493, -18.68858533207590966 ) ) ;
#9502=CARTESIAN_POINT ( 'NONE',  ( 15.09270446591840731, 5.883488971450414162, -17.42782692652931331 ) ) ;
#9515=CARTESIAN_POINT ( 'NONE',  ( 9.655099948573186097, 17.60583584124798051, -17.48406748397995614 ) ) ;
#9516=CARTESIAN_POINT ( 'NONE',  ( 22.71651454236177514, -3.376241010138071541, -20.62701743264632270 ) ) ;
#9517=CARTESIAN_POINT ( 'NONE',  ( 21.59786356094703308, -0.7637721020719707710, -13.97513905925265298 ) ) ;
#9518=CARTESIAN_POINT ( 'NONE',  ( 33.18306031693006730, -12.55741664378837896, -20.68523176094931415 ) ) ;
#9524=CARTESIAN_POINT ( 'NONE',  ( 19.51440197245297270, 8.071880087464508691, -17.28625796899888201 ) ) ;
#9527=CARTESIAN_POINT ( 'NONE',  ( 10.71981169803933120, 16.63568869523268390, -15.95461020916288675 ) ) ;
#9533=CARTESIAN_POINT ( 'NONE',  ( 17.29421355564066332, 9.360779442694735053, -19.18964209290773937 ) ) ;
#9534=CARTESIAN_POINT ( 'NONE',  ( 29.81560109580191664, -6.784977964013398477, -14.56477501241906403 ) ) ;
#9536=CARTESIAN_POINT ( 'NONE',  ( 35.54859390954303677, -23.18451583373416014, -15.55638201429745848 ) ) ;
#9537=CARTESIAN_POINT ( 'NONE',  ( 22.98313442454129429, 1.505266882216666158, -15.27805348665062546 ) ) ;
#9539=CARTESIAN_POINT ( 'NONE',  ( 20.14628369065288993, 2.528829491441240584, -14.55248280469624866 ) ) ;
#9542=CARTESIAN_POINT ( 'NONE',  ( 30.15014520769674533, -9.019674524353797906, -15.19912247041013842 ) ) ;
#9552=AXIS2_PLACEMENT_3D ( 'NONE', #28215, #26499, #5117 ) ;
#9554=CARTESIAN_POINT ( 'NONE',  ( 34.55638066306561029, -12.23714146529668234, -18.94394112255963236 ) ) ;
#9556=CARTESIAN_POINT ( 'NONE',  ( 9.641350810849047548, 17.66889113945805789, -19.66666666666842644 ) ) ;
#9561=CARTESIAN_POINT ( 'NONE',  ( 10.73134732381016576, 15.26288385841099249, -17.22756371135774245 ) ) ;
#9571=CARTESIAN_POINT ( 'NONE',  ( 9.662182123323882266, 16.25345509848694547, -17.90638241064055336 ) ) ;
#9573=CARTESIAN_POINT ( 'NONE',  ( 24.53726495287250486, -4.893489461768670168, -18.28393818840952534 ) ) ;
#9574=CARTESIAN_POINT ( 'NONE',  ( 26.39122182234759961, -2.132411660323914049, -15.07701415690354274 ) ) ;
#9580=CARTESIAN_POINT ( 'NONE',  ( 26.04489551603160180, -6.130266781319400948, -13.71289979607875154 ) ) ;
#9592=CARTESIAN_POINT ( 'NONE',  ( 10.47169460192958645, 16.45368433897878191, -17.33494088278173351 ) ) ;
#9594=CARTESIAN_POINT ( 'NONE',  ( 34.11209566957792561, -15.73109017586260272, -19.92372960426217787 ) ) ;
#9596=CARTESIAN_POINT ( 'NONE',  ( 15.26446397285951839, 8.458903494591371697, -14.20561233965910297 ) ) ;
#9600=CARTESIAN_POINT ( 'NONE',  ( 18.80472905218952917, 2.352968372735388503, -20.19605574946481497 ) ) ;
#9601=CARTESIAN_POINT ( 'NONE',  ( 11.05552354607739929, 17.68892703645376585, -17.88069451076903249 ) ) ;
#9607=CARTESIAN_POINT ( 'NONE',  ( 9.644802874473198173, 17.65305953564175567, -17.69767226479352118 ) ) ;
#9609=CARTESIAN_POINT ( 'NONE',  ( 9.879812780108833792, 16.57527415160161510, -16.52987074417163527 ) ) ;
#9614=CARTESIAN_POINT ( 'NONE',  ( 10.47169460192958645, 16.45368433897878191, -17.33494088278173351 ) ) ;
#9618=CARTESIAN_POINT ( 'NONE',  ( 32.82219004228267778, -9.671386367997632405, -18.62901690529166743 ) ) ;
#9619=CARTESIAN_POINT ( 'NONE',  ( 17.30683543869610119, 10.98570342618945617, -17.92154440881979482 ) ) ;
#9620=CARTESIAN_POINT ( 'NONE',  ( 27.51942754507220812, -5.605608590038333006, -14.64806962472005658 ) ) ;
#9623=CARTESIAN_POINT ( 'NONE',  ( 34.52681913409613657, -13.10175273156466069, -19.97882978310374469 ) ) ;
#9624=CARTESIAN_POINT ( 'NONE',  ( 16.66981565813235733, 9.362922448895053762, -13.87743608138566920 ) ) ;
#9625=CARTESIAN_POINT ( 'NONE',  ( 27.79246359028025992, -7.761574269410560944, -18.12988733074048753 ) ) ;
#9638=CARTESIAN_POINT ( 'NONE',  ( 10.71678736308702362, 16.64955868083699997, -15.95594379117117434 ) ) ;
#9642=CARTESIAN_POINT ( 'NONE',  ( 9.915538251416846194, 16.41143258624473233, -16.50493629029764264 ) ) ;
#9644=CARTESIAN_POINT ( 'NONE',  ( 9.667620158929956631, 16.22851557400931455, -17.88520075955172572 ) ) ;
#9645=CARTESIAN_POINT ( 'NONE',  ( 23.16986854814090080, 3.028408164773654931, -18.83379972368585342 ) ) ;
#9648=CARTESIAN_POINT ( 'NONE',  ( 27.51942754507220812, -5.605608590038333006, -14.64806962472005658 ) ) ;
#9651=CARTESIAN_POINT ( 'NONE',  ( 11.05541573950045375, 17.68942145115775944, -17.91357985325011626 ) ) ;
#9654=CARTESIAN_POINT ( 'NONE',  ( 33.60099431436507444, -12.44312249125652414, -18.72218098825057098 ) ) ;
#9655=CARTESIAN_POINT ( 'NONE',  ( 16.75072914628186282, 8.771658487634226731, -19.67538163746542779 ) ) ;
#9657=CARTESIAN_POINT ( 'NONE',  ( 9.114604345319493817, 16.17186091871610287, -17.05386699646955861 ) ) ;
#9658=CARTESIAN_POINT ( 'NONE',  ( 31.00997733146710900, -7.209757123251725019, -15.04105334301871011 ) ) ;
#9662=CARTESIAN_POINT ( 'NONE',  ( 20.01918758985507196, 7.682949113293006782, -15.97060347488303123 ) ) ;
#9663=CARTESIAN_POINT ( 'NONE',  ( 16.64656040655037827, 6.484405094197702724, -15.29036880746224014 ) ) ;
#9673=CARTESIAN_POINT ( 'NONE',  ( 9.641359250860388030, 17.66885243249017634, -17.90483003768722625 ) ) ;
#9674=CARTESIAN_POINT ( 'NONE',  ( 28.95742876386502118, -9.428754790923060014, -17.52548735455339823 ) ) ;
#9675=CARTESIAN_POINT ( 'NONE',  ( 24.52508672555368463, -0.3756359333432500169, -18.08805785897195051 ) ) ;
#9676=CARTESIAN_POINT ( 'NONE',  ( 32.52689891806821265, -10.77327725507678302, -19.81022979934233064 ) ) ;
#9678=CARTESIAN_POINT ( 'NONE',  ( 12.50268541164654756, 8.571888915454989544, -15.12803469218787811 ) ) ;
#9681=CARTESIAN_POINT ( 'NONE',  ( 15.14574614762244487, 6.587483969391940697, -15.14885142785537830 ) ) ;
#9683=CARTESIAN_POINT ( 'NONE',  ( 10.72001338896670397, 16.63476371493014128, -15.95452473000899118 ) ) ;
#9688=CARTESIAN_POINT ( 'NONE',  ( 17.12833724908345800, 9.171387755021909172, -19.38714867094073213 ) ) ;
#9690=CARTESIAN_POINT ( 'NONE',  ( 15.78898853071975061, 11.08777142890889245, -14.37707943039971781 ) ) ;
#9692=CARTESIAN_POINT ( 'NONE',  ( 32.63711423693117553, -11.05166607373017484, -18.34576405707344549 ) ) ;
#9694=CARTESIAN_POINT ( 'NONE',  ( 20.77099883799555258, -1.523348603316126981, -18.27480029096593839 ) ) ;
#9695=CARTESIAN_POINT ( 'NONE',  ( 18.95088517700565944, -0.6660330538943091128, -18.51770762617101340 ) ) ;
#9697=CARTESIAN_POINT ( 'NONE',  ( 30.28771073495105881, -9.259452824753982014, -16.33981616121770131 ) ) ;
#9704=CARTESIAN_POINT ( 'NONE',  ( 34.71713976128472723, -12.95676249388076329, -18.99403759477717557 ) ) ;
#9706=CARTESIAN_POINT ( 'NONE',  ( 9.641404825192898542, 17.66864342279195199, -17.88841768828662282 ) ) ;
#9710=CARTESIAN_POINT ( 'NONE',  ( 12.02841764901576838, 9.314357472305010432, -16.69117924060192948 ) ) ;
#9724=CARTESIAN_POINT ( 'NONE',  ( 11.22146363488324283, 9.102391324313689580, -17.24260967991309101 ) ) ;
#9726=CARTESIAN_POINT ( 'NONE',  ( 23.91915341143258544, -8.806945430038833678, -17.38103690300000181 ) ) ;
#9727=CARTESIAN_POINT ( 'NONE',  ( 22.45293885382703536, -0.3771200753331621081, -14.01028023225368635 ) ) ;
#9733=CARTESIAN_POINT ( 'NONE',  ( 26.80628776457338347, -3.176708023846821494, -16.02594779711905559 ) ) ;
#9742=CARTESIAN_POINT ( 'NONE',  ( 11.94706930840425407, 9.687427868553587729, -16.72481990518296158 ) ) ;
#9744=CARTESIAN_POINT ( 'NONE',  ( 35.02155038278115740, -19.81678845073966500, -20.19863594638463411 ) ) ;
#9747=CARTESIAN_POINT ( 'NONE',  ( 16.49632153860815720, 9.003283391651189405, -13.22380011606493788 ) ) ;
#9750=CARTESIAN_POINT ( 'NONE',  ( 21.58242789233717573, 5.264303332692052528, -18.32037006577847293 ) ) ;
#9751=CARTESIAN_POINT ( 'NONE',  ( 12.84980237226573863, 9.516412629723424388, -16.12948954962132575 ) ) ;
#9754=EDGE_CURVE ( 'NONE', #29043, #4557, #16346, .T. ) ;
#9756=CARTESIAN_POINT ( 'NONE',  ( 11.43229926783177497, 9.455373222906182207, -15.87769231223556332 ) ) ;
#9759=CARTESIAN_POINT ( 'NONE',  ( 9.826288910175632552, 16.82074144182198694, -16.60662094963572244 ) ) ;
#9766=CARTESIAN_POINT ( 'NONE',  ( 10.47079889355419446, 16.45779217176459852, -17.33533584583738829 ) ) ;
#9768=CARTESIAN_POINT ( 'NONE',  ( 36.35800453371076202, -21.32829872614925648, -20.07395605779921155 ) ) ;
#9769=CARTESIAN_POINT ( 'NONE',  ( 26.57062215293289498, -11.41726559881178638, -18.09730928560479057 ) ) ;
#9770=CARTESIAN_POINT ( 'NONE',  ( 29.22485947447185595, -8.910266539455653501, -18.36689805200119707 ) ) ;
#9777=CARTESIAN_POINT ( 'NONE',  ( 31.69910715399011636, -11.01187737159756352, -14.44698884073069145 ) ) ;
#9779=CARTESIAN_POINT ( 'NONE',  ( 28.09155340820903390, -11.11649160481613130, -13.74484337247343824 ) ) ;
#9786=CARTESIAN_POINT ( 'NONE',  ( 12.27688791398868950, 9.494734666090453246, -15.31069919958039804 ) ) ;
#9793=CARTESIAN_POINT ( 'NONE',  ( 9.920751600319857033, 16.38752350362809551, -16.50277044458016107 ) ) ;
#9797=CARTESIAN_POINT ( 'NONE',  ( 19.77208840006000656, -0.3814412559078061982, -20.24210485642555568 ) ) ;
#9805=CARTESIAN_POINT ( 'NONE',  ( 11.28016675873817576, 16.65868462784220227, -16.78288126510920719 ) ) ;
#9807=CARTESIAN_POINT ( 'NONE',  ( 35.36378496564391583, -20.35426714484339783, -19.25178739305277631 ) ) ;
#9808=CARTESIAN_POINT ( 'NONE',  ( 17.33713706444265412, 0.9871066061555996418, -18.79342181739402307 ) ) ;
#9810=CARTESIAN_POINT ( 'NONE',  ( 9.112400085652602399, 16.18196993452624355, -17.05477891849903926 ) ) ;
#9811=CARTESIAN_POINT ( 'NONE',  ( 27.13218800474287207, -6.260320175479137106, -19.66075965151719984 ) ) ;
#9815=CARTESIAN_POINT ( 'NONE',  ( 18.72775033408030154, 1.433941090885695768, -19.03071139844121262 ) ) ;
#9816=CARTESIAN_POINT ( 'NONE',  ( 14.32261721435726542, 8.042684561749755545, -14.95628083625202542 ) ) ;
#9822=DIRECTION ( 'NONE',  ( -0.7172983783020616677, 0.6967661275386687336, 0.000000000000000000 ) ) ;
#9827=CARTESIAN_POINT ( 'NONE',  ( 9.919231947839115549, 16.39449282361540483, -16.50339887433786501 ) ) ;
#9828=CARTESIAN_POINT ( 'NONE',  ( 28.11208967899271371, -8.897075463600188527, -14.13618326516971990 ) ) ;
#9829=CARTESIAN_POINT ( 'NONE',  ( 19.47744964272635926, 1.166342761889149982, -14.46873920536258495 ) ) ;
#9830=CARTESIAN_POINT ( 'NONE',  ( 33.33926371295168423, -12.28475995124076903, -19.67523791759492013 ) ) ;
#9839=CARTESIAN_POINT ( 'NONE',  ( 19.05868480923028940, 8.129737193291200370, -16.02886444249750042 ) ) ;
#9843=CARTESIAN_POINT ( 'NONE',  ( 10.33811697311952216, 18.38618935847563307, -17.91478972043705298 ) ) ;
#9846=CARTESIAN_POINT ( 'NONE',  ( 17.54642605795894994, 9.676486402519270058, -18.74681543856335608 ) ) ;
#9847=CARTESIAN_POINT ( 'NONE',  ( 30.15790919126650138, -6.784097790808209183, -15.35074926656157324 ) ) ;
#9849=CARTESIAN_POINT ( 'NONE',  ( 33.10952763335142635, -11.62914684427059697, -19.38687730282833499 ) ) ;
#9850=CARTESIAN_POINT ( 'NONE',  ( 20.31058213454123162, -2.053861134507735109, -16.68646832148754200 ) ) ;
#9852=CARTESIAN_POINT ( 'NONE',  ( 20.55682936838109498, 0.8107970201405315658, -19.60370085144657182 ) ) ;
#9854=CARTESIAN_POINT ( 'NONE',  ( 25.61980203353413543, -10.24193911033393256, -18.22380977611897990 ) ) ;
#9863=CARTESIAN_POINT ( 'NONE',  ( 33.07549275714919901, -10.34104163876563831, -17.35407900654646340 ) ) ;
#9864=CARTESIAN_POINT ( 'NONE',  ( 12.75704675400704424, 7.626265983139092874, -14.92530421254393147 ) ) ;
#9868=CARTESIAN_POINT ( 'NONE',  ( 12.40302661446015264, 8.678734247659738443, -16.45371344743900366 ) ) ;
#9878=CARTESIAN_POINT ( 'NONE',  ( 11.20373435594124878, 9.183700057499073921, -17.24994136041982529 ) ) ;
#9879=CARTESIAN_POINT ( 'NONE',  ( 23.38178567734072999, -4.037937620979102249, -14.56836966348588369 ) ) ;
#9880=CARTESIAN_POINT ( 'NONE',  ( 24.59824444495380646, -5.013944910511990649, -19.70109713935865514 ) ) ;
#9894=CARTESIAN_POINT ( 'NONE',  ( 12.02799090998256304, 9.316311091778235465, -16.69135597610317134 ) ) ;
#9896=CARTESIAN_POINT ( 'NONE',  ( 33.40713826534622655, -12.56408340279653757, -19.71064172033093698 ) ) ;
#9898=CARTESIAN_POINT ( 'NONE',  ( 8.944584698556434788, 16.95159269123564272, -17.91535980893264224 ) ) ;
#9900=CARTESIAN_POINT ( 'NONE',  ( 22.29983652437130814, 0.6627547066652448304, -20.09853802436992964 ) ) ;
#9901=CARTESIAN_POINT ( 'NONE',  ( 12.86387084073970222, 9.514634738764476296, -16.11888650007813339 ) ) ;
#9905=CARTESIAN_POINT ( 'NONE',  ( 11.47231678315799464, 9.271847796573304379, -15.86114366194887815 ) ) ;
#9907=CARTESIAN_POINT ( 'NONE',  ( 9.916118674515717046, 16.40877069192658055, -16.50468880802031890 ) ) ;
#9912=CARTESIAN_POINT ( 'NONE',  ( 13.09018272752966716, 8.557097568986355540, -15.93847522207377310 ) ) ;
#9914=CARTESIAN_POINT ( 'NONE',  ( 32.57905638361870615, -9.615828745292011703, -17.95267489271534700 ) ) ;
#9915=CARTESIAN_POINT ( 'NONE',  ( 17.20878921875063838, 11.12208594754616975, -17.23123872766219833 ) ) ;
#9916=CARTESIAN_POINT ( 'NONE',  ( 29.88803641097454999, -7.968445601786871002, -16.75847372370488131 ) ) ;
#9921=CARTESIAN_POINT ( 'NONE',  ( 33.54536560287652946, -10.49856191242287373, -18.63199441812703583 ) ) ;
#9923=CARTESIAN_POINT ( 'NONE',  ( 20.37262416712335167, 4.106476634890254829, -18.27772908839511246 ) ) ;
#9924=CARTESIAN_POINT ( 'NONE',  ( 27.00739300205740889, -11.59555048707680847, -14.72185353022491050 ) ) ;
#9934=CARTESIAN_POINT ( 'NONE',  ( 12.27567800861033120, 9.500287468128719937, -15.31119923128196625 ) ) ;
#9939=CARTESIAN_POINT ( 'NONE',  ( 11.48249212886396897, 9.228508165798535501, -15.85668214399537845 ) ) ;
#9940=CARTESIAN_POINT ( 'NONE',  ( 17.37750100583229340, 1.587821987789380440, -15.03969266580305764 ) ) ;
#9946=CARTESIAN_POINT ( 'NONE',  ( 12.84002880955021197, 9.524163120117652426, -16.13635871874149430 ) ) ;
#9948=CARTESIAN_POINT ( 'NONE',  ( 33.25502826659400313, -11.79853993747392771, -18.08863679259532731 ) ) ;
#9949=CARTESIAN_POINT ( 'NONE',  ( 14.73401617531889229, 6.408058468588501810, -15.60580005407095960 ) ) ;
#9951=CARTESIAN_POINT ( 'NONE',  ( 22.14981412484149104, -6.473446789742020258, -15.39974742277494713 ) ) ;
#9955=CARTESIAN_POINT ( 'NONE',  ( 21.84445237452005628, 0.7298858868756038509, -19.18266460542251295 ) ) ;
#9956=CARTESIAN_POINT ( 'NONE',  ( 17.88967384018823026, 7.017424582044266224, -15.49508032100559696 ) ) ;
#9972=CARTESIAN_POINT ( 'NONE',  ( 11.47231678315799464, 9.271847796573304379, -15.86114366194887815 ) ) ;
#9973=CARTESIAN_POINT ( 'NONE',  ( 27.38292679376507266, -11.43094998702963849, -14.23096243513112036 ) ) ;
#9974=CARTESIAN_POINT ( 'NONE',  ( 22.83681518364245022, 2.349634567491368564, -16.30468554850739338 ) ) ;
#9975=CARTESIAN_POINT ( 'NONE',  ( 34.90271572771163733, -20.28292729397994876, -21.20502438346732887 ) ) ;
#9983=CARTESIAN_POINT ( 'NONE',  ( 23.76365953361780470, 2.837943588559999508, -16.54419024451982168 ) ) ;
#9985=CARTESIAN_POINT ( 'NONE',  ( 10.72042364955539284, 16.63288220757436164, -15.95435249082810003 ) ) ;
#9988=CARTESIAN_POINT ( 'NONE',  ( 18.80472905218952917, 2.352968372735388503, -20.19605574946481497 ) ) ;
#9989=CARTESIAN_POINT ( 'NONE',  ( 25.85217995398321378, -12.57279400931185620, -13.36530271656463320 ) ) ;
#9991=CARTESIAN_POINT ( 'NONE',  ( 34.96805304670973413, -19.57645325810014114, -20.18246498508359466 ) ) ;
#9993=CARTESIAN_POINT ( 'NONE',  ( 26.79503139269368006, -8.611318205148688065, -11.94858980718629304 ) ) ;
#9994=CARTESIAN_POINT ( 'NONE',  ( 17.84334503882807255, 1.539790780908459000, -16.51430848555953190 ) ) ;
#10008=CARTESIAN_POINT ( 'NONE',  ( 35.70376052765831787, -18.38912696963886617, -20.33459093173238941 ) ) ;
#10009=CARTESIAN_POINT ( 'NONE',  ( 9.641350810849047548, 17.66889113945805789, -17.91928203681695564 ) ) ;
#10013=CARTESIAN_POINT ( 'NONE',  ( 13.12174330432777047, 8.570030634161971861, -15.91339823077023929 ) ) ;
#10024=CARTESIAN_POINT ( 'NONE',  ( 11.22348983819090407, 9.093098897663914215, -17.24177177356946800 ) ) ;
#10026=CARTESIAN_POINT ( 'NONE',  ( 23.72538513773186608, -9.146839435613468794, -15.72061189943629600 ) ) ;
#10027=CARTESIAN_POINT ( 'NONE',  ( 24.00718893345771932, -1.002666751694005765, -18.91818096615087796 ) ) ;
#10041=CARTESIAN_POINT ( 'NONE',  ( 11.37973238226026318, 12.28930733048782642, -16.95943368139929319 ) ) ;
#10043=CARTESIAN_POINT ( 'NONE',  ( 33.60099431436507444, -12.44312249125652414, -18.72218098825057098 ) ) ;
#10045=CARTESIAN_POINT ( 'NONE',  ( 13.48814714115247249, 7.673917307032582791, -15.62136820872497545 ) ) ;
#10047=CARTESIAN_POINT ( 'NONE',  ( 24.92864811393110358, -0.2441600445015326137, -14.78813717129899885 ) ) ;
#10048=CARTESIAN_POINT ( 'NONE',  ( 12.84300253770136990, 9.521034635873322216, -16.13432743836305505 ) ) ;
#10053=CARTESIAN_POINT ( 'NONE',  ( 11.47293561586387867, 9.269010148984008879, -15.86088772249501666 ) ) ;
#10056=CARTESIAN_POINT ( 'NONE',  ( 9.893572868141015775, 16.51216863388285461, -16.51808063826580408 ) ) ;
#10061=CARTESIAN_POINT ( 'NONE',  ( 12.04525852301462585, 9.245982119944198274, -16.68353927915122981 ) ) ;
#10065=CARTESIAN_POINT ( 'NONE',  ( 35.81175537756147520, -19.87429062379433731, -21.40957262365663993 ) ) ;
#10066=CARTESIAN_POINT ( 'NONE',  ( 24.87127057246125972, -9.548149280147088191, -14.79180087847266556 ) ) ;
#10067=CARTESIAN_POINT ( 'NONE',  ( 17.15446488409023829, 10.64262399902749578, -18.76211774343175520 ) ) ;
#10070=CARTESIAN_POINT ( 'NONE',  ( 34.35798975979065517, -12.34328324435382207, -19.92780167937219815 ) ) ;
#10071=CARTESIAN_POINT ( 'NONE',  ( 19.90313213008900206, 2.415960287222779890, -14.54935787103550560 ) ) ;
#10072=CARTESIAN_POINT ( 'NONE',  ( 14.57776618122778700, 6.338444840345393239, -15.85465340776532095 ) ) ;
#10083=CARTESIAN_POINT ( 'NONE',  ( 10.88291651000981730, 15.88766923650820928, -15.88715510423204513 ) ) ;
#10088=CARTESIAN_POINT ( 'NONE',  ( 11.82447321682112751, 8.672047275158794477, -15.63808403058127006 ) ) ;
#10090=CARTESIAN_POINT ( 'NONE',  ( 16.47391574482200483, 4.481796633190492152, -18.19319569287263150 ) ) ;
#10097=CARTESIAN_POINT ( 'NONE',  ( 11.79482239888288042, 14.29840825880376265, -16.57005305382644877 ) ) ;
#10101=CARTESIAN_POINT ( 'NONE',  ( 32.72889690553877529, -10.93821547844579634, -14.37279655741261486 ) ) ;
#10102=CARTESIAN_POINT ( 'NONE',  ( 21.04385110482095200, 5.766204710259658306, -15.30406332615466347 ) ) ;
#10108=CARTESIAN_POINT ( 'NONE',  ( 16.06097560829885040, 7.604535090956617616, -20.76572858943923094 ) ) ;
#10111=CARTESIAN_POINT ( 'NONE',  ( 21.12965431673027794, -4.223434333162931154, -14.75790768142083031 ) ) ;
#10113=CARTESIAN_POINT ( 'NONE',  ( 17.50199379865806293, 2.211901401554522639, -18.92990045904890550 ) ) ;
#10124=CARTESIAN_POINT ( 'NONE',  ( 10.56508425215480074, 13.43253182900300402, -16.23631622730588830 ) ) ;
#10125=CARTESIAN_POINT ( 'NONE',  ( 28.43808809371321189, -7.037065510061861318, -17.41003659457544117 ) ) ;
#10126=CARTESIAN_POINT ( 'NONE',  ( 26.83671086236671144, -5.482767762337403816, -13.01846673106422436 ) ) ;
#10127=CARTESIAN_POINT ( 'NONE',  ( 35.54859390953724585, -23.18451583373416014, -17.22552805718784441 ) ) ;
#10135=CARTESIAN_POINT ( 'NONE',  ( 18.88762249820254624, 5.002188274287570735, -13.90571046850145542 ) ) ;
#10138=CARTESIAN_POINT ( 'NONE',  ( 12.27692691330339514, 9.494559429826583852, -15.31068279593241144 ) ) ;
#10142=CARTESIAN_POINT ( 'NONE',  ( 18.97268594440662426, -2.511067197207834667, -17.06021009607598415 ) ) ;
#10144=CARTESIAN_POINT ( 'NONE',  ( 18.39217644224905257, 0.04847210594158309072, -18.71474297224575878 ) ) ;
#10146=CARTESIAN_POINT ( 'NONE',  ( 35.02155038278115740, -19.81678845073966500, -20.19863594638463411 ) ) ;
#10148=CARTESIAN_POINT ( 'NONE',  ( 22.02790516022008660, -6.446180030103099590, -16.19395709203531197 ) ) ;
#10149=CARTESIAN_POINT ( 'NONE',  ( 19.60537025999656890, 4.505197036469223981, -15.34927506990110047 ) ) ;
#10162=CARTESIAN_POINT ( 'NONE',  ( 36.54222296954648641, -22.15589457513855010, -18.69601260479128513 ) ) ;
#10163=CARTESIAN_POINT ( 'NONE',  ( 9.870716668364401869, 16.61699007954640805, -16.53972800451630931 ) ) ;
#10166=CARTESIAN_POINT ( 'NONE',  ( 13.11546866977305825, 8.567317423965196355, -15.91839467484043880 ) ) ;
#10181=CARTESIAN_POINT ( 'NONE',  ( 11.22298328736398965, 9.095422004326360721, -17.24198125015536576 ) ) ;
#10183=CARTESIAN_POINT ( 'NONE',  ( 17.86674704105132605, 10.80914456302241788, -19.54358591003751755 ) ) ;
#10184=CARTESIAN_POINT ( 'NONE',  ( 24.52508672555368463, -0.3756359333432500169, -18.08805785897195051 ) ) ;
#10196=CARTESIAN_POINT ( 'NONE',  ( 11.89844042902047505, 9.910446108148166289, -16.74492965742949835 ) ) ;
#10197=CARTESIAN_POINT ( 'NONE',  ( 33.36629945566365052, -11.89386221509426633, -18.35752312617820081 ) ) ;
#10199=CARTESIAN_POINT ( 'NONE',  ( 10.02031722384195156, 12.01814620627372143, -16.67932286086919902 ) ) ;
#10200=CARTESIAN_POINT ( 'NONE',  ( 23.11440248821028831, -7.346120041196752659, -16.32852059634029018 ) ) ;
#10201=CARTESIAN_POINT ( 'NONE',  ( 12.83240265444113071, 9.539962209189782882, -16.14097488725632346 ) ) ;
#10206=CARTESIAN_POINT ( 'NONE',  ( 11.47250673971808688, 9.270976631574885829, -15.86106510822916249 ) ) ;
#10214=CARTESIAN_POINT ( 'NONE',  ( 12.02748425217687789, 9.318634685891279190, -16.69156549717016702 ) ) ;
#10217=CARTESIAN_POINT ( 'NONE',  ( 35.76309413546784555, -19.65568143964299352, -21.39484760613106573 ) ) ;
#10218=CARTESIAN_POINT ( 'NONE',  ( 22.64650317123243894, 5.657944777580039997, -17.08144094666319646 ) ) ;
#10219=CARTESIAN_POINT ( 'NONE',  ( 13.26656245924271005, 6.725567473591735457, -17.69027979179009691 ) ) ;
#10225=CARTESIAN_POINT ( 'NONE',  ( 19.18059203083059217, 2.087369379035357575, -14.72322290489779917 ) ) ;
#10226=CARTESIAN_POINT ( 'NONE',  ( 21.41025690189560748, 5.821651141963339882, -16.00656683556521998 ) ) ;
#10236=CARTESIAN_POINT ( 'NONE',  ( 12.27441163154304071, 9.506095234784829984, -15.31172292274672664 ) ) ;
#10240=CARTESIAN_POINT ( 'NONE',  ( 12.50140887008201851, 8.571324787501421127, -15.12905211845398412 ) ) ;
#10241=CARTESIAN_POINT ( 'NONE',  ( 10.60386377644718614, 9.341927331141327784, -16.43800583390468262 ) ) ;
#10248=CARTESIAN_POINT ( 'NONE',  ( 12.83021228909557010, 9.549978240774745331, -16.14188291223562288 ) ) ;
#10251=CARTESIAN_POINT ( 'NONE',  ( 35.54859390954303677, -21.18451583373416014, -15.55638201429745848 ) ) ;
#10253=CARTESIAN_POINT ( 'NONE',  ( 18.21616227284554057, 4.699354889203569918, -13.86658597208997179 ) ) ;
#10256=CARTESIAN_POINT ( 'NONE',  ( 19.42071131597032974, 7.574497315622086724, -15.00200944635056644 ) ) ;
#10261=CARTESIAN_POINT ( 'NONE',  ( 25.46127020808262387, -4.208148299910691392, -19.59612275642668777 ) ) ;
#10262=CARTESIAN_POINT ( 'NONE',  ( 20.43163981785493988, 0.2187255735321424754, -20.49791845872360341 ) ) ;
#10275=CARTESIAN_POINT ( 'NONE',  ( 9.936961226781097167, 16.31318409042999917, -16.49606719383117337 ) ) ;
#10276=CARTESIAN_POINT ( 'NONE',  ( 26.02011856185544048, -9.832954462109395166, -14.66174570188732140 ) ) ;
#10277=CARTESIAN_POINT ( 'NONE',  ( 28.56881743257453721, -8.627791766613455593, -12.78522491232925873 ) ) ;
#10278=CARTESIAN_POINT ( 'NONE',  ( 32.96569147872224903, -11.36116021242123608, -19.12347989294568151 ) ) ;
#10286=CARTESIAN_POINT ( 'NONE',  ( 17.96884874826282186, 1.586046385177752871, -19.67104016136476119 ) ) ;
#10290=CARTESIAN_POINT ( 'NONE',  ( 12.26073475921635669, 9.568819114670704451, -15.31737879056614737 ) ) ;
#10291=CARTESIAN_POINT ( 'NONE',  ( 33.17819505895439391, -11.78846528140086924, -19.49437495119144259 ) ) ;
#10293=CARTESIAN_POINT ( 'NONE',  ( 19.38992137333195842, 2.881095379261479739, -20.30776781288435373 ) ) ;
#10295=CARTESIAN_POINT ( 'NONE',  ( 19.69411524970139737, 8.437195840132273972, -14.56566581881308409 ) ) ;
#10297=CARTESIAN_POINT ( 'NONE',  ( 33.48796008207983022, -12.92717959506727965, -19.73506838908087246 ) ) ;
#10300=CARTESIAN_POINT ( 'NONE',  ( 31.00997733146710900, -7.209757123251725019, -15.04105334301871011 ) ) ;
#10302=CARTESIAN_POINT ( 'NONE',  ( 19.28943675834911531, -1.002762487816046155, -14.40755329178536037 ) ) ;
#10303=CARTESIAN_POINT ( 'NONE',  ( 29.62588713853392264, -10.65184931322849060, -12.76488833982454629 ) ) ;
#10314=CARTESIAN_POINT ( 'NONE',  ( 35.98907965336992731, -19.67091466371804742, -20.42083605867238205 ) ) ;
#10315=CARTESIAN_POINT ( 'NONE',  ( 11.31072706937237982, 10.01291882189198112, -15.92796669285280764 ) ) ;
#10318=CARTESIAN_POINT ( 'NONE',  ( 9.661883135045433946, 16.25482629684424296, -17.91562380025844803 ) ) ;
#10330=CARTESIAN_POINT ( 'NONE',  ( 13.16425014233558954, 7.550783913790151125, -15.87799427043765021 ) ) ;
#10331=CARTESIAN_POINT ( 'NONE',  ( 17.99586569009407455, 10.99629947005995767, -19.18704736271931210 ) ) ;
#10332=CARTESIAN_POINT ( 'NONE',  ( 30.78125299044525320, -8.317598597646391312, -16.28273480984023891 ) ) ;
#10349=CARTESIAN_POINT ( 'NONE',  ( 12.72883512080982804, 8.524354266104470668, -16.21679389071614352 ) ) ;
#10351=CARTESIAN_POINT ( 'NONE',  ( 35.45944968151609800, -21.78403803824750185, -19.54251958818673174 ) ) ;
#10353=CARTESIAN_POINT ( 'NONE',  ( 8.944914148442956403, 16.95008179206086396, -17.86239244656949765 ) ) ;
#10355=CARTESIAN_POINT ( 'NONE',  ( 23.61827771231835982, -0.6465389018800060672, -13.57143891608981612 ) ) ;
#10356=CARTESIAN_POINT ( 'NONE',  ( 12.83224840168406544, 9.540640483216481726, -16.14104089933701758 ) ) ;
#10361=CARTESIAN_POINT ( 'NONE',  ( 12.48799528366842360, 8.565546312597838607, -15.13973160209665991 ) ) ;
#10366=CARTESIAN_POINT ( 'NONE',  ( 11.89844042902047505, 9.910446108148166289, -16.74492965742949835 ) ) ;
#10368=CARTESIAN_POINT ( 'NONE',  ( 18.97315296117551497, 8.914538345978252565, -15.07232217507325345 ) ) ;
#10369=CARTESIAN_POINT ( 'NONE',  ( 15.57351372253994271, 10.71565324155555388, -15.28765949597478624 ) ) ;
#10373=CARTESIAN_POINT ( 'NONE',  ( 36.54859390953723874, -22.18451583373416014, -15.00000000000000000 ) ) ;
#10375=CARTESIAN_POINT ( 'NONE',  ( 18.46387099684246635, 2.251061286204190992, -18.51322769290417369 ) ) ;
#10376=CARTESIAN_POINT ( 'NONE',  ( 14.24706144987486667, 6.238427219560604087, -16.72753349211556184 ) ) ;
#10387=CARTESIAN_POINT ( 'NONE',  ( 12.11484812106508713, 10.23787383345373136, -15.37770804730690166 ) ) ;
#10392=CARTESIAN_POINT ( 'NONE',  ( 11.47372892693763902, 9.265404009280679531, -15.86055721330185619 ) ) ;
#10395=CARTESIAN_POINT ( 'NONE',  ( 10.65249265583095095, 9.118909091547207524, -16.41789608165773728 ) ) ;
#10401=CARTESIAN_POINT ( 'NONE',  ( 12.83198842527593087, 9.541832653742346793, -16.14114841745374562 ) ) ;
#10402=CARTESIAN_POINT ( 'NONE',  ( 34.71713976128472723, -12.95676249388076329, -18.99403759477717557 ) ) ;
#10403=CARTESIAN_POINT ( 'NONE',  ( 21.58242789233717573, 5.264303332692052528, -18.32037006577847293 ) ) ;
#10407=CARTESIAN_POINT ( 'NONE',  ( 13.98191416104776685, 5.331502061239655532, -16.22335970869868760 ) ) ;
#10412=CARTESIAN_POINT ( 'NONE',  ( 23.07678757892180244, -0.1267571646896241688, -14.23703129728563965 ) ) ;
#10413=CARTESIAN_POINT ( 'NONE',  ( 21.41414477019618090, -0.8106431452899078849, -12.56463806509592018 ) ) ;
#10422=CARTESIAN_POINT ( 'NONE',  ( 9.957223259857686415, 16.22025982393231303, -16.48768813039480818 ) ) ;
#10423=CARTESIAN_POINT ( 'NONE',  ( 16.09764958744793262, 8.143416238145906760, -19.84970969296679044 ) ) ;
#10424=CARTESIAN_POINT ( 'NONE',  ( 22.24201797625671517, -7.474445146391827777, -15.38054711335415803 ) ) ;
#10432=CARTESIAN_POINT ( 'NONE',  ( 20.24985932600369409, 3.694099309552050237, -20.13309853732883781 ) ) ;
#10435=CARTESIAN_POINT ( 'NONE',  ( 12.27681432698556918, 9.495076167121005994, -15.31072932366845407 ) ) ;
#10439=CARTESIAN_POINT ( 'NONE',  ( 23.16390915794477223, 2.882539813099532555, -14.99485278278146438 ) ) ;
#10442=CARTESIAN_POINT ( 'NONE',  ( 18.04051923446642292, -0.4597542321540471488, -16.60176153622942508 ) ) ;
#10446=DIRECTION ( 'NONE',  ( 1.000000000000000000, 0.000000000000000000, 0.000000000000000000 ) ) ;
#10447=CARTESIAN_POINT ( 'NONE',  ( 30.62308825650849187, -7.210737555064373083, -14.15269394828060889 ) ) ;
#10449=CARTESIAN_POINT ( 'NONE',  ( 20.16317987096495656, -0.6177526724804084379, -13.65447574297484223 ) ) ;
#10461=CARTESIAN_POINT ( 'NONE',  ( 34.39307579391925174, -12.50091474996580487, -19.93840237985029162 ) ) ;
#10462=CARTESIAN_POINT ( 'NONE',  ( 10.04637620539468124, 15.81139305134258599, -16.45082025127570091 ) ) ;
#10465=CARTESIAN_POINT ( 'NONE',  ( 9.661883107508126400, 16.25482642313383508, -17.91565355200308218 ) ) ;
#10476=CARTESIAN_POINT ( 'NONE',  ( 13.38350887602579142, 7.627675785621035764, -15.70476675302002612 ) ) ;
#10479=CARTESIAN_POINT ( 'NONE',  ( 29.95565488329840775, -10.73317148848732039, -11.80569981112315325 ) ) ;
#10481=CARTESIAN_POINT ( 'NONE',  ( 26.00956027078203192, -8.595392566010074731, -19.46287731774799212 ) ) ;
#10494=CARTESIAN_POINT ( 'NONE',  ( 12.90142504057275197, 8.513187104919181181, -16.08590544042818493 ) ) ;
#10495=CARTESIAN_POINT ( 'NONE',  ( 32.01580575020638975, -11.60503005433848500, -14.58926670671732673 ) ) ;
#10498=CARTESIAN_POINT ( 'NONE',  ( 9.111692801717447665, 16.18521362881060455, -17.05508072787638696 ) ) ;
#10499=CARTESIAN_POINT ( 'NONE',  ( 24.79644250101478065, -1.608028467720058918, -19.02763285027648976 ) ) ;
#10500=CARTESIAN_POINT ( 'NONE',  ( 12.86924247997729687, 9.516471784987144744, -16.11464614809275631 ) ) ;
#10506=CARTESIAN_POINT ( 'NONE',  ( 11.47395765415086188, 9.264374527449886543, -15.86046114005151075 ) ) ;
#10512=CARTESIAN_POINT ( 'NONE',  ( 12.02780084644370007, 9.317182744227245905, -16.69143457430396893 ) ) ;
#10514=CARTESIAN_POINT ( 'NONE',  ( 14.47211339546095488, 7.927559549074161716, -19.99378091926031686 ) ) ;
#10515=CARTESIAN_POINT ( 'NONE',  ( 15.30633068984937317, 3.801504677414661693, -19.72534293519717608 ) ) ;
#10524=CARTESIAN_POINT ( 'NONE',  ( 36.54859390953724585, -22.18451583373416014, -17.78191007148576475 ) ) ;
#10526=CARTESIAN_POINT ( 'NONE',  ( 17.54642605795894994, 9.676486402519270058, -18.74681543856335608 ) ) ;
#10536=CARTESIAN_POINT ( 'NONE',  ( 11.05541531668977662, 17.68942339022145305, -17.91664992932185996 ) ) ;
#10542=CARTESIAN_POINT ( 'NONE',  ( 11.47304865262203499, 9.268493388164605662, -15.86084085272616484 ) ) ;
#10545=CARTESIAN_POINT ( 'NONE',  ( 11.11829553246053770, 8.091015213210848600, -16.14073874907621331 ) ) ;
#10552=CARTESIAN_POINT ( 'NONE',  ( 12.70256148071318414, 10.13540111970991653, -16.19467101188346092 ) ) ;
#10554=CARTESIAN_POINT ( 'NONE',  ( 33.45149595566165601, -11.04796323883829423, -16.41509932566969354 ) ) ;
#10555=CARTESIAN_POINT ( 'NONE',  ( 22.16846437878366061, -4.107540447007581363, -19.06500358040360865 ) ) ;
#10561=CARTESIAN_POINT ( 'NONE',  ( 16.94700227795405212, 10.49100606271714931, -14.51747230701220559 ) ) ;
#10567=CARTESIAN_POINT ( 'NONE',  ( 20.05514754915220266, -1.452567280579552866, -14.87399747198034738 ) ) ;
#10568=CARTESIAN_POINT ( 'NONE',  ( 18.07093408371026300, -2.157424655934858215, -16.53044640867639359 ) ) ;
#10579=CARTESIAN_POINT ( 'NONE',  ( 11.45661370752365116, 9.343864103108954211, -15.86763743611193789 ) ) ;
#10580=CARTESIAN_POINT ( 'NONE',  ( 26.39122182234759961, -2.132411660323914049, -15.07701415690354274 ) ) ;
#10589=CARTESIAN_POINT ( 'NONE',  ( 20.51249478307574847, 1.942573248051725709, -13.31196225760961838 ) ) ;
#10593=CARTESIAN_POINT ( 'NONE',  ( 12.27691367651725862, 9.494620545951883983, -15.31068823849801319 ) ) ;
#10595=CARTESIAN_POINT ( 'NONE',  ( 32.48283477683061449, -11.02614750807341260, -17.91093295056291979 ) ) ;
#10597=CARTESIAN_POINT ( 'NONE',  ( 19.12501085131992085, -2.578449613843157184, -15.80510918775627438 ) ) ;
#10599=CARTESIAN_POINT ( 'NONE',  ( 21.82606822486871323, 1.157895394498012154, -14.17951425939655508 ) ) ;
#10604=CARTESIAN_POINT ( 'NONE',  ( 23.86193934616450818, -4.638293873783104537, -19.03466029786466152 ) ) ;
#10606=CARTESIAN_POINT ( 'NONE',  ( 24.13298513268436452, -7.720266465098472253, -12.91035621449759496 ) ) ;
#10618=CARTESIAN_POINT ( 'NONE',  ( 29.60394739741320080, -6.827861936862228198, -14.22031441372854843 ) ) ;
#10621=CARTESIAN_POINT ( 'NONE',  ( 36.54859195715578579, -22.18450706271777406, -18.40832622446962930 ) ) ;
#10623=CARTESIAN_POINT ( 'NONE',  ( 9.917965570771830386, 16.40030059027150600, -16.50392256580263606 ) ) ;
#10626=CARTESIAN_POINT ( 'NONE',  ( 9.661883061612440926, 16.25482663361732705, -21.33333333332589632 ) ) ;
#10629=CARTESIAN_POINT ( 'NONE',  ( 9.932908820165812003, 16.33176894372950727, -16.49774300651844072 ) ) ;
#10637=CARTESIAN_POINT ( 'NONE',  ( 13.38012098442259834, 7.626178612778168109, -15.70746696265163145 ) ) ;
#10640=CARTESIAN_POINT ( 'NONE',  ( 28.80153578082395427, -7.039779562103731791, -13.29052886957691371 ) ) ;
#10641=CARTESIAN_POINT ( 'NONE',  ( 28.56881743257453721, -8.627791766613455593, -12.78522491232925873 ) ) ;
#10652=CARTESIAN_POINT ( 'NONE',  ( 13.11546866977305825, 8.567317423965196355, -15.91839467484043880 ) ) ;
#10655=CARTESIAN_POINT ( 'NONE',  ( 33.25502826659400313, -11.79853993747392771, -18.08863679259532731 ) ) ;
#10658=CARTESIAN_POINT ( 'NONE',  ( 9.112637166705713554, 16.18088265059586561, -17.05468042929993189 ) ) ;
#10662=CARTESIAN_POINT ( 'NONE',  ( 25.36810815240369621, -0.9165050883202133791, -18.11329069065276443 ) ) ;
#10663=CARTESIAN_POINT ( 'NONE',  ( 13.08618951557147803, 9.612344561400664844, -15.94173553134588595 ) ) ;
#10670=CARTESIAN_POINT ( 'NONE',  ( 11.49350937636955372, 9.187954247928445284, -15.85136552863131421 ) ) ;
#10675=CARTESIAN_POINT ( 'NONE',  ( 9.661883061612440926, 16.25482663361732705, -17.97192418671890835 ) ) ;
#10677=CARTESIAN_POINT ( 'NONE',  ( 13.34169928452473819, 6.621333031661079005, -16.53230918748570488 ) ) ;
#10678=CARTESIAN_POINT ( 'NONE',  ( 17.03934835405440751, -0.5873649402599611102, -16.44458879923593742 ) ) ;
#10681=CARTESIAN_POINT ( 'NONE',  ( 36.54859390953724585, -22.18451583373416014, -16.11276402859391865 ) ) ;
#10683=CARTESIAN_POINT ( 'NONE',  ( 18.76632379254337835, 6.868107169226369102, -19.55161205380106892 ) ) ;
#10685=MECHANICAL_DESIGN_GEOMETRIC_PRESENTATION_REPRESENTATION('',(#19945),#25820);
#10691=CARTESIAN_POINT ( 'NONE',  ( 33.96943610671532809, -15.09019632882451134, -19.88060704079178720 ) ) ;
#10698=CARTESIAN_POINT ( 'NONE',  ( 12.46291758456249354, 9.612344561400664844, -15.15973035232449462 ) ) ;
#10704=CARTESIAN_POINT ( 'NONE',  ( 10.74080116101666427, 8.781381604732478863, -16.37623182050610993 ) ) ;
#10709=CARTESIAN_POINT ( 'NONE',  ( 12.86826794643883609, 9.516041646402381815, -16.11542282846662388 ) ) ;
#10710=CARTESIAN_POINT ( 'NONE',  ( 36.27242973171742335, -19.94385647102418702, -19.46417027601260230 ) ) ;
#10711=CARTESIAN_POINT ( 'NONE',  ( 21.79935899731381710, -1.430375723040585356, -13.25318265510616733 ) ) ;
#10717=CARTESIAN_POINT ( 'NONE',  ( 26.06583011202948441, -9.749651170145462231, -12.94692625511877182 ) ) ;
#10718=CARTESIAN_POINT ( 'NONE',  ( 20.52698940127687877, 5.222567878441341627, -18.38034891569893503 ) ) ;
#10730=EDGE_CURVE ( 'NONE', #29043, #24264, #12634, .T. ) ;
#10732=CARTESIAN_POINT ( 'NONE',  ( 11.22518019566232716, 9.085373951847735441, -17.24107067304604257 ) ) ;
#10734=CARTESIAN_POINT ( 'NONE',  ( 10.33811693838771717, 18.38618951776012267, -17.92981046679734547 ) ) ;
#10736=CARTESIAN_POINT ( 'NONE',  ( 26.06583011202948441, -9.749651170145462231, -12.94692625511877182 ) ) ;
#10743=CARTESIAN_POINT ( 'NONE',  ( 9.907423389235603395, 16.44864837861227969, -16.50891839478055090 ) ) ;
#10746=CARTESIAN_POINT ( 'NONE',  ( 25.55230692589818631, -0.5649882819070038975, -17.32853901032857280 ) ) ;
#10749=CARTESIAN_POINT ( 'NONE',  ( 12.01759036229752553, 10.68391031264169122, -15.41792755180196473 ) ) ;
#10751=CARTESIAN_POINT ( 'NONE',  ( 32.68951927270060764, -11.07419627511998605, -18.48540492261787449 ) ) ;
#10753=CARTESIAN_POINT ( 'NONE',  ( 23.84106988684860440, -4.080291168153947545, -13.50610408985603250 ) ) ;
#10755=CARTESIAN_POINT ( 'NONE',  ( 15.57379856253263206, 2.175854586521385858, -15.33309735461106094 ) ) ;
#10758=CARTESIAN_POINT ( 'NONE',  ( 14.73435313093308174, 9.569269045654692718, -13.91804818168885305 ) ) ;
#10759=CARTESIAN_POINT ( 'NONE',  ( 21.36789492492977871, -4.378045371801569274, -13.15753336270543095 ) ) ;
#10762=CARTESIAN_POINT ( 'NONE',  ( 29.90031526554274777, -7.862644070287768905, -16.42500436498598049 ) ) ;
#10774=CARTESIAN_POINT ( 'NONE',  ( 24.88525782559502630, -5.606924519715485111, -13.99218633471889817 ) ) ;
#10776=CARTESIAN_POINT ( 'NONE',  ( 32.45862320860160821, -9.597537451891041016, -17.61229109800368064 ) ) ;
#10778=CARTESIAN_POINT ( 'NONE',  ( 9.932908820165812003, 16.33176894372950727, -16.49774300651844072 ) ) ;
#10781=CARTESIAN_POINT ( 'NONE',  ( 13.12468173219994760, 8.571325198882655982, -15.91105655537220009 ) ) ;
#10785=CARTESIAN_POINT ( 'NONE',  ( 9.920751600319857033, 16.38752350362809551, -16.50277044458016107 ) ) ;
#10793=CARTESIAN_POINT ( 'NONE',  ( 15.26446397285951839, 8.458903494591371697, -14.20561233965910297 ) ) ;
#10794=CARTESIAN_POINT ( 'NONE',  ( 31.83585693452864973, -10.27807049784803972, -18.08404909334234745 ) ) ;
#10795=CARTESIAN_POINT ( 'NONE',  ( 32.00807787192805876, -10.01600718589171990, -13.21854031764240389 ) ) ;
#10796=CARTESIAN_POINT ( 'NONE',  ( 24.16496757332932788, -10.42823604606268617, -16.34834267607407909 ) ) ;
#10805=CARTESIAN_POINT ( 'NONE',  ( 13.23272240178861381, 8.619070305187777947, -15.82494623455082916 ) ) ;
#10806=CARTESIAN_POINT ( 'NONE',  ( 33.63214571818804188, -11.07540017893869866, -16.92567501773416794 ) ) ;
#10808=CARTESIAN_POINT ( 'NONE',  ( 9.111869836743295537, 16.18440172361536611, -17.05500387803421702 ) ) ;
#10811=CARTESIAN_POINT ( 'NONE',  ( 25.07290406138036687, -9.006318079059196791, -17.79994936451110732 ) ) ;
#10812=CARTESIAN_POINT ( 'NONE',  ( 12.92285173585636215, 9.540162674316999158, -16.07191862488577527 ) ) ;
#10816=CARTESIAN_POINT ( 'NONE',  ( 11.47748818427356987, 9.248962635895034978, -15.85894168489154765 ) ) ;
#10821=CARTESIAN_POINT ( 'NONE',  ( 9.661883064511089358, 16.25482662032373327, -17.91571053624716470 ) ) ;
#10822=CARTESIAN_POINT ( 'NONE',  ( 19.51424001318473245, 7.885341048999412017, -19.79681821819610832 ) ) ;
#10823=CARTESIAN_POINT ( 'NONE',  ( 16.54285080251403173, 3.669380853427548939, -13.47387114519368012 ) ) ;
#10826=CARTESIAN_POINT ( 'NONE',  ( 35.91774987194125401, -19.35046774019819438, -20.39927477693754554 ) ) ;
#10829=CARTESIAN_POINT ( 'NONE',  ( 19.25770813156441008, -2.543370271471735222, -15.40753146551623587 ) ) ;
#10836=CARTESIAN_POINT ( 'NONE',  ( 33.44337896868773186, -12.72690026786775341, -19.72159258799634074 ) ) ;
#10841=CARTESIAN_POINT ( 'NONE',  ( 12.24562038388194551, 9.516309650702005740, -15.33292062045688908 ) ) ;
#10842=CARTESIAN_POINT ( 'NONE',  ( 34.74206752880779447, -19.56122003402509080, -21.15647653254228189 ) ) ;
#10845=CARTESIAN_POINT ( 'NONE',  ( 10.66743590522492369, 9.050377445005224786, -16.41171652237351353 ) ) ;
#10850=CARTESIAN_POINT ( 'NONE',  ( 10.35864918915110877, 16.97212501191939538, -21.33333333332589277 ) ) ;
#10851=CARTESIAN_POINT ( 'NONE',  ( 34.18187006836440389, -11.68445768601494628, -19.79758194388510972 ) ) ;
#10852=CARTESIAN_POINT ( 'NONE',  ( 21.57856661146780652, -4.666631351218505586, -18.28211233923166645 ) ) ;
#10862=CARTESIAN_POINT ( 'NONE',  ( 28.02603357813017482, -6.678172375388682802, -19.11289830413424440 ) ) ;
#10864=CARTESIAN_POINT ( 'NONE',  ( 27.32111546295355708, -6.651148440249742499, -13.76656720552121982 ) ) ;
#10874=CARTESIAN_POINT ( 'NONE',  ( 11.22423757029256741, 9.089670537749404033, -17.24146249637195183 ) ) ;
#10875=CARTESIAN_POINT ( 'NONE',  ( 12.49271550807400999, 8.567542729147559655, -15.13597632865050535 ) ) ;
#10876=CARTESIAN_POINT ( 'NONE',  ( 31.37220973900873489, -11.08107799475175348, -13.94606079199652982 ) ) ;
#10884=CARTESIAN_POINT ( 'NONE',  ( 22.51149892830068211, -1.106640851078940502, -13.23823320067571885 ) ) ;
#10888=CARTESIAN_POINT ( 'NONE',  ( 12.24670349824113380, 9.516721811805902931, -15.33206243003379754 ) ) ;
#10893=CARTESIAN_POINT ( 'NONE',  ( 27.83100014064079275, -5.545984359997562230, -15.13782040115233052 ) ) ;
#10895=CARTESIAN_POINT ( 'NONE',  ( 23.38119176934044674, -2.968156504308268495, -14.25447959695224043 ) ) ;
#10899=CARTESIAN_POINT ( 'NONE',  ( 32.15747877504752950, -11.00374777879112642, -13.30332049327740052 ) ) ;
#10900=CARTESIAN_POINT ( 'NONE',  ( 25.10166869626759123, -5.595937160916529152, -20.34551573546397307 ) ) ;
#10908=CARTESIAN_POINT ( 'NONE',  ( 24.78692427941192733, -9.284778175067517125, -17.23615439686343720 ) ) ;
#10913=CARTESIAN_POINT ( 'NONE',  ( 9.641350810849047548, 17.66889113945805789, -21.33333333332589277 ) ) ;
#10914=CARTESIAN_POINT ( 'NONE',  ( 23.39779239333391914, -5.936415184958717894, -17.60678703246490429 ) ) ;
#10915=CARTESIAN_POINT ( 'NONE',  ( 18.63710449947919301, 3.826706299981984305, -14.11708861520305192 ) ) ;
#10916=CARTESIAN_POINT ( 'NONE',  ( 34.40782828833705054, -13.56718989277036691, -20.98518325316450372 ) ) ;
#10918=CARTESIAN_POINT ( 'NONE',  ( 11.48890098693651396, 9.204103201752445784, -15.85365151319587440 ) ) ;
#10922=CARTESIAN_POINT ( 'NONE',  ( 9.661883061612440926, 16.25482663361732705, -17.98596209335946128 ) ) ;
#10925=CARTESIAN_POINT ( 'NONE',  ( 12.50396148805030627, 8.572452836447732594, -15.12701763676990119 ) ) ;
#10932=CARTESIAN_POINT ( 'NONE',  ( 8.944584683310379702, 16.95159276115599667, -17.97192418671890835 ) ) ;
#10933=CARTESIAN_POINT ( 'NONE',  ( 36.54859390953724585, -23.18451583373416014, -18.19919658220850422 ) ) ;
#10934=CARTESIAN_POINT ( 'NONE',  ( 20.90484242567171691, 8.469164366756103846, -17.19731680296963106 ) ) ;
#10936=CARTESIAN_POINT ( 'NONE',  ( 22.24201797625671517, -7.474445146391827777, -15.38054711335415803 ) ) ;
#10942=CARTESIAN_POINT ( 'NONE',  ( 22.90368100322821121, -1.908636692139587199, -20.53213217155426662 ) ) ;
#10951=CARTESIAN_POINT ( 'NONE',  ( 13.10707286029108865, 8.563798077496334926, -15.92507172258792281 ) ) ;
#10952=CARTESIAN_POINT ( 'NONE',  ( 33.69236230569678980, -11.08454582564024449, -17.09586691508924972 ) ) ;
#10954=CARTESIAN_POINT ( 'NONE',  ( 12.75200725638203281, 7.624046516185085665, -14.92932020320056452 ) ) ;
#10955=CARTESIAN_POINT ( 'NONE',  ( 27.91615220763155847, -6.225400021157185826, -17.67258836524805332 ) ) ;
#10956=CARTESIAN_POINT ( 'NONE',  ( 12.86830129319110405, 9.516055860257337073, -16.11539629037995169 ) ) ;
#10963=CARTESIAN_POINT ( 'NONE',  ( 12.50035968906703765, 8.570861208087439564, -15.12988832871674560 ) ) ;
#10967=CARTESIAN_POINT ( 'NONE',  ( 13.12404665403065707, 8.571044468271947991, -15.91156272984762765 ) ) ;
#10969=CARTESIAN_POINT ( 'NONE',  ( 23.69691533927305116, -2.951365702903132604, -18.66995449711026822 ) ) ;
#10970=CARTESIAN_POINT ( 'NONE',  ( 19.05076746314986025, 7.350425291474770084, -20.38782652337943446 ) ) ;
#10977=CARTESIAN_POINT ( 'NONE',  ( 19.12501085131992085, -2.578449613843157184, -15.80510918775627438 ) ) ;
#10988=CARTESIAN_POINT ( 'NONE',  ( 14.24706144987486667, 6.238427219560604087, -16.72753349211556184 ) ) ;
#10989=CARTESIAN_POINT ( 'NONE',  ( 12.24683531348137144, 9.516853939945930208, -15.33195173648645593 ) ) ;
#10990=CARTESIAN_POINT ( 'NONE',  ( 35.52583876341286384, -22.08228901593173177, -18.97221062538168113 ) ) ;
#10996=CARTESIAN_POINT ( 'NONE',  ( 9.641350810849047548, 17.66889113945805789, -19.66666666666842644 ) ) ;
#11003=CARTESIAN_POINT ( 'NONE',  ( 10.35864924400752862, 16.97212476034085782, -17.91519562840587199 ) ) ;
#11005=CARTESIAN_POINT ( 'NONE',  ( 32.11202735699620803, -10.19471129157119194, -14.63100864886716934 ) ) ;
#11006=CARTESIAN_POINT ( 'NONE',  ( 19.12501085131992085, -2.578449613843157184, -15.80510918775627438 ) ) ;
#11013=CARTESIAN_POINT ( 'NONE',  ( 29.02390443993225588, -5.138988301204332920, -16.36505798003706857 ) ) ;
#11014=CARTESIAN_POINT ( 'NONE',  ( 23.76792026503975919, -8.198361753721227885, -14.67730844950409441 ) ) ;
#11027=CARTESIAN_POINT ( 'NONE',  ( 13.31307029362551475, 7.598550302509940124, -15.76075481184169647 ) ) ;
#11028=CARTESIAN_POINT ( 'NONE',  ( 12.13006862794127017, 8.527244997094612700, -15.41586291625151972 ) ) ;
#11036=CARTESIAN_POINT ( 'NONE',  ( 9.745779815811758340, 17.18996641109745482, -16.82979807527155458 ) ) ;
#11042=CARTESIAN_POINT ( 'NONE',  ( 21.16681283796276603, -5.103637247178538061, -17.00692323485822754 ) ) ;
#11046=CARTESIAN_POINT ( 'NONE',  ( 11.05541531668977662, 17.68942339022145305, -17.92015940598198753 ) ) ;
#11047=CARTESIAN_POINT ( 'NONE',  ( 35.09336438560361415, -20.13941072448723801, -20.22035334018532637 ) ) ;
#11050=CARTESIAN_POINT ( 'NONE',  ( 23.22413189157496305, -7.367447486509826504, -15.63851824576001981 ) ) ;
#11052=CARTESIAN_POINT ( 'NONE',  ( 23.56326861202678202, -1.685860805813322427, -18.23406631578895798 ) ) ;
#11055=CARTESIAN_POINT ( 'NONE',  ( 13.51621490077814691, 9.019785729699995258, -14.32023381125561556 ) ) ;
#11057=CARTESIAN_POINT ( 'NONE',  ( 28.58746438791548528, -7.443717211345676432, -18.79719194573140584 ) ) ;
#11067=CARTESIAN_POINT ( 'NONE',  ( 9.641350810849047548, 17.66889113945805789, -17.92981046679734547 ) ) ;
#11068=CARTESIAN_POINT ( 'NONE',  ( 24.17451698631213475, -5.926886182136407832, -14.25952201372300365 ) ) ;
#11069=CARTESIAN_POINT ( 'NONE',  ( 17.20140313730510684, 4.016069822000726042, -19.84498366692964666 ) ) ;
#11071=CARTESIAN_POINT ( 'NONE',  ( 35.92571694232586310, -20.38625956716168020, -21.41712135977877907 ) ) ;
#11074=CARTESIAN_POINT ( 'NONE',  ( 12.49742530276927610, 8.569573706352677789, -15.13222638044318735 ) ) ;
#11079=CARTESIAN_POINT ( 'NONE',  ( 9.669898452045105230, 16.21806703136846295, -17.88423646254436861 ) ) ;
#11082=CARTESIAN_POINT ( 'NONE',  ( 11.77869587587188249, 8.711114196793760200, -15.67004689359726299 ) ) ;
#11089=CARTESIAN_POINT ( 'NONE',  ( 13.38265815842314943, 7.627299838292535661, -15.70544478996546900 ) ) ;
#11090=CARTESIAN_POINT ( 'NONE',  ( 35.92571694232586310, -20.38625956716168020, -21.41712135977877907 ) ) ;
#11091=CARTESIAN_POINT ( 'NONE',  ( 22.15888525254269581, 3.701285330253634154, -19.09944157575669621 ) ) ;
#11092=CARTESIAN_POINT ( 'NONE',  ( 15.40919527484693319, 5.754234090002595003, -19.70842740302703078 ) ) ;
#11096=CARTESIAN_POINT ( 'NONE',  ( 23.73516035876120611, -6.831976609072074602, -19.85773546425274105 ) ) ;
#11105=CARTESIAN_POINT ( 'NONE',  ( 35.37054299657279444, -20.38462739797860479, -19.24905200684423789 ) ) ;
#11107=CARTESIAN_POINT ( 'NONE',  ( 10.74080116101666427, 8.781381604732478863, -16.37623182050610993 ) ) ;
#11112=CARTESIAN_POINT ( 'NONE',  ( 25.26806593431409453, -8.821542497490490575, -18.05414547114721557 ) ) ;
#11115=CARTESIAN_POINT ( 'NONE',  ( 12.86946920628831670, 9.516571979449480523, -16.11446544321706398 ) ) ;
#11123=CARTESIAN_POINT ( 'NONE',  ( 12.50268541164654756, 8.571888915454989544, -15.12803469218787811 ) ) ;
#11128=CARTESIAN_POINT ( 'NONE',  ( 13.12425544150138279, 8.571136816377206813, -15.91139631635614471 ) ) ;
#11129=CARTESIAN_POINT ( 'NONE',  ( 24.91993355315554837, -1.627520125476753510, -17.55906114018776876 ) ) ;
#11130=CARTESIAN_POINT ( 'NONE',  ( 17.51795708650258732, -0.4494001013054305660, -15.13702969726144509 ) ) ;
#11131=CARTESIAN_POINT ( 'NONE',  ( 14.30110556002302680, 5.443193088601498530, -15.49285935407157666 ) ) ;
#11135=CARTESIAN_POINT ( 'NONE',  ( 19.71807001554888217, -1.708786246101231532, -19.21472004699903380 ) ) ;
#11140=CARTESIAN_POINT ( 'NONE',  ( 10.35864918915110877, 16.97212501191939538, -17.91752729848689185 ) ) ;
#11141=CARTESIAN_POINT ( 'NONE',  ( 32.48283477683061449, -11.02614750807341260, -17.91093295056291979 ) ) ;
#11147=CARTESIAN_POINT ( 'NONE',  ( 14.93287775521291394, 9.378568215907955974, -14.88591063491414168 ) ) ;
#11149=CARTESIAN_POINT ( 'NONE',  ( 12.24516467974477152, 9.516115653471018732, -15.33328326133307762 ) ) ;
#11150=CARTESIAN_POINT ( 'NONE',  ( 35.32886446602115171, -21.19738783794349857, -20.03221113960638178 ) ) ;
#11154=CARTESIAN_POINT ( 'NONE',  ( 12.75704675400704424, 7.626265983139092874, -14.92530421254393147 ) ) ;
#11159=CARTESIAN_POINT ( 'NONE',  ( 12.89562877257107054, 9.528132359803098694, -16.09361580714184825 ) ) ;
#11161=CARTESIAN_POINT ( 'NONE',  ( 34.49115424338278046, -12.94152926980570939, -19.96804914223585925 ) ) ;
#11162=CARTESIAN_POINT ( 'NONE',  ( 22.39939798857497877, 2.694615832958070722, -14.02792042734668065 ) ) ;
#11168=CARTESIAN_POINT ( 'NONE',  ( 22.68884594494833706, -6.762261587817247843, -18.56982216542981234 ) ) ;
#11169=CARTESIAN_POINT ( 'NONE',  ( 28.47173825316771101, -6.366402965996883268, -15.18523185298700007 ) ) ;
#11178=CARTESIAN_POINT ( 'NONE',  ( 12.50140887008201851, 8.571324787501421127, -15.12905211845398412 ) ) ;
#11180=CARTESIAN_POINT ( 'NONE',  ( 27.87518295380144551, -11.54787579004265652, -18.81772651352153858 ) ) ;
#11185=CARTESIAN_POINT ( 'NONE',  ( 30.94061990612449264, -11.12808277128230294, -15.28946652318938959 ) ) ;
#11188=CARTESIAN_POINT ( 'NONE',  ( 24.52797215547132836, -1.897736678990579184, -19.26084780660264073 ) ) ;
#11192=CARTESIAN_POINT ( 'NONE',  ( 12.24619727527933222, 9.516571979449480523, -15.33246026419563890 ) ) ;
#11193=CARTESIAN_POINT ( 'NONE',  ( 35.54859390953724585, -22.18451583373416014, -16.11276402859391865 ) ) ;
#11195=CARTESIAN_POINT ( 'NONE',  ( 22.16846437878366061, -4.107540447007581363, -19.06500358040360865 ) ) ;
#11197=CARTESIAN_POINT ( 'NONE',  ( 25.72346593501046996, -2.209713236584236018, -16.07608620281017053 ) ) ;
#11202=CARTESIAN_POINT ( 'NONE',  ( 17.83091951040035283, 10.74857467630938501, -15.40187535130914753 ) ) ;
#11203=CARTESIAN_POINT ( 'NONE',  ( 28.55476651072185845, -11.97999099613336504, -13.94805024529803994 ) ) ;
#11220=CARTESIAN_POINT ( 'NONE',  ( 23.84753192840887337, -5.516882280943989691, -18.03677479665242345 ) ) ;
#11221=CARTESIAN_POINT ( 'NONE',  ( 20.05507840940144959, 2.642024363331392234, -19.51255487852252912 ) ) ;
#11222=CARTESIAN_POINT ( 'NONE',  ( 34.47915806976548936, -13.88763681628941349, -21.00674453490027460 ) ) ;
#11226=CARTESIAN_POINT ( 'NONE',  ( 12.50098444160134470, 8.571137227758441668, -15.12939039523150520 ) ) ;
#11229=CARTESIAN_POINT ( 'NONE',  ( 9.667771292961528928, 16.22782245407549340, -17.88511957776909966 ) ) ;
#11232=CARTESIAN_POINT ( 'NONE',  ( 11.82447321682112751, 8.672047275158794477, -15.63808403058127006 ) ) ;
#11238=CARTESIAN_POINT ( 'NONE',  ( 9.112830967032516938, 16.17999385759334885, -17.05460035006107589 ) ) ;
#11239=CARTESIAN_POINT ( 'NONE',  ( 33.21739345078569272, -12.71166704379270129, -20.69560413545502797 ) ) ;
#11240=CARTESIAN_POINT ( 'NONE',  ( 18.68528716101036480, 3.575476808761081760, -13.14399490972872186 ) ) ;
#11242=CARTESIAN_POINT ( 'NONE',  ( 31.69910715399011636, -11.01187737159756352, -14.44698884073069145 ) ) ;
#11244=CARTESIAN_POINT ( 'NONE',  ( 18.48843674521961589, -1.244547778534776938, -16.48413177534300900 ) ) ;
#11256=CARTESIAN_POINT ( 'NONE',  ( 13.55939796120610374, 8.763434079353437767, -15.56458004748339263 ) ) ;
#11257=CARTESIAN_POINT ( 'NONE',  ( 35.54170021948790748, -21.15354613602950096, -18.58520066250327929 ) ) ;
#11260=CARTESIAN_POINT ( 'NONE',  ( 10.66464987567688993, 9.063154531648658363, -16.41286864359600983 ) ) ;
#11262=CARTESIAN_POINT ( 'NONE',  ( 26.32595758385100382, -12.12905223104374386, -14.21117607008287642 ) ) ;
#11264=CARTESIAN_POINT ( 'NONE',  ( 10.99070134719017311, 14.07345324724201063, -17.12031169937328201 ) ) ;
#11269=CARTESIAN_POINT ( 'NONE',  ( 12.50162201464318557, 8.571418981294288031, -15.12888223836978341 ) ) ;
#11274=CARTESIAN_POINT ( 'NONE',  ( 13.12174330432777047, 8.570030634161971861, -15.91339823077023929 ) ) ;
#11275=CARTESIAN_POINT ( 'NONE',  ( 24.98402180921622673, -1.135180495641346266, -16.01319527449767932 ) ) ;
#11276=CARTESIAN_POINT ( 'NONE',  ( 25.05533511103952904, -1.369129923259265524, -16.98221401193426416 ) ) ;
#11277=CARTESIAN_POINT ( 'NONE',  ( 19.14470263920462401, 1.819183656627200829, -19.33730474122706866 ) ) ;
#11282=CARTESIAN_POINT ( 'NONE',  ( 20.14386580841007657, 1.771853782379294140, -13.30505882909219295 ) ) ;
#11290=CARTESIAN_POINT ( 'NONE',  ( 10.35865266338826984, 16.97210907862488938, -17.91126819201198472 ) ) ;
#11295=CARTESIAN_POINT ( 'NONE',  ( 18.47369133221681281, 7.987600538477567014, -15.27093437040897861 ) ) ;
#11296=CARTESIAN_POINT ( 'NONE',  ( 11.43821061673542872, 15.93387534916056758, -16.71752457030684980 ) ) ;
#11297=CARTESIAN_POINT ( 'NONE',  ( 33.68411698100747032, -13.80840863474736935, -19.79436191385186916 ) ) ;
#11299=( BOUNDED_CURVE ( )  B_SPLINE_CURVE ( 3, ( #26588, #5672, #3385, #8397 ),
 .UNSPECIFIED., .F., .F. ) 
 B_SPLINE_CURVE_WITH_KNOTS ( ( 4, 4 ),
 ( 0.001563228649568139134, 0.003126104531729828346 ),
 .UNSPECIFIED. ) 
 CURVE ( )  GEOMETRIC_REPRESENTATION_ITEM ( )  RATIONAL_B_SPLINE_CURVE ( ( 1.000000000000001110, 0.3333333333333333703, 0.3333333333333322046, 1.000000000000000000 ) ) 
 REPRESENTATION_ITEM ( '' )  );
#11302=CARTESIAN_POINT ( 'NONE',  ( 9.641384570184822422, 17.66873631484086715, -17.89388817125738385 ) ) ;
#11308=CARTESIAN_POINT ( 'NONE',  ( 12.86946920628831670, 9.516571979449480523, -16.11446544321706398 ) ) ;
#11309=CARTESIAN_POINT ( 'NONE',  ( 35.06179249480944549, -15.50510465796065596, -20.14053939611612520 ) ) ;
#11310=CARTESIAN_POINT ( 'NONE',  ( 25.77659985377941254, -6.250509680199615836, -13.67467641272277312 ) ) ;
#11313=CARTESIAN_POINT ( 'NONE',  ( 28.50411217586706769, -6.135108760518566129, -18.55796808427148648 ) ) ;
#11314=CARTESIAN_POINT ( 'NONE',  ( 28.03106068525412908, -6.431813172927290267, -14.41205174211060402 ) ) ;
#11326=CARTESIAN_POINT ( 'NONE',  ( 12.49428694376680049, 8.568214790255201052, -15.13472557389765072 ) ) ;
#11327=CARTESIAN_POINT ( 'NONE',  ( 31.69910715399011636, -11.01187737159756352, -14.44698884073069145 ) ) ;
#11331=CARTESIAN_POINT ( 'NONE',  ( 9.641350810849047548, 17.66889113945805789, -17.92981046679734547 ) ) ;
#11333=CARTESIAN_POINT ( 'NONE',  ( 15.19333023161420648, 6.044621996704095501, -18.15278115226310263 ) ) ;
#11336=CARTESIAN_POINT ( 'NONE',  ( 24.18219217278060995, -6.970120066757704791, -14.18070892486464629 ) ) ;
#11340=CARTESIAN_POINT ( 'NONE',  ( 12.24537663854593816, 9.516207477791880365, -15.33311446707169701 ) ) ;
#11343=CARTESIAN_POINT ( 'NONE',  ( 33.57712230886461668, -13.32773824946660923, -19.76201999124979736 ) ) ;
#11344=CARTESIAN_POINT ( 'NONE',  ( 15.19603151210977821, 9.502094893032342782, -14.87270315361914896 ) ) ;
#11345=CARTESIAN_POINT ( 'NONE',  ( 26.31132954256896639, -3.159408024760113509, -14.81636702655834803 ) ) ;
#11347=CARTESIAN_POINT ( 'NONE',  ( 20.39818463913025681, -2.063888138892570723, -16.18016139629216354 ) ) ;
#11350=CARTESIAN_POINT ( 'NONE',  ( 17.10097030076851610, 6.697663726599960121, -13.82760435466811089 ) ) ;
#11352=CARTESIAN_POINT ( 'NONE',  ( 28.61171173311277016, -11.12923776720465874, -18.00325214586577971 ) ) ;
#11362=CARTESIAN_POINT ( 'NONE',  ( 23.18557557936948044, -8.345241077663208884, -16.42592668061853800 ) ) ;
#11363=CARTESIAN_POINT ( 'NONE',  ( 18.53947781130984751, 1.256531364521723537, -18.82393729036428098 ) ) ;
#11365=CARTESIAN_POINT ( 'NONE',  ( 34.13391181137448882, -12.33661648534566524, -20.90239171999057888 ) ) ;
#11368=CARTESIAN_POINT ( 'NONE',  ( 11.47293561586387867, 9.269010148984008879, -15.86088772249501666 ) ) ;
#11371=CARTESIAN_POINT ( 'NONE',  ( 9.662070302079424522, 16.25396792496884046, -17.90822120357413638 ) ) ;
#11375=CARTESIAN_POINT ( 'NONE',  ( 12.50098444160134470, 8.571137227758441668, -15.12939039523150520 ) ) ;
#11379=DIRECTION ( 'NONE',  ( -1.000000000000000000, 0.000000000000000000, -0.000000000000000000 ) ) ;
#11383=CARTESIAN_POINT ( 'NONE',  ( 9.132840175088396961, 16.08822907886823472, -17.04632583937691592 ) ) ;
#11384=CARTESIAN_POINT ( 'NONE',  ( 31.39893620166130717, -10.86152586746012183, -14.84747879817187943 ) ) ;
#11385=CARTESIAN_POINT ( 'NONE',  ( 15.52843720209238931, 6.760224976758691717, -13.32525641785786696 ) ) ;
#11386=CARTESIAN_POINT ( 'NONE',  ( 18.45234147263269620, 6.489596213788811241, -14.85506563039705519 ) ) ;
#11388=CARTESIAN_POINT ( 'NONE',  ( 23.77355757633466382, -7.879698323813751237, -13.16654918938113283 ) ) ;
#11396=CARTESIAN_POINT ( 'NONE',  ( 35.39068211221506743, -20.47510177656754493, -19.23609803736608725 ) ) ;
#11397=CARTESIAN_POINT ( 'NONE',  ( 11.11829553246053770, 8.091015213210848600, -16.14073874907621331 ) ) ;
#11399=CARTESIAN_POINT ( 'NONE',  ( 27.78884322698630882, -6.380937659459246625, -17.89340433249687834 ) ) ;
#11401=CARTESIAN_POINT ( 'NONE',  ( 10.50441255335269020, 16.30363564318377811, -17.32140922184415288 ) ) ;
#11410=CARTESIAN_POINT ( 'NONE',  ( 14.38576730248667701, 9.404056492746565965, -13.62718518646353161 ) ) ;
#11415=CARTESIAN_POINT ( 'NONE',  ( 9.664154528927689114, 16.24440939496457403, -17.89215119606715021 ) ) ;
#11416=CARTESIAN_POINT ( 'NONE',  ( 21.88384027766407414, -2.187040905716116868, -14.00385029740408704 ) ) ;
#11417=CARTESIAN_POINT ( 'NONE',  ( 24.36273546358933828, 1.710929640254579720, -17.54733717687237160 ) ) ;
#11418=CARTESIAN_POINT ( 'NONE',  ( 21.26575470983302196, 3.903880982571942493, -18.68858533207590966 ) ) ;
#11422=CARTESIAN_POINT ( 'NONE',  ( 22.29983652437130814, 0.6627547066652448304, -20.09853802436992964 ) ) ;
#11427=CARTESIAN_POINT ( 'NONE',  ( 10.35865057885519214, 16.97211863855931924, -17.91295731025335414 ) ) ;
#11428=CARTESIAN_POINT ( 'NONE',  ( 35.54859390953724585, -22.18451583373416014, -16.11276402859391865 ) ) ;
#11434=CARTESIAN_POINT ( 'NONE',  ( 13.77718166750866224, 8.859676595473322536, -15.39100258941132715 ) ) ;
#11435=CARTESIAN_POINT ( 'NONE',  ( 11.05584814685795081, 17.68743837589741830, -17.84564518929906285 ) ) ;
#11436=CARTESIAN_POINT ( 'NONE',  ( 33.43446274600908907, -12.68684440242773448, -19.71889742777951327 ) ) ;
#11439=CARTESIAN_POINT ( 'NONE',  ( 9.916118674515717046, 16.40877069192658055, -16.50468880802031890 ) ) ;
#11441=CARTESIAN_POINT ( 'NONE',  ( 9.641350810849047548, 17.66889113945805789, -17.92279151347709032 ) ) ;
#11449=CARTESIAN_POINT ( 'NONE',  ( 10.46960557229346733, 16.46326489517938541, -17.33590790293451178 ) ) ;
#11450=CARTESIAN_POINT ( 'NONE',  ( 34.06228043176686526, -11.34293828116054037, -19.64761387034043949 ) ) ;
#11451=CARTESIAN_POINT ( 'NONE',  ( 24.95482030053459965, -6.624749414579512496, -13.76522253407564733 ) ) ;
#11454=CARTESIAN_POINT ( 'NONE',  ( 16.51457045034215199, 5.649390745141357861, -14.67502403374339437 ) ) ;
#11455=CARTESIAN_POINT ( 'NONE',  ( 23.58034929565730309, -2.629172400889816075, -20.70693660786654888 ) ) ;
#11464=CARTESIAN_POINT ( 'NONE',  ( 10.33812163068573575, 18.38616799828327686, -17.90626694547636433 ) ) ;
#11469=CARTESIAN_POINT ( 'NONE',  ( 11.46877092736959014, 9.288109543210406827, -15.86260999805022820 ) ) ;
#11473=CARTESIAN_POINT ( 'NONE',  ( 27.66237087416717699, -12.37519551434573017, -14.68082181149132204 ) ) ;
#11477=CARTESIAN_POINT ( 'NONE',  ( 28.12266609392075267, -5.599633216697744942, -16.00068813756295327 ) ) ;
#11482=CARTESIAN_POINT ( 'NONE',  ( 12.51736351114195500, 9.636405190433555035, -15.11633598780129439 ) ) ;
#11484=CARTESIAN_POINT ( 'NONE',  ( 33.68411698100747032, -13.80840863474736935, -19.79436191385186916 ) ) ;
#11487=CARTESIAN_POINT ( 'NONE',  ( 21.08246358516588259, -1.232126404925322438, -18.58940169363586037 ) ) ;
#11492=CARTESIAN_POINT ( 'NONE',  ( 21.37428249720081297, 2.009508332918806151, -14.44682725892062614 ) ) ;
#11493=CARTESIAN_POINT ( 'NONE',  ( 26.51887141003594195, -6.641914482010843557, -12.47546034222045819 ) ) ;
#11503=CARTESIAN_POINT ( 'NONE',  ( 9.641350810849047548, 17.66889113945805789, -17.92015940598198753 ) ) ;
#11504=CARTESIAN_POINT ( 'NONE',  ( 21.56333733550986409, -5.354713294276967517, -13.65854400988971484 ) ) ;
#11505=CARTESIAN_POINT ( 'NONE',  ( 20.07445496384854877, 6.874260549971754841, -18.87959640166664954 ) ) ;
#11506=CARTESIAN_POINT ( 'NONE',  ( 34.52807818452484412, -18.59987926346575549, -21.09179268733712576 ) ) ;
#11508=CARTESIAN_POINT ( 'NONE',  ( 12.47535353872619446, 8.560407331872438519, -15.14977315560688176 ) ) ;
#11513=CARTESIAN_POINT ( 'NONE',  ( 14.93287775521291394, 9.378568215907955974, -14.88591063491414168 ) ) ;
#11517=CARTESIAN_POINT ( 'NONE',  ( 10.33811693838771717, 18.38618951776012267, -21.33333333332589632 ) ) ;
#11523=CARTESIAN_POINT ( 'NONE',  ( 18.21616227284554057, 4.699354889203569918, -13.86658597208997179 ) ) ;
#11526=CARTESIAN_POINT ( 'NONE',  ( 9.274674406624409784, 15.43775921338471413, -16.98767239532306661 ) ) ;
#11527=CARTESIAN_POINT ( 'NONE',  ( 32.52689891806821265, -10.77327725507678302, -19.81022979934233064 ) ) ;
#11528=CARTESIAN_POINT ( 'NONE',  ( 17.45108151888110726, 3.014897074772306507, -13.47014999590450479 ) ) ;
#11529=CARTESIAN_POINT ( 'NONE',  ( 13.40933447586352578, 7.914523597318124715, -14.40541938456405369 ) ) ;
#11531=CARTESIAN_POINT ( 'NONE',  ( 20.11894618883271946, -4.454955732405634805, -18.36807076737963129 ) ) ;
#11541=CARTESIAN_POINT ( 'NONE',  ( 32.11202735699620803, -10.19471129157119194, -14.63100864886716934 ) ) ;
#11542=CARTESIAN_POINT ( 'NONE',  ( 10.66915452275446619, 9.042499785519874322, -16.41100549784887619 ) ) ;
#11546=CARTESIAN_POINT ( 'NONE',  ( 10.35873811938078504, 16.97171716655003593, -17.89325570535168453 ) ) ;
#11557=CARTESIAN_POINT ( 'NONE',  ( 9.797549260427590667, 15.63264415243319938, -17.83144836289601898 ) ) ;
#11559=CARTESIAN_POINT ( 'NONE',  ( 21.05341046998850629, -2.558799731849103587, -14.42238450910079806 ) ) ;
#11560=CARTESIAN_POINT ( 'NONE',  ( 22.79055345825320344, -4.301464833599455417, -14.90020420563294046 ) ) ;
#11562=CARTESIAN_POINT ( 'NONE',  ( 19.75232399841803854, 1.290101960903724754, -14.36573431580270999 ) ) ;
#11566=CARTESIAN_POINT ( 'NONE',  ( 26.72610680620850232, -7.491537437428757329, -18.63066883040512067 ) ) ;
#11577=CARTESIAN_POINT ( 'NONE',  ( 10.35864919943752405, 16.97212496474457311, -17.91550491156534974 ) ) ;
#11582=CARTESIAN_POINT ( 'NONE',  ( 11.22367979475099631, 9.092227732665495665, -17.24169321984975056 ) ) ;
#11585=CARTESIAN_POINT ( 'NONE',  ( 21.42923412144385509, -1.598955984811285536, -13.33006947543598741 ) ) ;
#11586=CARTESIAN_POINT ( 'NONE',  ( 11.27674754065650653, 16.67436559781366157, -16.78429523206404994 ) ) ;
#11587=CARTESIAN_POINT ( 'NONE',  ( 35.09336438560361415, -20.13941072448723801, -20.22035334018532637 ) ) ;
#11591=CARTESIAN_POINT ( 'NONE',  ( 9.917015787971365626, 16.40465641526357743, -16.50431533440121257 ) ) ;
#11593=CARTESIAN_POINT ( 'NONE',  ( 9.641350810849047548, 17.66889113945805789, -17.91928203681695564 ) ) ;
#11599=CARTESIAN_POINT ( 'NONE',  ( 10.47230989469697882, 16.45086252791593751, -17.33468480047602256 ) ) ;
#11600=CARTESIAN_POINT ( 'NONE',  ( 34.16709027601721971, -12.48568152589075098, -20.91241392730897886 ) ) ;
#11601=CARTESIAN_POINT ( 'NONE',  ( 24.60501232743784783, -9.531698448777172317, -16.22453333552994792 ) ) ;
#11607=CARTESIAN_POINT ( 'NONE',  ( 19.47111902912460124, 6.782054727477878409, -15.90798308235397407 ) ) ;
#11609=CARTESIAN_POINT ( 'NONE',  ( 27.54771222089439320, -11.35863810494041459, -14.08592588049474692 ) ) ;
#11623=CARTESIAN_POINT ( 'NONE',  ( 10.72074420406304895, 16.63141210374104872, -15.95421917676928025 ) ) ;
#11628=CARTESIAN_POINT ( 'NONE',  ( 10.82443827553465177, 12.24310121783546634, -16.12906421532448675 ) ) ;
#11629=CARTESIAN_POINT ( 'NONE',  ( 17.11242430243909141, 7.828829022555451544, -19.39938683153768295 ) ) ;
#11632=CARTESIAN_POINT ( 'NONE',  ( 28.06689949639850212, -8.111051215268487269, -13.49421662364394514 ) ) ;
#11637=CARTESIAN_POINT ( 'NONE',  ( 11.27564905058850719, 16.67940341329043363, -16.78475148866115774 ) ) ;
#11640=CARTESIAN_POINT ( 'NONE',  ( 35.49237112349044310, -21.93193663806729887, -19.32748734164077931 ) ) ;
#11643=CARTESIAN_POINT ( 'NONE',  ( 31.14759003376246582, -7.259970019232452998, -15.53234487094253069 ) ) ;
#11646=CARTESIAN_POINT ( 'NONE',  ( 16.63724033897865340, 2.930722838386041751, -15.17604395537502526 ) ) ;
#11647=CARTESIAN_POINT ( 'NONE',  ( 27.40270966038060152, -12.25096941946872953, -16.90735844088681006 ) ) ;
#11660=CARTESIAN_POINT ( 'NONE',  ( 9.916551108984865692, 16.40678749232849398, -16.50450761325770443 ) ) ;
#11661=CARTESIAN_POINT ( 'NONE',  ( 24.41106252871404436, -7.915231898853421377, -13.94454578273958667 ) ) ;
#11662=CARTESIAN_POINT ( 'NONE',  ( 22.45293885382703536, -0.3771200753331621081, -14.01028023225368635 ) ) ;
#11663=CARTESIAN_POINT ( 'NONE',  ( 36.54859390954302967, -23.18451583373416014, -15.55638201429745848 ) ) ;
#11669=CARTESIAN_POINT ( 'NONE',  ( 17.95327243003904982, 7.812726124483462264, -14.88485059575767266 ) ) ;
#11672=CARTESIAN_POINT ( 'NONE',  ( 10.73702987185851931, 16.55672395529124330, -15.94748436097269817 ) ) ;
#11676=CARTESIAN_POINT ( 'NONE',  ( 15.70491959545049987, 3.570626008024105680, -15.63470537622339229 ) ) ;
#11679=CARTESIAN_POINT ( 'NONE',  ( 25.18430082464795916, -12.47910854170484818, -17.34997305645471855 ) ) ;
#11682=CARTESIAN_POINT ( 'NONE',  ( 33.74345058881453241, -15.07496310474945922, -20.85461858825047798 ) ) ;
#11683=CARTESIAN_POINT ( 'NONE',  ( 22.42041779846375604, -0.009017426515379003624, -18.82878497401882001 ) ) ;
#11684=CARTESIAN_POINT ( 'NONE',  ( 16.51457045034215199, 5.649390745141357861, -14.67502403374339437 ) ) ;
#11685=CARTESIAN_POINT ( 'NONE',  ( 30.29779709953443501, -9.168887887504279632, -16.05354238668875055 ) ) ;
#11699=CARTESIAN_POINT ( 'NONE',  ( 36.19723272591463115, -19.60603615691276858, -19.44143419077989421 ) ) ;
#11700=CARTESIAN_POINT ( 'NONE',  ( 12.82404076521984670, 7.655871835264917102, -14.87190880308183871 ) ) ;
#11704=CARTESIAN_POINT ( 'NONE',  ( 10.41412541532089620, 16.71770396712979689, -17.42473314453425814 ) ) ;
#11714=CARTESIAN_POINT ( 'NONE',  ( 9.667864356596815867, 16.22739565238121529, -17.88507765419223716 ) ) ;
#11717=CARTESIAN_POINT ( 'NONE',  ( 23.17017814088865535, -4.132587038751921682, -14.65442522582375240 ) ) ;
#11718=CARTESIAN_POINT ( 'NONE',  ( 24.81022290780906658, -1.767900772465358372, -17.79475844156381470 ) ) ;
#11719=CARTESIAN_POINT ( 'NONE',  ( 21.10828700581006601, 3.717818950362942854, -18.90958453460783417 ) ) ;
#11723=CARTESIAN_POINT ( 'NONE',  ( 27.95388715220626707, -5.541385876428546631, -15.41148221666858831 ) ) ;
#11732=CARTESIAN_POINT ( 'NONE',  ( 10.38089682401341385, 16.87009452252716102, -17.57504515238516873 ) ) ;
#11733=CARTESIAN_POINT ( 'NONE',  ( 35.54859390953724585, -22.18451583373416014, -18.06010107863414405 ) ) ;
#11735=CARTESIAN_POINT ( 'NONE',  ( 32.89062095351589932, -11.25267498498577723, -18.96775996542842435 ) ) ;
#11737=CARTESIAN_POINT ( 'NONE',  ( 8.944584694422324844, 16.95159271019519664, -17.91554756312530117 ) ) ;
#11740=CARTESIAN_POINT ( 'NONE',  ( 23.36212950203212557, 2.915605996956767587, -15.34809340432955693 ) ) ;
#11741=CARTESIAN_POINT ( 'NONE',  ( 11.20364811077027767, 17.00960890128215297, -16.86645280501126365 ) ) ;
#11746=CARTESIAN_POINT ( 'NONE',  ( 9.917965570771830386, 16.40030059027150600, -16.50392256580263606 ) ) ;
#11748=CARTESIAN_POINT ( 'NONE',  ( 9.957223259857686415, 16.22025982393231303, -16.48768813039480818 ) ) ;
#11754=CARTESIAN_POINT ( 'NONE',  ( 10.53683180627515981, 16.15495681678771689, -17.30800272034635867 ) ) ;
#11757=CARTESIAN_POINT ( 'NONE',  ( 32.09732368354767118, -9.542663571685382706, -16.59113971387166941 ) ) ;
#11759=CARTESIAN_POINT ( 'NONE',  ( 25.97256211245905533, -8.171536508395311316, -18.54953510021574559 ) ) ;
#11762=CARTESIAN_POINT ( 'NONE',  ( 33.28625081342995884, -10.37305140221732991, -17.94975064729133862 ) ) ;
#11764=ORIENTED_EDGE ( 'NONE', *, *, #18000, .F. ) ;
#11765=CARTESIAN_POINT ( 'NONE',  ( 27.62103240953636174, -12.62788667074165794, -13.46147607715242245 ) ) ;
#11766=CARTESIAN_POINT ( 'NONE',  ( 29.25528888857379783, -9.059906918047152757, -17.02304095575280130 ) ) ;
#11773=CARTESIAN_POINT ( 'NONE',  ( 10.35008142444812052, 18.33131885956999696, -17.43324812465761653 ) ) ;
#11777=CARTESIAN_POINT ( 'NONE',  ( 9.936961226781097167, 16.31318409042999917, -16.49606719383117337 ) ) ;
#11780=CARTESIAN_POINT ( 'NONE',  ( 16.16754939756797782, 8.873905313537072459, -14.69432754670026142 ) ) ;
#11784=CARTESIAN_POINT ( 'NONE',  ( 26.92971693216691165, -8.617903733377630715, -13.36642543767191427 ) ) ;
#11787=CARTESIAN_POINT ( 'NONE',  ( 11.27553273857261296, 16.67993683502164615, -16.78480078315762469 ) ) ;
#11790=CARTESIAN_POINT ( 'NONE',  ( 33.30991885831043220, -11.83535627117299960, -18.22721479198959926 ) ) ;
#11791=CARTESIAN_POINT ( 'NONE',  ( 16.53342136567307108, 10.04554801986687629, -15.32032680638607047 ) ) ;
#11796=CARTESIAN_POINT ( 'NONE',  ( 27.35338705259445646, -4.307586880325415812, -13.99634582963401996 ) ) ;
#11799=CARTESIAN_POINT ( 'NONE',  ( 18.97628335640213493, 0.9430780577607489334, -14.77698032187241850 ) ) ;
#11800=CARTESIAN_POINT ( 'NONE',  ( 15.31194320040279777, 8.488938064892046498, -14.62880434596509183 ) ) ;
#11811=CARTESIAN_POINT ( 'NONE',  ( 9.917965570771830386, 16.40030059027150600, -16.50392256580263606 ) ) ;
#11812=CARTESIAN_POINT ( 'NONE',  ( 25.61803826562323394, -0.4625480611756047078, -19.10237625710802334 ) ) ;
#11813=CARTESIAN_POINT ( 'NONE',  ( 22.84118038848623655, 1.850029439873439152, -18.07216660426987431 ) ) ;
#11815=CARTESIAN_POINT ( 'NONE',  ( 31.95629010954621663, -10.29636179124881679, -18.42443288805318247 ) ) ;
#11821=CARTESIAN_POINT ( 'NONE',  ( 17.66155849027303049, 7.702290371990539342, -14.74052880078125760 ) ) ;
#11824=CARTESIAN_POINT ( 'NONE',  ( 10.52543090623380451, 17.52714378424053265, -16.25779133722369707 ) ) ;
#11829=CARTESIAN_POINT ( 'NONE',  ( 21.64656857049893901, 5.639188926465734220, -17.17864421186117951 ) ) ;
#11832=CARTESIAN_POINT ( 'NONE',  ( 29.95565488329840775, -10.73317148848732039, -11.80569981112315325 ) ) ;
#11835=CARTESIAN_POINT ( 'NONE',  ( 35.53993026725221682, -23.14559467820676275, -18.82474504553469075 ) ) ;
#11836=CARTESIAN_POINT ( 'NONE',  ( 22.40466763571637543, -1.191653471825661059, -14.65485681160645548 ) ) ;
#11837=CARTESIAN_POINT ( 'NONE',  ( 17.95893182911733277, 3.791778598950861667, -15.25628287466289024 ) ) ;
#11839=CARTESIAN_POINT ( 'NONE',  ( 26.13670795350922660, -6.813068953109826076, -12.41955265015470999 ) ) ;
#11847=CARTESIAN_POINT ( 'NONE',  ( 36.54816482920796972, -21.18258820310476409, -18.41547799146826847 ) ) ;
#11848=CARTESIAN_POINT ( 'NONE',  ( 12.79001206111077948, 7.640833942120977440, -14.89903028090515136 ) ) ;
#11853=CARTESIAN_POINT ( 'NONE',  ( 10.47139596700049147, 16.45505391683073526, -17.33506929010674114 ) ) ;
#11865=CARTESIAN_POINT ( 'NONE',  ( 9.667069921042207525, 16.23103903510144619, -17.88562738470040969 ) ) ;
#11866=CARTESIAN_POINT ( 'NONE',  ( 25.35799213500633442, -5.391047399292974163, -13.97031313328441726 ) ) ;
#11867=CARTESIAN_POINT ( 'NONE',  ( 20.97044927184332508, -4.289323992320570156, -15.06659861376252429 ) ) ;
#11871=CARTESIAN_POINT ( 'NONE',  ( 21.43917814492346707, -4.799604530101110988, -17.97822123721208243 ) ) ;
#11878=CARTESIAN_POINT ( 'NONE',  ( 10.60167031212029443, 15.85759916399494607, -17.28118971735050735 ) ) ;
#11881=CARTESIAN_POINT ( 'NONE',  ( 33.96943610671532809, -15.09019632882451134, -19.88060704079178720 ) ) ;
#11883=CARTESIAN_POINT ( 'NONE',  ( 13.38265815842314943, 7.627299838292535661, -15.70544478996546900 ) ) ;
#11886=CARTESIAN_POINT ( 'NONE',  ( 22.39939798857497877, 2.694615832958070722, -14.02792042734668065 ) ) ;
#11887=CARTESIAN_POINT ( 'NONE',  ( 11.27624053946810889, 16.67669076989127674, -16.78450489582619554 ) ) ;
#11890=CARTESIAN_POINT ( 'NONE',  ( 9.641359250860388030, 17.66885243249017634, -17.90483003768722625 ) ) ;
#11893=CARTESIAN_POINT ( 'NONE',  ( 9.905109554012803130, 16.45925992188944420, -16.51025697316969953 ) ) ;
#11900=CARTESIAN_POINT ( 'NONE',  ( 10.47139596700049147, 16.45505391683073526, -17.33506929010674114 ) ) ;
#11902=CARTESIAN_POINT ( 'NONE',  ( 32.39840662109286029, -9.588391805189495187, -17.44209920064860597 ) ) ;
#11903=CARTESIAN_POINT ( 'NONE',  ( 16.30094628073386076, 10.97451324635404291, -15.74372407192620216 ) ) ;
#11904=CARTESIAN_POINT ( 'NONE',  ( 27.44219139316946965, -6.774709612358828181, -18.29578255718776703 ) ) ;
#11908=CARTESIAN_POINT ( 'NONE',  ( 15.13914318552241056, 5.040073780016904870, -15.86576734333453764 ) ) ;
#11909=CARTESIAN_POINT ( 'NONE',  ( 25.65469514739125856, -9.762610920096198797, -17.09127189072687614 ) ) ;
#11917=PRODUCT_DEFINITION ( 'UNKNOWN', '', #21444, #24752 ) ;
#11920=CARTESIAN_POINT ( 'NONE',  ( 10.65690970294255280, 16.92416526288626955, -16.00322527524160066 ) ) ;
#11924=CARTESIAN_POINT ( 'NONE',  ( 11.47293561586387867, 9.269010148984008879, -15.86088772249501666 ) ) ;
#11925=CARTESIAN_POINT ( 'NONE',  ( 9.666872068725954392, 16.23194641104447911, -17.88584179299332533 ) ) ;
#11926=CARTESIAN_POINT ( 'NONE',  ( 17.50199379865806293, 2.211901401554522639, -18.92990045904890550 ) ) ;
#11929=CARTESIAN_POINT ( 'NONE',  ( 28.67486520862709654, -7.888541471525570614, -13.83454100519475105 ) ) ;
#11932=CARTESIAN_POINT ( 'NONE',  ( 11.23925813788225447, 16.84629677772421275, -16.81283633444384407 ) ) ;
#11934=CARTESIAN_POINT ( 'NONE',  ( 35.54859390953724585, -21.18451583373416014, -17.78191007148576119 ) ) ;
#11935=FACE_OUTER_BOUND ( 'NONE', #25106, .T. ) ;
#11940=CARTESIAN_POINT ( 'NONE',  ( 24.62608015258945215, -5.401662417846991637, -13.04198456947205820 ) ) ;
#11943=CARTESIAN_POINT ( 'NONE',  ( 19.36978511310259421, 2.022953856625822944, -19.43459320487130171 ) ) ;
#11944=CARTESIAN_POINT ( 'NONE',  ( 18.67591552545227174, 7.243412299697878254, -16.30691131850022657 ) ) ;
#11959=CARTESIAN_POINT ( 'NONE',  ( 9.776119957569173735, 17.05082265352876547, -16.72288386497739765 ) ) ;
#11960=CARTESIAN_POINT ( 'NONE',  ( 23.87837110222071502, -4.315358902625421322, -12.52832693522684693 ) ) ;
#11961=CARTESIAN_POINT ( 'NONE',  ( 24.68325608809179528, -0.07379305852225118145, -17.41420097001153167 ) ) ;
#11962=CARTESIAN_POINT ( 'NONE',  ( 36.54742519285235858, -23.17926540875556896, -18.54852884019370762 ) ) ;
#11967=CARTESIAN_POINT ( 'NONE',  ( 15.19603151210977821, 9.502094893032342782, -14.87270315361914896 ) ) ;
#11970=CARTESIAN_POINT ( 'NONE',  ( 10.71880336532874445, 16.64031303757595026, -15.95504377300109944 ) ) ;
#11976=CARTESIAN_POINT ( 'NONE',  ( 21.58242789233717573, 5.264303332692052528, -18.32037006577847293 ) ) ;
#11978=CARTESIAN_POINT ( 'NONE',  ( 32.00807787192805876, -10.01600718589171990, -13.21854031764240389 ) ) ;
#11980=CARTESIAN_POINT ( 'NONE',  ( 33.35202879388211983, -12.33251541790028760, -19.68467382345759376 ) ) ;
#11981=CARTESIAN_POINT ( 'NONE',  ( 20.36893440901172170, -1.919154233093003814, -17.42624063329192552 ) ) ;
#11983=CARTESIAN_POINT ( 'NONE',  ( 17.24163842130223046, 3.474294283696999219, -15.80253352452890425 ) ) ;
#11985=CARTESIAN_POINT ( 'NONE',  ( 29.20193236150002392, -6.731655735042891386, -17.98962132073140552 ) ) ;
#11997=CARTESIAN_POINT ( 'NONE',  ( 34.93112910557051976, -13.91810326443952306, -19.05872143998290014 ) ) ;
#11999=CARTESIAN_POINT ( 'NONE',  ( 9.641350810849047548, 17.66889113945805789, -17.92279151347709032 ) ) ;
#12005=CARTESIAN_POINT ( 'NONE',  ( 13.09018272752966716, 8.557097568986355540, -15.93847522207377310 ) ) ;
#12015=CARTESIAN_POINT ( 'NONE',  ( 9.700291501659986437, 16.07868063162199945, -17.87166786738998780 ) ) ;
#12016=CARTESIAN_POINT ( 'NONE',  ( 27.00779440489029071, -4.779404007149373079, -14.88408750732950914 ) ) ;
#12017=CARTESIAN_POINT ( 'NONE',  ( 20.59283418570449697, -4.290598171560842111, -16.90930062131523215 ) ) ;
#12023=CARTESIAN_POINT ( 'NONE',  ( 25.04068920418659161, -5.475481712173364990, -18.92835678451453774 ) ) ;
#12036=CARTESIAN_POINT ( 'NONE',  ( 11.50940939395034768, 11.69459202490242689, -16.90580767540677343 ) ) ;
#12038=CARTESIAN_POINT ( 'NONE',  ( 33.37634376253905089, -12.42895282922877342, -19.69946502924221932 ) ) ;
#12040=CARTESIAN_POINT ( 'NONE',  ( 13.43370121458407418, 7.649856678006609734, -15.66476257323406784 ) ) ;
#12044=CARTESIAN_POINT ( 'NONE',  ( 19.71807001554888217, -1.708786246101231532, -19.21472004699903380 ) ) ;
#12045=CARTESIAN_POINT ( 'NONE',  ( 12.83198842527593087, 9.541832653742346793, -16.14114841745374562 ) ) ;
#12049=CARTESIAN_POINT ( 'NONE',  ( 9.913797604922770290, 16.41941541294738727, -16.50570979788118464 ) ) ;
#12051=CARTESIAN_POINT ( 'NONE',  ( 9.916551108984865692, 16.40678749232849398, -16.50450761325770443 ) ) ;
#12053=ORIENTED_EDGE ( 'NONE', *, *, #3821, .T. ) ;
#12056=CARTESIAN_POINT ( 'NONE',  ( 10.35870477237433818, 16.97187010017241349, -17.89775757279876700 ) ) ;
#12058=CARTESIAN_POINT ( 'NONE',  ( 33.01522398464379648, -9.800858501837518943, -19.11635465682842394 ) ) ;
#12059=CARTESIAN_POINT ( 'NONE',  ( 29.76939623719675510, -8.219725197086590995, -17.35520659559267287 ) ) ;
#12060=CARTESIAN_POINT ( 'NONE',  ( 15.44177808481316383, 7.494736869644298416, -14.00399691429678306 ) ) ;
#12065=CARTESIAN_POINT ( 'NONE',  ( 27.03191753302054323, -12.88672130028117735, -14.08881772908025454 ) ) ;
#12066=CARTESIAN_POINT ( 'NONE',  ( 28.63694740700460173, -9.765300015774602826, -17.75617681614052046 ) ) ;
#12076=CARTESIAN_POINT ( 'NONE',  ( 36.04859390953723874, -22.18451583373416014, -15.00000000000000000 ) ) ;
#12079=CARTESIAN_POINT ( 'NONE',  ( 10.72107673987424015, 16.62988705212242735, -15.95408154060974404 ) ) ;
#12083=CARTESIAN_POINT ( 'NONE',  ( 10.17605321708455257, 15.21667774575863419, -16.39719424528293246 ) ) ;
#12086=CARTESIAN_POINT ( 'NONE',  ( 21.72387110042699376, 1.401658020055618792, -20.45241765577301152 ) ) ;
#12090=CARTESIAN_POINT ( 'NONE',  ( 30.24922550192677306, -10.40856591028444278, -13.02298783260255988 ) ) ;
#12093=CARTESIAN_POINT ( 'NONE',  ( 11.27588265011317326, 16.67833209609329259, -16.78465339804365541 ) ) ;
#12096=CARTESIAN_POINT ( 'NONE',  ( 34.98004922032874475, -18.63034571161586683, -19.14376959241974774 ) ) ;
#12097=CARTESIAN_POINT ( 'NONE',  ( 14.24706144987486667, 6.238427219560604087, -16.72753349211556184 ) ) ;
#12099=CARTESIAN_POINT ( 'NONE',  ( 8.977559110355956662, 16.80036783546273327, -17.41076197725142194 ) ) ;
#12100=CARTESIAN_POINT ( 'NONE',  ( 22.80194228990702143, -6.214338098008789224, -14.16187805771452801 ) ) ;
#12106=CARTESIAN_POINT ( 'NONE',  ( 21.65198393244800812, 4.573788442230395823, -17.29480057625502454 ) ) ;
#12107=CARTESIAN_POINT ( 'NONE',  ( 17.00905032053054811, 4.985101812230166907, -18.82491780458422781 ) ) ;
#12118=CARTESIAN_POINT ( 'NONE',  ( 9.641350829061996919, 17.66889105593114806, -17.91548090047172437 ) ) ;
#12120=CARTESIAN_POINT ( 'NONE',  ( 26.19520757255249066, -7.109971961106261951, -13.37903969216112898 ) ) ;
#12121=CARTESIAN_POINT ( 'NONE',  ( 21.56383972367567736, -3.323709001909281202, -18.92284382192250192 ) ) ;
#12122=CARTESIAN_POINT ( 'NONE',  ( 34.79556486487921774, -19.80155522666461465, -21.17264749384332134 ) ) ;
#12126=CARTESIAN_POINT ( 'NONE',  ( 14.38576730248667701, 9.404056492746565965, -13.62718518646353161 ) ) ;
#12129=CARTESIAN_POINT ( 'NONE',  ( 15.93484470893836935, 6.939319753835953009, -14.67888072223970752 ) ) ;
#12132=CARTESIAN_POINT ( 'NONE',  ( 10.70792791965113544, 16.69018921775036546, -15.96040338026158523 ) ) ;
#12136=CARTESIAN_POINT ( 'NONE',  ( 14.39533340154967433, 6.572929804808670617, -18.54476805420031837 ) ) ;
#12137=CARTESIAN_POINT ( 'NONE',  ( 26.67611703245768950, -12.21101477627283849, -12.48819288018415108 ) ) ;
#12139=CARTESIAN_POINT ( 'NONE',  ( 32.74314609665832165, -11.10724048739539782, -18.62249297335446840 ) ) ;
#12142=CARTESIAN_POINT ( 'NONE',  ( 22.92155253933561809, -3.178009374129639131, -14.34666800710537693 ) ) ;
#12145=CARTESIAN_POINT ( 'NONE',  ( 22.41093758190154972, 3.143874582428516806, -16.84310506638757943 ) ) ;
#12147=CARTESIAN_POINT ( 'NONE',  ( 25.09247252535503492, -10.89683230441130135, -15.98339435310939827 ) ) ;
#12154=CARTESIAN_POINT ( 'NONE',  ( 34.53678113438137842, -12.15940631226206925, -18.93201839848989465 ) ) ;
#12156=CARTESIAN_POINT ( 'NONE',  ( 9.641364314812712166, 17.66882920855936590, -17.90209449470656722 ) ) ;
#12159=CARTESIAN_POINT ( 'NONE',  ( 12.72883512080982804, 8.524354266104470668, -16.21679389071614352 ) ) ;
#12169=CARTESIAN_POINT ( 'NONE',  ( 11.22637516657937162, 9.079975409179585455, -17.24057027585384105 ) ) ;
#12171=CARTESIAN_POINT ( 'NONE',  ( 24.01829950071418907, -5.359185124211399476, -18.14381017295562160 ) ) ;
#12173=CARTESIAN_POINT ( 'NONE',  ( 24.68325608809179528, -0.07379305852225118145, -17.41420097001153167 ) ) ;
#12185=CARTESIAN_POINT ( 'NONE',  ( 10.55304143273637330, 16.08061740358965253, -17.30129946959702281 ) ) ;
#12191=CARTESIAN_POINT ( 'NONE',  ( 13.37957753592864663, 7.625938299336016968, -15.70790011242621453 ) ) ;
#12193=CARTESIAN_POINT ( 'NONE',  ( 20.14386580841007657, 1.771853782379294140, -13.30505882909219295 ) ) ;
#12194=CARTESIAN_POINT ( 'NONE',  ( 12.57288446902313872, 10.73011642529405307, -16.24829701787703939 ) ) ;
#12199=CARTESIAN_POINT ( 'NONE',  ( 10.82443827553465177, 12.24310121783546634, -16.12906421532448675 ) ) ;
#12201=CARTESIAN_POINT ( 'NONE',  ( 11.43229926783177497, 9.455373222906182207, -15.87769231223556332 ) ) ;
#12206=CARTESIAN_POINT ( 'NONE',  ( 12.35422140817580683, 8.720385185214494683, -16.48779044034850116 ) ) ;
#12208=CARTESIAN_POINT ( 'NONE',  ( 36.44920892064849482, -21.73803172434679354, -19.68085951391205057 ) ) ;
#12209=CARTESIAN_POINT ( 'NONE',  ( 17.15446488409023829, 10.64262399902749578, -18.76211774343175520 ) ) ;
#12210=CARTESIAN_POINT ( 'NONE',  ( 25.90632082398269276, -12.28056132945115841, -15.12647891527467969 ) ) ;
#12217=CARTESIAN_POINT ( 'NONE',  ( 32.20428705557502269, -10.20872362009771095, -14.89176492545819919 ) ) ;
#12219=SHAPE_DEFINITION_REPRESENTATION ( #24973, #22819 ) ;
#12220=CARTESIAN_POINT ( 'NONE',  ( 21.74214448781610542, 1.960522507982400020, -19.23370281053773923 ) ) ;
#12222=CARTESIAN_POINT ( 'NONE',  ( 29.36168402625536444, -8.616725751243539122, -15.73432514746931155 ) ) ;
#12230=CARTESIAN_POINT ( 'NONE',  ( 12.19589625337134997, 9.866176767462979669, -15.34419179356244634 ) ) ;
#12236=CARTESIAN_POINT ( 'NONE',  ( 12.49742530276927610, 8.569573706352677789, -15.13222638044318735 ) ) ;
#12238=CARTESIAN_POINT ( 'NONE',  ( 22.35455276305805938, 2.055732105393538678, -20.05127887597516434 ) ) ;
#12244=CARTESIAN_POINT ( 'NONE',  ( 11.26867954870061439, 16.71136643735313143, -16.78814161468471156 ) ) ;
#12246=CARTESIAN_POINT ( 'NONE',  ( 33.55945865873172096, -12.30028340163019607, -18.68418013052470883 ) ) ;
#12247=CARTESIAN_POINT ( 'NONE',  ( 17.32695330507268494, 5.471673316493076200, -20.08600194542987794 ) ) ;
#12250=CARTESIAN_POINT ( 'NONE',  ( 26.73315660230872837, -4.509142541826837380, -13.49646658189591619 ) ) ;
#12255=CARTESIAN_POINT ( 'NONE',  ( 25.47985489653468605, -2.350970512090694520, -13.88367939857760014 ) ) ;
#12256=CARTESIAN_POINT ( 'NONE',  ( 15.10317701704014226, 5.923596928851710075, -17.67988701311836053 ) ) ;
#12267=CARTESIAN_POINT ( 'NONE',  ( 11.46471852075427478, 9.306694396509932687, -15.86428581073749378 ) ) ;
#12268=CARTESIAN_POINT ( 'NONE',  ( 27.49606495187617128, -9.167791027049197794, -14.03786016821673677 ) ) ;
#12269=CARTESIAN_POINT ( 'NONE',  ( 21.55249387529322647, -4.041031698679099726, -14.19001464829599435 ) ) ;
#12271=CARTESIAN_POINT ( 'NONE',  ( 32.67186286342521839, -11.06527230177895227, -18.43913201350460440 ) ) ;
#12279=CARTESIAN_POINT ( 'NONE',  ( 21.19279910686179846, 4.720633506281588510, -19.26595127233560234 ) ) ;
#12282=CARTESIAN_POINT ( 'NONE',  ( 10.71275814632708823, 16.66803718250374899, -15.95787532639072914 ) ) ;
#12285=CARTESIAN_POINT ( 'NONE',  ( 21.79935899731381710, -1.430375723040585356, -13.25318265510616733 ) ) ;
#12286=CARTESIAN_POINT ( 'NONE',  ( 25.97279949409942290, -11.71600155862194015, -18.85018042282848683 ) ) ;
#12288=CARTESIAN_POINT ( 'NONE',  ( 32.36240160181304759, -11.00785621467150044, -17.57054915585148436 ) ) ;
#12289=CARTESIAN_POINT ( 'NONE',  ( 22.60637541839240683, -1.101515789306901194, -14.68923631892221948 ) ) ;
#12291=CARTESIAN_POINT ( 'NONE',  ( 19.31105547890425100, 3.022890346832332042, -18.89353813576326857 ) ) ;
#12293=CARTESIAN_POINT ( 'NONE',  ( 27.51083730600015897, -9.905735641176994122, -13.30399992039142099 ) ) ;
#12301=CARTESIAN_POINT ( 'NONE',  ( 34.38415957124060895, -12.46085888452578594, -19.93570721963346060 ) ) ;
#12302=CARTESIAN_POINT ( 'NONE',  ( 9.641350810849047548, 17.66889113945805789, -17.92981046679734547 ) ) ;
#12307=CARTESIAN_POINT ( 'NONE',  ( 13.11043623405165448, 8.565188957795726310, -15.92239833454181230 ) ) ;
#12315=CARTESIAN_POINT ( 'NONE',  ( 11.96143972814086531, 7.837808674300617007, -16.77422427047595477 ) ) ;
#12316=CARTESIAN_POINT ( 'NONE',  ( 23.79992313191835507, -8.927985498448517632, -17.01055530912027791 ) ) ;
#12317=CARTESIAN_POINT ( 'NONE',  ( 20.53420570626898822, -0.4664991210283321310, -19.04361528682417415 ) ) ;
#12329=CARTESIAN_POINT ( 'NONE',  ( 10.48009811366078381, 16.41514476298091907, -17.33146409796769660 ) ) ;
#12333=CARTESIAN_POINT ( 'NONE',  ( 35.37764311538968087, -21.41652447078215005, -19.89511094362359955 ) ) ;
#12335=CARTESIAN_POINT ( 'NONE',  ( 13.41328399211976397, 7.640833942120977440, -15.68103545992656578 ) ) ;
#12339=CARTESIAN_POINT ( 'NONE',  ( 23.56138260001205964, -6.829566487537672259, -18.05074380722902916 ) ) ;
#12340=CARTESIAN_POINT ( 'NONE',  ( 12.85916040382217318, 9.514151651470600157, -16.12251888295402580 ) ) ;
#12344=CARTESIAN_POINT ( 'NONE',  ( 11.47219014545126647, 9.272428573238919114, -15.86119603109536058 ) ) ;
#12346=CARTESIAN_POINT ( 'NONE',  ( 9.915538251416846194, 16.41143258624473233, -16.50493629029764264 ) ) ;
#12351=CARTESIAN_POINT ( 'NONE',  ( 12.03842576178837298, 9.272001309349649389, -16.68677036593512497 ) ) ;
#12353=CARTESIAN_POINT ( 'NONE',  ( 36.52535953212831998, -23.08013608362457703, -19.17046861472280028 ) ) ;
#12354=CARTESIAN_POINT ( 'NONE',  ( 24.78692427941192733, -9.284778175067517125, -17.23615439686343720 ) ) ;
#12355=CARTESIAN_POINT ( 'NONE',  ( 14.78952226657687063, 10.37904477376192069, -15.12939866669752575 ) ) ;
#12361=CARTESIAN_POINT ( 'NONE',  ( 33.30032953382602301, -10.37518355935928938, -17.98954529685971337 ) ) ;
#12363=CARTESIAN_POINT ( 'NONE',  ( 17.95893182911733277, 3.791778598950861667, -15.25628287466289024 ) ) ;
#12364=CARTESIAN_POINT ( 'NONE',  ( 18.55171814111300321, 6.637122934506423988, -19.73184648383247364 ) ) ;
#12369=DIRECTION ( 'NONE',  ( 0.000000000000000000, 0.000000000000000000, -1.000000000000000000 ) ) ;
#12377=CARTESIAN_POINT ( 'NONE',  ( 12.27584558688950978, 9.498490731067679604, -15.31120835137462244 ) ) ;
#12382=CARTESIAN_POINT ( 'NONE',  ( 12.50076791318051761, 8.571041463825640250, -15.12956297801270900 ) ) ;
#12384=CARTESIAN_POINT ( 'NONE',  ( 20.14260469057294500, 4.737385465944226048, -19.07682320266127718 ) ) ;
#12390=CARTESIAN_POINT ( 'NONE',  ( 11.53546837550287130, 15.48783886997274450, -16.67730506581143501 ) ) ;
#12392=CARTESIAN_POINT ( 'NONE',  ( 35.40392844931823646, -20.53461055239511879, -19.22110946685632271 ) ) ;
#12393=CARTESIAN_POINT ( 'NONE',  ( 15.39489021548154568, 6.697694061803245447, -14.95590323207311734 ) ) ;
#12396=CARTESIAN_POINT ( 'NONE',  ( 18.55888777153046121, 10.80885496093247689, -16.87139299526244685 ) ) ;
#12399=CARTESIAN_POINT ( 'NONE',  ( 20.97149233804390533, -0.06858483505933390956, -19.21322127741759189 ) ) ;
#12400=CARTESIAN_POINT ( 'NONE',  ( 18.06018518654990856, -2.098401534709970928, -17.02619504079518364 ) ) ;
#12413=CARTESIAN_POINT ( 'NONE',  ( 11.31072706937237982, 10.01291882189198112, -15.92796669285280764 ) ) ;
#12415=CARTESIAN_POINT ( 'NONE',  ( 28.13717792526295014, -10.23527491042630011, -17.83415580063453376 ) ) ;
#12416=CARTESIAN_POINT ( 'NONE',  ( 26.09074415779471323, -5.786596670875995940, -12.76770422508296932 ) ) ;
#12417=CARTESIAN_POINT ( 'NONE',  ( 33.38708106686501509, -12.47399286361455850, -19.70456970583452616 ) ) ;
#12425=CARTESIAN_POINT ( 'NONE',  ( 21.10023079691774228, -0.4353598523292347422, -20.14113737667230097 ) ) ;
#12428=CARTESIAN_POINT ( 'NONE',  ( 12.26149629667000340, 9.515828874666294013, -15.32083899563621898 ) ) ;
#12431=CARTESIAN_POINT ( 'NONE',  ( 21.19279910686179846, 4.720633506281588510, -19.26595127233560234 ) ) ;
#12432=CARTESIAN_POINT ( 'NONE',  ( 18.99162967131814028, 0.6168208955672017657, -19.54819510397825510 ) ) ;
#12434=CARTESIAN_POINT ( 'NONE',  ( 35.45944968151609800, -21.78403803824750185, -19.54251958818673174 ) ) ;
#12435=CARTESIAN_POINT ( 'NONE',  ( 27.61464345320196045, -4.235915813641956795, -14.29244051139929894 ) ) ;
#12436=CARTESIAN_POINT ( 'NONE',  ( 20.92249676953290916, 2.861121271339598593, -14.71414025844469720 ) ) ;
#12446=CARTESIAN_POINT ( 'NONE',  ( 18.55888777153046121, 10.80885496093247689, -16.87139299526244685 ) ) ;
#12448=CARTESIAN_POINT ( 'NONE',  ( 36.54859390953724585, -22.18451583373416014, -18.06010107863414405 ) ) ;
#12449=CARTESIAN_POINT ( 'NONE',  ( 9.745779815811758340, 17.18996641109745482, -16.82979807527155458 ) ) ;
#12453=CARTESIAN_POINT ( 'NONE',  ( 12.05017172662707381, 9.228765020691243492, -16.68110209197688221 ) ) ;
#12467=CARTESIAN_POINT ( 'NONE',  ( 11.46306169112780537, 8.437560028716553973, -17.10890052424691632 ) ) ;
#12469=CARTESIAN_POINT ( 'NONE',  ( 26.67611703245768950, -12.21101477627283849, -12.48819288018415108 ) ) ;
#12470=CARTESIAN_POINT ( 'NONE',  ( 25.46127020808262387, -4.208148299910691392, -19.59612275642668777 ) ) ;
#12483=CARTESIAN_POINT ( 'NONE',  ( 10.47193650065820592, 16.45257496057443802, -17.33483926051624735 ) ) ;
#12484=CARTESIAN_POINT ( 'NONE',  ( 32.91905456285188336, -11.74221475484424104, -17.14214516703887980 ) ) ;
#12486=CARTESIAN_POINT ( 'NONE',  ( 9.193626274318058123, 15.80945627937554576, -17.02118864906812234 ) ) ;
#12488=CARTESIAN_POINT ( 'NONE',  ( 25.23810427664335165, -6.496417100615061280, -13.69959235629456629 ) ) ;
#12489=CARTESIAN_POINT ( 'NONE',  ( 12.83296646064745339, 9.537815246119466295, -16.14070827264395547 ) ) ;
#12494=CARTESIAN_POINT ( 'NONE',  ( 12.46899830068120352, 8.557956911948249257, -15.15481108270911825 ) ) ;
#12499=CARTESIAN_POINT ( 'NONE',  ( 12.56022695423237145, 8.580358410770909217, -16.34122335808152826 ) ) ;
#12502=CARTESIAN_POINT ( 'NONE',  ( 34.26516872548082659, -12.92629604573065549, -20.94206068969455004 ) ) ;
#12503=CARTESIAN_POINT ( 'NONE',  ( 26.48263329513011755, -12.06126822337667903, -13.95730679897583038 ) ) ;
#12504=CARTESIAN_POINT ( 'NONE',  ( 26.38113052396219516, -11.59678093645141672, -17.84452879788985769 ) ) ;
#12512=CARTESIAN_POINT ( 'NONE',  ( 20.49785840140504689, 4.750029832917431527, -16.36601636927073145 ) ) ;
#12514=CARTESIAN_POINT ( 'NONE',  ( 19.11618317516819587, 7.271703427217982352, -19.10559232466456692 ) ) ;
#12524=CARTESIAN_POINT ( 'NONE',  ( 12.26149629667000340, 9.515828874666294013, -15.32083899563621898 ) ) ;
#12529=CARTESIAN_POINT ( 'NONE',  ( 12.50098444160134470, 8.571137227758441668, -15.12939039523150520 ) ) ;
#12531=CARTESIAN_POINT ( 'NONE',  ( 11.68234546060339163, 7.643720436761259229, -15.74430661255668262 ) ) ;
#12538=CARTESIAN_POINT ( 'NONE',  ( 12.85536779349230052, 9.514564043964993445, -16.12538237964846388 ) ) ;
#12540=CARTESIAN_POINT ( 'NONE',  ( 34.07550722110926955, -11.19626532300822674, -18.14763417942564061 ) ) ;
#12541=CARTESIAN_POINT ( 'NONE',  ( 17.85084670134855145, 5.929878015568476712, -20.08862479909851828 ) ) ;
#12545=CARTESIAN_POINT ( 'NONE',  ( 17.10097030076851610, 6.697663726599960121, -13.82760435466811089 ) ) ;
#12548=CARTESIAN_POINT ( 'NONE',  ( 26.02348467347448491, -3.622150272347476108, -19.21400332953221124 ) ) ;
#12551=CARTESIAN_POINT ( 'NONE',  ( 18.39947282702827991, 3.040288584705510999, -19.58888106367123427 ) ) ;
#12562=CARTESIAN_POINT ( 'NONE',  ( 11.40798482813988635, 9.566882342703072695, -15.88774718835883348 ) ) ;
#12563=CARTESIAN_POINT ( 'NONE',  ( 26.47302276827314671, -6.985584592454325836, -13.42065591321591711 ) ) ;
#12564=CARTESIAN_POINT ( 'NONE',  ( 25.66600519952783799, -8.909200411882650883, -19.30012332941604924 ) ) ;
#12565=CARTESIAN_POINT ( 'NONE',  ( 31.39893620166130717, -10.86152586746012183, -14.84747879817187943 ) ) ;
#12574=CARTESIAN_POINT ( 'NONE',  ( 19.83745040964868522, -2.306422872736943575, -14.39351019504378293 ) ) ;
#12577=CARTESIAN_POINT ( 'NONE',  ( 12.23642031952448406, 9.680328234467932447, -15.32743366668982432 ) ) ;
#12583=CARTESIAN_POINT ( 'NONE',  ( 16.89369580670022941, 0.5033910033923695293, -17.32063897790030893 ) ) ;
#12584=CARTESIAN_POINT ( 'NONE',  ( 18.25722813608836859, -0.08152059447761372812, -18.39925177747023710 ) ) ;
#12586=CARTESIAN_POINT ( 'NONE',  ( 35.07504771885155037, -20.05712364337910714, -20.21480690768607857 ) ) ;
#12587=( LENGTH_UNIT ( ) NAMED_UNIT ( * ) SI_UNIT ( .MILLI., .METRE. ) );
#12588=CARTESIAN_POINT ( 'NONE',  ( 25.85951265464835203, -2.375871015539448461, -16.96122936427994787 ) ) ;
#12589=CARTESIAN_POINT ( 'NONE',  ( 22.33422182767193576, -8.475443503041637072, -15.36134680393336538 ) ) ;
#12595=CARTESIAN_POINT ( 'NONE',  ( 21.94319337455657859, -4.318501116253552041, -18.82930321547734920 ) ) ;
#12603=CARTESIAN_POINT ( 'NONE',  ( 16.06097560829885040, 7.604535090956617616, -20.76572858943923094 ) ) ;
#12604=CARTESIAN_POINT ( 'NONE',  ( 36.48591233058812833, -21.90292070287360460, -19.44112467175505898 ) ) ;
#12605=CARTESIAN_POINT ( 'NONE',  ( 9.916953853453376766, 16.40494045485788632, -16.50434094533541085 ) ) ;
#12608=CARTESIAN_POINT ( 'NONE',  ( 12.04525852301462585, 9.245982119944198274, -16.68353927915122981 ) ) ;
#12620=CARTESIAN_POINT ( 'NONE',  ( 12.94178543664954972, 7.512178771719595360, -16.05074886939826939 ) ) ;
#12622=CARTESIAN_POINT ( 'NONE',  ( 28.02170931380428698, -7.325026966936788675, -12.85224998211816860 ) ) ;
#12624=CARTESIAN_POINT ( 'NONE',  ( 27.71186802668094273, -7.007055141436442369, -19.33373627201896383 ) ) ;
#12634=( BOUNDED_CURVE ( )  B_SPLINE_CURVE ( 3, ( #15500, #27145, #29141, #26996 ),
 .UNSPECIFIED., .F., .F. ) 
 B_SPLINE_CURVE_WITH_KNOTS ( ( 4, 4 ),
 ( 1.734723475976807094E-18, 0.001563228649568139134 ),
 .UNSPECIFIED. ) 
 CURVE ( )  GEOMETRIC_REPRESENTATION_ITEM ( )  RATIONAL_B_SPLINE_CURVE ( ( 1.000000000000000000, 0.3333333333333345361, 0.3333333333333333703, 0.9999999999999987788 ) ) 
 REPRESENTATION_ITEM ( '' )  );
#12640=CARTESIAN_POINT ( 'NONE',  ( 12.03006260835556951, 9.306948544855226046, -16.69048869075990638 ) ) ;
#12641=CARTESIAN_POINT ( 'NONE',  ( 32.97927115036063839, -11.75136040154610662, -17.31233706439427067 ) ) ;
#12643=CARTESIAN_POINT ( 'NONE',  ( 9.113591243665672081, 16.17650713204097102, -17.05428594964136835 ) ) ;
#12644=CARTESIAN_POINT ( 'NONE',  ( 27.31974442496251143, -5.660127319198639206, -14.41990313654811651 ) ) ;
#12645=CARTESIAN_POINT ( 'NONE',  ( 12.83122539074939894, 9.545332027449857648, -16.14146395906381670 ) ) ;
#12651=CARTESIAN_POINT ( 'NONE',  ( 12.13006862794127017, 8.527244997094612700, -15.41586291625151972 ) ) ;
#12657=CARTESIAN_POINT ( 'NONE',  ( 12.03055882466574289, 9.304755949677762317, -16.69027714870545864 ) ) ;
#12660=CARTESIAN_POINT ( 'NONE',  ( 19.69280650922798515, 8.111729275751024204, -19.45082099569356160 ) ) ;
#12661=CARTESIAN_POINT ( 'NONE',  ( 29.82081855766934453, -7.722587238354316597, -15.76009366473342332 ) ) ;
#12668=CARTESIAN_POINT ( 'NONE',  ( 17.24163842130223046, 3.474294283696999219, -15.80253352452890425 ) ) ;
#12669=CARTESIAN_POINT ( 'NONE',  ( 16.21960234321935701, 7.070186740785398882, -14.59618053200276044 ) ) ;
#12680=CARTESIAN_POINT ( 'NONE',  ( 12.27434273475605409, 9.502313893772186049, -15.31206391052669602 ) ) ;
#12685=CARTESIAN_POINT ( 'NONE',  ( 12.63667343406881294, 8.631100619704961119, -15.02124387326777111 ) ) ;
#12687=CARTESIAN_POINT ( 'NONE',  ( 10.66927416475804158, 9.041953549878499530, -16.41095583421565962 ) ) ;
#12694=CARTESIAN_POINT ( 'NONE',  ( 12.86387084073970222, 9.514634738764476296, -16.11888650007813339 ) ) ;
#12695=CARTESIAN_POINT ( 'NONE',  ( 34.53678113438137842, -12.15940631226206925, -18.93201839848989465 ) ) ;
#12697=CARTESIAN_POINT ( 'NONE',  ( 17.21692058948253035, 4.245457944912791604, -14.13226496128363863 ) ) ;
#12700=CARTESIAN_POINT ( 'NONE',  ( 31.01114313885700824, -11.37490951371675507, -12.31627997798639917 ) ) ;
#12704=CARTESIAN_POINT ( 'NONE',  ( 22.96196402503608169, -2.069733343145511828, -19.51364111617685992 ) ) ;
#12705=CARTESIAN_POINT ( 'NONE',  ( 18.87764716858279002, 3.471780965079254599, -19.68009874701989048 ) ) ;
#12716=CARTESIAN_POINT ( 'NONE',  ( 10.07879545831710999, 15.66271422494645904, -16.43741374977755143 ) ) ;
#12717=CARTESIAN_POINT ( 'NONE',  ( 25.72483820513325270, -9.972596264566449875, -15.12420980763781664 ) ) ;
#12718=CARTESIAN_POINT ( 'NONE',  ( 24.59975295023496855, -6.462932407320696626, -12.83695652901824147 ) ) ;
#12729=CARTESIAN_POINT ( 'NONE',  ( 20.23291344124205793, 5.521974472852556381, -14.51730806008046137 ) ) ;
#12732=CARTESIAN_POINT ( 'NONE',  ( 11.23952829215726901, 14.25220214615140257, -15.73968358775164056 ) ) ;
#12733=CARTESIAN_POINT ( 'NONE',  ( 32.52799721746220740, -11.03300674309804386, -18.03857687357939099 ) ) ;
#12736=CARTESIAN_POINT ( 'NONE',  ( 20.22088415693689356, -1.238650738454883493, -19.72259765018230482 ) ) ;
#12738=CARTESIAN_POINT ( 'NONE',  ( 20.08305308227469510, 0.3843232119764288246, -14.09874237319206358 ) ) ;
#12743=CARTESIAN_POINT ( 'NONE',  ( 24.25137658470242386, -8.936440734373054084, -19.04774169986686161 ) ) ;
#12745=CARTESIAN_POINT ( 'NONE',  ( 22.15378238435969394, -4.028439702987021143, -12.64872919198682943 ) ) ;
#12746=CARTESIAN_POINT ( 'NONE',  ( 25.79824969357368047, -12.24460132778619226, -15.92960863319586906 ) ) ;
#12754=CARTESIAN_POINT ( 'NONE',  ( 34.43765690731135720, -12.70119407716533111, -19.95187818093482335 ) ) ;
#12755=CARTESIAN_POINT ( 'NONE',  ( 9.879812780108833792, 16.57527415160161510, -16.52987074417163527 ) ) ;
#12761=CARTESIAN_POINT ( 'NONE',  ( 17.47275436513300662, 10.49281628697410262, -12.44556591811621082 ) ) ;
#12772=B_SPLINE_CURVE_WITH_KNOTS ( 'NONE', 3,
 ( #1604, #4029, #22952, #9029, #22796, #25236, #1904, #2052, #11331, #20338, #4322, #6767, #27107, #6169, #24793, #4173, #24947, #6613, #20191, #27416, #13178, #29572, #6320, #25084, #8591, #22504, #18053, #15616, #13621, #20637, #17889, #13324, #18200, #27270, #6467, #22648, #18353, #1747, #27709, #11036, #29728, #16059, #20493, #29879, #27561, #3732, #13029, #22346, #10743, #20052, #29424, #4478, #358, #2802, #9642, #4923, #23097, #21244, #25530, #204, #4769, #23240, #14362, #18961, #2511, #7221, #28315, #54, #507, #23697, #2200, #9793, #28009, #21402, #16215, #14065, #11777, #13913, #7376, #25993, #16671, #6922, #5070, #12083, #18663, #2356, #13768, #11628, #25844, #20940, #23394, #21097, #9484, #19110, #18807, #14216, #7068, #4622, #20788, #30173, #28166, #28464, #11469, #7513, #25387, #9181, #16515, #18507, #27865, #9335, #23544, #2648, #16362, #25684, #11924, #10542, #21694, #26595, #23859, #10392, #21550, #17122, #24296, #8102, #15116, #2957, #9939, #26447, #24151, #5381, #14809, #19701, #29065, #5683, #3255, #12835, #10088, #14666, #26146, #24011, #17266, #654, #5829, #14963, #19251, #16970, #3106, #24448, #28607, #21846, #7664, #17412, #26296, #3541, #12236, #1113, #22148, #1255, #956, #22007, #14515, #12382, #12529, #10240, #26759, #798, #19401, #19850, #29215, #16814, #5223, #28771, #7815, #5528, #3392, #19555, #28922, #7956, #12685, #8552, #15575, #17711, #1408, #22919 ),
 .UNSPECIFIED., .F., .F.,
 ( 4, 2, 2, 2, 2, 2, 2, 2, 2, 2, 2, 2, 2, 2, 2, 2, 2, 2, 2, 2, 2, 2, 2, 2, 2, 2, 2, 2, 2, 2, 2, 2, 2, 2, 2, 2, 2, 2, 2, 2, 2, 2, 2, 2, 2, 2, 2, 2, 2, 2, 2, 2, 2, 2, 2, 2, 2, 2, 2, 2, 2, 2, 2, 2, 2, 2, 2, 2, 2, 2, 2, 2, 2, 2, 2, 2, 2, 2, 2, 2, 2, 2, 2, 2, 2, 2, 2, 2, 2, 2, 2, 4 ),
 ( 0.000000000000000000, 0.2329478137359916601, 0.2349098735327963261, 0.2358909034311986452, 0.2363814183803998326, 0.2366266758550004123, 0.2367493045923006745, 0.2368106189609508194, 0.2368719333296009921, 0.2369056680493116518, 0.2369394027690223392, 0.2370068722084437141, 0.2371418110872864082, 0.2374116888449718521, 0.2379514443603427676, 0.2390309553910845153, 0.2411899774525680384, 0.2455080215755350015, 0.2541441098214690109, 0.2714162863133369741, 0.2886884628052049373, 0.2973245510511389189, 0.3016425951741059097, 0.3038016172355894051, 0.3048811282663311251, 0.3054208837817020128, 0.3056907615393874567, 0.3058257004182301508, 0.3058931698576515257, 0.3059269045773622131, 0.3059606392970729005, 0.3060023410584322701, 0.3060440428197916396, 0.3061274463425104342, 0.3062942533879479678, 0.3066278674788230352, 0.3072950956605731698, 0.3086295520240734391, 0.3112984647510739777, 0.3166362902050751105, 0.3273119411130773204, 0.3486632429290816848, 0.3913658465610905246, 0.4767710538251080932, 0.5621762610891257728, 0.6048788647211346126, 0.6262301665371389214, 0.6369058174451410759, 0.6422436428991421531, 0.6449125556261426917, 0.6462470119896429610, 0.6469142401713930957, 0.6472478542622682740, 0.6474146613077057522, 0.6474980648304246023, 0.6475397665917840273, 0.6475814683531433413, 0.6476196945210074274, 0.6476579206888716245, 0.6477343730245997966, 0.6478872776960561408, 0.6481930870389688293, 0.6488047057247942062, 0.6500279430964451821, 0.6524744178397469119, 0.6573673673263503714, 0.6671532662995571794, 0.6769391652727643205, 0.6867250642459713506, 0.6965109632191783806, 0.7062968621923852997, 0.7160827611655923297, 0.7209757106521957892, 0.7234221853954975190, 0.7246454227671484949, 0.7252570414529738718, 0.7255628507958865603, 0.7257157554673429045, 0.7257922078030710766, 0.7258304339709352737, 0.7258686601387993598, 0.7259088784260311344, 0.7259490967132626871, 0.7260295332877261254, 0.7261904064366527800, 0.7265121527345063113, 0.7271556453302132628, 0.7284426305216268327, 0.7310166009044544166, 0.7361645416701094735, 0.7464604232014194762, 0.7670521862640397037 ),
 .UNSPECIFIED. ) ;
#12775=CARTESIAN_POINT ( 'NONE',  ( 13.27290874800832121, 7.583804977141803683, -15.79253525446438999 ) ) ;
#12776=CARTESIAN_POINT ( 'NONE',  ( 27.89044320811645505, -9.967159925860730851, -19.81290489186636350 ) ) ;
#12777=CARTESIAN_POINT ( 'NONE',  ( 28.56280713547801398, -4.978584871567802494, -14.74258920993753641 ) ) ;
#12792=CARTESIAN_POINT ( 'NONE',  ( 13.12299649507002464, 8.570581087883812899, -15.91239967140973022 ) ) ;
#12793=CARTESIAN_POINT ( 'NONE',  ( 35.54787733059053778, -22.18129662410796854, -18.46719521006932396 ) ) ;
#12795=CARTESIAN_POINT ( 'NONE',  ( 9.128787768473113573, 16.10681393216777835, -17.04800165206417972 ) ) ;
#12798=CARTESIAN_POINT ( 'NONE',  ( 27.83100014064079275, -5.545984359997562230, -15.13782040115233052 ) ) ;
#12800=CARTESIAN_POINT ( 'NONE',  ( 10.35865057885519214, 16.97211863855931924, -17.91295731025335414 ) ) ;
#12806=CARTESIAN_POINT ( 'NONE',  ( 12.29195110325218288, 8.516770644378290456, -15.29309475950548958 ) ) ;
#12811=CARTESIAN_POINT ( 'NONE',  ( 12.02305193244137449, 9.338961869187645704, -16.69339841729684437 ) ) ;
#12813=CARTESIAN_POINT ( 'NONE',  ( 21.84805831652669283, 4.237162156985878170, -20.00989837289113282 ) ) ;
#12814=CARTESIAN_POINT ( 'NONE',  ( 19.73194482477335399, 0.5267938184197646923, -13.16654652480547583 ) ) ;
#12817=CARTESIAN_POINT ( 'NONE',  ( 35.77509030908504428, -18.70957389315904962, -20.35615221346758474 ) ) ;
#12819=CARTESIAN_POINT ( 'NONE',  ( 18.21616227284554057, 4.699354889203569918, -13.86658597208997179 ) ) ;
#12825=CARTESIAN_POINT ( 'NONE',  ( 33.75544676243647757, -14.12885555826641593, -19.81592319558764004 ) ) ;
#12829=CARTESIAN_POINT ( 'NONE',  ( 12.27687350794345456, 9.494798321042301481, -15.31070534102384251 ) ) ;
#12835=CARTESIAN_POINT ( 'NONE',  ( 11.77869587587188249, 8.711114196793760200, -15.67004689359726299 ) ) ;
#12836=EDGE_LOOP ( 'NONE', ( #4751, #23825, #24428, #28171, #24271 ) ) ;
#12838=CARTESIAN_POINT ( 'NONE',  ( 10.40934825891211979, 10.23400028951819607, -16.51844484289298265 ) ) ;
#12843=CARTESIAN_POINT ( 'NONE',  ( 12.83173194157631514, 9.543008920787411142, -16.14125448247791184 ) ) ;
#12845=CARTESIAN_POINT ( 'NONE',  ( 34.55638066306561029, -12.23714146529668234, -18.94394112255963236 ) ) ;
#12846=CARTESIAN_POINT ( 'NONE',  ( 21.69765170278760280, -5.035756590920279940, -14.89200278627170881 ) ) ;
#12850=CARTESIAN_POINT ( 'NONE',  ( 27.15828739042733631, -11.95405637977086677, -19.54710185400437794 ) ) ;
#12854=CARTESIAN_POINT ( 'NONE',  ( 19.39950943988042553, -1.649204456521256246, -16.58530004841527727 ) ) ;
#12855=CARTESIAN_POINT ( 'NONE',  ( 19.55603740332541918, 4.113176889600292263, -19.54140316641015573 ) ) ;
#12866=CARTESIAN_POINT ( 'NONE',  ( 11.46877092736959014, 9.288109543210406827, -15.86260999805022820 ) ) ;
#12867=CARTESIAN_POINT ( 'NONE',  ( 17.69365662292968366, 10.27476822432933545, -17.01437286930526227 ) ) ;
#12868=CARTESIAN_POINT ( 'NONE',  ( 24.77705064808911217, -2.604154092221317551, -13.46095375842554098 ) ) ;
#12876=CARTESIAN_POINT ( 'NONE',  ( 17.88091890332929523, 4.544920326333207861, -13.91018511019278669 ) ) ;
#12879=CARTESIAN_POINT ( 'NONE',  ( 12.27688791398868950, 9.494734666090453246, -15.31069919958039804 ) ) ;
#12882=CARTESIAN_POINT ( 'NONE',  ( 23.36212950203212557, 2.915605996956767587, -15.34809340432955693 ) ) ;
#12885=CARTESIAN_POINT ( 'NONE',  ( 21.03983889671009422, 4.536326888612346231, -13.89983168792289270 ) ) ;
#12889=CARTESIAN_POINT ( 'NONE',  ( 25.50153931649120764, -9.195696458170099064, -12.32940773450113170 ) ) ;
#12890=CARTESIAN_POINT ( 'NONE',  ( 22.17025134254096130, -8.444422103036636429, -16.38876926059057126 ) ) ;
#12904=CARTESIAN_POINT ( 'NONE',  ( 27.25745087693901425, -5.581270904725432302, -18.17424208600867175 ) ) ;
#12906=CARTESIAN_POINT ( 'NONE',  ( 36.53271160917758209, -22.11316507130252873, -18.90714217169671230 ) ) ;
#12908=CARTESIAN_POINT ( 'NONE',  ( 9.915538251416846194, 16.41143258624473233, -16.50493629029764264 ) ) ;
#12911=CARTESIAN_POINT ( 'NONE',  ( 9.661883061612440926, 16.25482663361732705, -17.92279151347708677 ) ) ;
#12914=CARTESIAN_POINT ( 'NONE',  ( 11.55687758731922798, 9.016417257711555777, -15.81607864292198329 ) ) ;
#12922=CARTESIAN_POINT ( 'NONE',  ( 8.944584683310379702, 16.95159276115599667, -17.91664992932185996 ) ) ;
#12923=CARTESIAN_POINT ( 'NONE',  ( 30.38377115645388571, -7.011354780429720712, -16.65419678813778503 ) ) ;
#12924=CARTESIAN_POINT ( 'NONE',  ( 25.05301747714807448, -9.477991407908255894, -18.78921932654604632 ) ) ;
#12942=CARTESIAN_POINT ( 'NONE',  ( 13.09018272752966716, 8.557097568986355540, -15.93847522207377310 ) ) ;
#12943=CARTESIAN_POINT ( 'NONE',  ( 33.19002920664139111, -11.78337016499817658, -17.90800870513906773 ) ) ;
#12946=CARTESIAN_POINT ( 'NONE',  ( 8.977559110355956662, 16.80036783546273327, -17.41076197725142194 ) ) ;
#12948=CARTESIAN_POINT ( 'NONE',  ( 25.55230692589818631, -0.5649882819070038975, -17.32853901032857280 ) ) ;
#12949=CARTESIAN_POINT ( 'NONE',  ( 12.86818510107347890, 9.516005823298000266, -16.11548879760486130 ) ) ;
#12954=CARTESIAN_POINT ( 'NONE',  ( 11.55687758731922798, 9.016417257711555777, -15.81607864292198329 ) ) ;
#12959=CARTESIAN_POINT ( 'NONE',  ( 13.17827647522021906, 8.595009676161804890, -15.86834059905992511 ) ) ;
#12962=CARTESIAN_POINT ( 'NONE',  ( 19.20998527735078198, 1.665648160765265784, -20.80323043525838855 ) ) ;
#12963=CARTESIAN_POINT ( 'NONE',  ( 18.86526831082781541, 1.353360947173176232, -20.65364330072180366 ) ) ;
#12967=CARTESIAN_POINT ( 'NONE',  ( 36.54859590101256828, -22.18452478037840336, -18.26685560724362034 ) ) ;
#12970=CARTESIAN_POINT ( 'NONE',  ( 17.32695330507268494, 5.471673316493076200, -20.08600194542987794 ) ) ;
#12980=CARTESIAN_POINT ( 'NONE',  ( 32.68951927270060764, -11.07419627511998605, -18.48540492261787449 ) ) ;
#12985=CARTESIAN_POINT ( 'NONE',  ( 12.24516416863347956, 9.516115402270077794, -15.33328367062981279 ) ) ;
#12993=CARTESIAN_POINT ( 'NONE',  ( 12.22241433628510165, 7.513235304754858568, -15.34201686955167609 ) ) ;
#12999=CARTESIAN_POINT ( 'NONE',  ( 12.83240265444113071, 9.539962209189782882, -16.14097488725632346 ) ) ;
#13000=CARTESIAN_POINT ( 'NONE',  ( 36.21506517127201619, -19.68614788779310132, -19.44682451121369482 ) ) ;
#13001=CARTESIAN_POINT ( 'NONE',  ( 23.36212950203212557, 2.915605996956767587, -15.34809340432955693 ) ) ;
#13003=CARTESIAN_POINT ( 'NONE',  ( 13.78676817088038931, 5.425489125369224119, -17.89072192914586168 ) ) ;
#13006=CARTESIAN_POINT ( 'NONE',  ( 30.50670359208957905, -8.903545733563623443, -17.67935522427464079 ) ) ;
#13007=CARTESIAN_POINT ( 'NONE',  ( 23.36829581039676640, 3.373260575288004937, -18.04565522708177738 ) ) ;
#13021=CARTESIAN_POINT ( 'NONE',  ( 13.36280753930113363, 7.618652675320872980, -15.72125653641924892 ) ) ;
#13023=CARTESIAN_POINT ( 'NONE',  ( 10.33811693838771717, 18.38618951776012267, -17.92454625180715411 ) ) ;
#13024=CARTESIAN_POINT ( 'NONE',  ( 29.02390443993225588, -5.138988301204332920, -16.36505798003706857 ) ) ;
#13029=CARTESIAN_POINT ( 'NONE',  ( 9.898178882064430084, 16.49104486689975246, -16.51464960819000893 ) ) ;
#13032=CARTESIAN_POINT ( 'NONE',  ( 22.09544204423535874, -4.864148257255451746, -14.35781331922719772 ) ) ;
#13036=CARTESIAN_POINT ( 'NONE',  ( 12.19589625337134997, 9.866176767462979669, -15.34419179356244634 ) ) ;
#13041=CARTESIAN_POINT ( 'NONE',  ( 22.97938783112199701, -3.359759438970757017, -19.62490732200095067 ) ) ;
#13043=CARTESIAN_POINT ( 'NONE',  ( 16.82931527361030533, 7.354042003703605168, -13.11858969620360504 ) ) ;
#13046=CARTESIAN_POINT ( 'NONE',  ( 23.38597214775318278, -9.778565425610747042, -17.35394146810280347 ) ) ;
#13047=CARTESIAN_POINT ( 'NONE',  ( 23.10480167063333212, 0.6704577443818302562, -13.62402792225823944 ) ) ;
#13048=CARTESIAN_POINT ( 'NONE',  ( 27.76312469413510442, -10.32446017237915648, -18.80420148706337358 ) ) ;
#13056=CARTESIAN_POINT ( 'NONE',  ( 24.53726495287250486, -4.893489461768670168, -18.28393818840952534 ) ) ;
#13057=CARTESIAN_POINT ( 'NONE',  ( 17.27944038698359464, 10.59897317215052226, -14.78577975581568360 ) ) ;
#13058=CARTESIAN_POINT ( 'NONE',  ( 34.03885009341546208, -11.93819216554969742, -20.85700406890413916 ) ) ;
#13061=CARTESIAN_POINT ( 'NONE',  ( 9.914377700407460026, 16.41675502110963336, -16.50544604630902867 ) ) ;
#13064=CARTESIAN_POINT ( 'NONE',  ( 9.661883795922106444, 16.25482326597959926, -17.91529654610192424 ) ) ;
#13068=CARTESIAN_POINT ( 'NONE',  ( 11.47511325496290624, 9.259230714725578792, -15.85997136665693041 ) ) ;
#13075=CARTESIAN_POINT ( 'NONE',  ( 16.77165338796101324, 10.12286561294300569, -15.51291369241808304 ) ) ;
#13077=CARTESIAN_POINT ( 'NONE',  ( 8.944584694422324844, 16.95159271019519664, -17.91554756312530117 ) ) ;
#13078=CARTESIAN_POINT ( 'NONE',  ( 34.69314741404605229, -14.84897758684750890, -21.07142838010442176 ) ) ;
#13080=CARTESIAN_POINT ( 'NONE',  ( 25.64452216564459164, -12.66255397501067570, -13.70049860994083701 ) ) ;
#13081=CARTESIAN_POINT ( 'NONE',  ( 24.59975295023496855, -6.462932407320696626, -12.83695652901824147 ) ) ;
#13087=FILL_AREA_STYLE ('',( #22569 ) ) ;
#13090=CARTESIAN_POINT ( 'NONE',  ( 12.03309083968702886, 9.293808706017943067, -16.68917936036902105 ) ) ;
#13091=CARTESIAN_POINT ( 'NONE',  ( 35.54859390953724585, -21.18451583373416014, -17.99055332684694974 ) ) ;
#13094=CARTESIAN_POINT ( 'NONE',  ( 9.631286188771861489, 13.80229212302790920, -16.84020087884530881 ) ) ;
#13096=CARTESIAN_POINT ( 'NONE',  ( 27.26129135193747999, -10.77754955263135095, -18.64424489656416739 ) ) ;
#13097=CARTESIAN_POINT ( 'NONE',  ( 10.35864918915110877, 16.97212501191939538, -17.91664992932186351 ) ) ;
#13105=CARTESIAN_POINT ( 'NONE',  ( 11.47464782381437587, 9.261287281732329291, -15.86016978468419936 ) ) ;
#13111=CARTESIAN_POINT ( 'NONE',  ( 13.12341270237516078, 8.570764515250925086, -15.91206798513452192 ) ) ;
#13113=CARTESIAN_POINT ( 'NONE',  ( 14.76280285026742867, 7.190900411307756812, -14.35234371774122408 ) ) ;
#13114=CARTESIAN_POINT ( 'NONE',  ( 18.01687101988986583, 8.608027666922664523, -14.27462087050975015 ) ) ;
#13117=CARTESIAN_POINT ( 'NONE',  ( 35.48977118337261771, -17.42778619908077076, -20.26990708652652629 ) ) ;
#13120=CARTESIAN_POINT ( 'NONE',  ( 19.40121574091639189, 1.432572567346982240, -13.43353846741550406 ) ) ;
#13121=COLOUR_RGB ( '', 0.66274510, 0.83137255, 0.94901961) ;
#13126=CARTESIAN_POINT ( 'NONE',  ( 32.36240160181304759, -11.00785621467150044, -17.57054915585148436 ) ) ;
#13131=CARTESIAN_POINT ( 'NONE',  ( 11.05541531668977662, 17.68942339022145305, -17.98596209335946128 ) ) ;
#13132=CARTESIAN_POINT ( 'NONE',  ( 35.53993026725221682, -23.14559467820676275, -18.82474504553469075 ) ) ;
#13138=CARTESIAN_POINT ( 'NONE',  ( 10.66819573146529621, 9.046892785011555915, -16.41140230749465800 ) ) ;
#13149=CARTESIAN_POINT ( 'NONE',  ( 12.86812980024498643, 9.515982172609518841, -16.11553281326163045 ) ) ;
#13150=CARTESIAN_POINT ( 'NONE',  ( 36.30315773322485740, -20.08190110472122214, -19.47147371593984388 ) ) ;
#13151=CARTESIAN_POINT ( 'NONE',  ( 18.97268594440662426, -2.511067197207834667, -17.06021009607598415 ) ) ;
#13158=CARTESIAN_POINT ( 'NONE',  ( 26.69342817538273138, -7.978421288772274522, -19.59580293194042966 ) ) ;
#13159=CARTESIAN_POINT ( 'NONE',  ( 25.59095072769168766, -7.385909681514642777, -13.40699837787023618 ) ) ;
#13170=CARTESIAN_POINT ( 'NONE',  ( 12.16405474897817207, 7.700086518927777846, -16.63006945039463247 ) ) ;
#13171=CARTESIAN_POINT ( 'NONE',  ( 12.49742530276927610, 8.569573706352677789, -15.13222638044318735 ) ) ;
#13178=CARTESIAN_POINT ( 'NONE',  ( 9.641351021852148762, 17.66889017177091503, -17.91406276888456617 ) ) ;
#13184=CARTESIAN_POINT ( 'NONE',  ( 23.60870351872479844, -7.222488552757559077, -14.83554404960226947 ) ) ;
#13189=CARTESIAN_POINT ( 'NONE',  ( 16.59405769476016701, 11.43796928512929867, -11.86713876492064124 ) ) ;
#13190=AXIS2_PLACEMENT_3D ( 'NONE', #5435, #19606, #10446 ) ;
#13193=CARTESIAN_POINT ( 'NONE',  ( 26.18758235895636233, -4.355437658720127558, -18.53605802859044260 ) ) ;
#13195=CARTESIAN_POINT ( 'NONE',  ( 21.44242187996815119, -3.785596145164559445, -16.19382493935754397 ) ) ;
#13200=CARTESIAN_POINT ( 'NONE',  ( 15.17188473929424930, 6.803351907998973935, -20.50413427079521256 ) ) ;
#13201=CARTESIAN_POINT ( 'NONE',  ( 25.20506945179333513, 0.8918220058822420304, -17.26233558910082166 ) ) ;
#13213=CARTESIAN_POINT ( 'NONE',  ( 23.91915341143258544, -8.806945430038833678, -17.38103690300000181 ) ) ;
#13214=CARTESIAN_POINT ( 'NONE',  ( 18.23802153489769751, 0.9697156596711644649, -18.35043786425562828 ) ) ;
#13215=CARTESIAN_POINT ( 'NONE',  ( 32.39840662109286029, -9.588391805189495187, -17.44209920064860597 ) ) ;
#13217=CARTESIAN_POINT ( 'NONE',  ( 11.47338783222600789, 9.266948822715743717, -15.86069975447064806 ) ) ;
#13220=CARTESIAN_POINT ( 'NONE',  ( 13.15105351193492744, 8.582979361647906202, -15.89003778131599098 ) ) ;
#13226=CARTESIAN_POINT ( 'NONE',  ( 12.77278825050581013, 8.691252192278360766, -14.91275796197543890 ) ) ;
#13235=CARTESIAN_POINT ( 'NONE',  ( 13.40647825129878612, 7.637826363492710158, -15.68645975549014082 ) ) ;
#13236=CARTESIAN_POINT ( 'NONE',  ( 32.11502935538656800, -10.34531343835429062, -18.85863636141847621 ) ) ;
#13238=CARTESIAN_POINT ( 'NONE',  ( 14.70433163182692482, 6.391443753141328621, -13.74806202935933541 ) ) ;
#13239=CARTESIAN_POINT ( 'NONE',  ( 27.15223745481332784, -12.21752729395051063, -18.24437427626675046 ) ) ;
#13243=CARTESIAN_POINT ( 'NONE',  ( 17.46640274557904959, 4.060524459741898795, -18.82505950134852313 ) ) ;
#13251=CARTESIAN_POINT ( 'NONE',  ( 13.05603179413191839, 8.545058472539723837, -15.96546128479914373 ) ) ;
#13252=CARTESIAN_POINT ( 'NONE',  ( 33.98143228033899987, -14.14408878234146982, -18.84191164812894570 ) ) ;
#13254=CARTESIAN_POINT ( 'NONE',  ( 12.74324588813389170, 7.620242904383297322, -14.93629796730785486 ) ) ;
#13257=CARTESIAN_POINT ( 'NONE',  ( 28.09718568327657806, -5.958257988085632562, -17.17874431236187149 ) ) ;
#13258=CARTESIAN_POINT ( 'NONE',  ( 13.30397322184224329, 9.708587077508630259, -15.76815807330931030 ) ) ;
#13263=CARTESIAN_POINT ( 'NONE',  ( 12.50736435846123484, 8.573956625762026107, -15.12430548898761806 ) ) ;
#13269=CARTESIAN_POINT ( 'NONE',  ( 16.24089679924285790, 9.948436389806387226, -13.42737814189079337 ) ) ;
#13270=CARTESIAN_POINT ( 'NONE',  ( 21.88956083454650781, 5.816198478639956093, -14.73130718433538178 ) ) ;
#13271=CARTESIAN_POINT ( 'NONE',  ( 17.13759149762038803, 5.494404601539362609, -21.09448147619161418 ) ) ;
#13274=CARTESIAN_POINT ( 'NONE',  ( 16.94076125623460527, 0.4124075662712927692, -16.40086227390004936 ) ) ;
#13289=CARTESIAN_POINT ( 'NONE',  ( 11.05541529015696156, 17.68942351190433726, -17.91624098666951070 ) ) ;
#13293=CARTESIAN_POINT ( 'NONE',  ( 12.75629879507850717, 7.625935294889710114, -14.92590036059129943 ) ) ;
#13299=CARTESIAN_POINT ( 'NONE',  ( 10.35864918915110877, 16.97212501191939538, -17.91796598306941135 ) ) ;
#13300=CARTESIAN_POINT ( 'NONE',  ( 35.91774987194125401, -19.35046774019819438, -20.39927477693754554 ) ) ;
#13301=CARTESIAN_POINT ( 'NONE',  ( 20.22088415693689356, -1.238650738454883493, -19.72259765018230482 ) ) ;
#13306=CARTESIAN_POINT ( 'NONE',  ( 29.49448338005720416, -10.05855281841770221, -18.88094824714235642 ) ) ;
#13307=CARTESIAN_POINT ( 'NONE',  ( 25.48002462322397577, -3.608900787083736184, -12.74538502395823691 ) ) ;
#13318=CARTESIAN_POINT ( 'NONE',  ( 11.26737699260669778, 8.919714795263022467, -17.22149591130980184 ) ) ;
#13319=CARTESIAN_POINT ( 'NONE',  ( 12.50268541164654756, 8.571888915454989544, -15.12803469218787811 ) ) ;
#13320=CARTESIAN_POINT ( 'NONE',  ( 27.15223745481332784, -12.21752729395051063, -18.24437427626675046 ) ) ;
#13324=CARTESIAN_POINT ( 'NONE',  ( 9.641890818133653340, 17.66641459721583374, -17.82828029666912073 ) ) ;
#13328=CARTESIAN_POINT ( 'NONE',  ( 20.72626264887238534, -1.914771856900582714, -13.62749948506543518 ) ) ;
#13332=CARTESIAN_POINT ( 'NONE',  ( 14.13034256312282189, 10.34920949090176201, -13.83076321228938887 ) ) ;
#13334=CARTESIAN_POINT ( 'NONE',  ( 33.96943610671532809, -15.09019632882451134, -19.88060704079178720 ) ) ;
#13337=CARTESIAN_POINT ( 'NONE',  ( 25.04992766293576878, -3.547109489677171101, -13.67097983722207033 ) ) ;
#13339=CARTESIAN_POINT ( 'NONE',  ( 22.40033610297568956, 1.362009800809227178, -14.54093962742820700 ) ) ;
#13340=ORIENTED_EDGE ( 'NONE', *, *, #14608, .T. ) ;
#13342=CARTESIAN_POINT ( 'NONE',  ( 14.30110556002302680, 5.443193088601498530, -15.49285935407157666 ) ) ;
#13343=CARTESIAN_POINT ( 'NONE',  ( 28.63790973356518776, -5.888324979419876648, -13.82040474618100312 ) ) ;
#13356=CARTESIAN_POINT ( 'NONE',  ( 9.641350810849047548, 17.66889113945805789, -17.93331994345748370 ) ) ;
#13357=CARTESIAN_POINT ( 'NONE',  ( 23.38178567734072999, -4.037937620979102249, -14.56836966348588369 ) ) ;
#13358=CARTESIAN_POINT ( 'NONE',  ( 19.14398323884976350, 7.495936751868839565, -14.71076302495156263 ) ) ;
#13359=CARTESIAN_POINT ( 'NONE',  ( 34.16709027601721971, -12.48568152589075098, -20.91241392730897886 ) ) ;
#13361=CARTESIAN_POINT ( 'NONE',  ( 12.43696608443014284, 8.546664718661613591, -15.18012293544581226 ) ) ;
#13365=CARTESIAN_POINT ( 'NONE',  ( 9.661883061612440926, 16.25482663361732705, -19.66666666666843000 ) ) ;
#13369=CARTESIAN_POINT ( 'NONE',  ( 12.50035968906703765, 8.570861208087439564, -15.12988832871674560 ) ) ;
#13376=CARTESIAN_POINT ( 'NONE',  ( 13.37966566800644763, 7.625977406171305262, -15.70782985742499527 ) ) ;
#13377=CARTESIAN_POINT ( 'NONE',  ( 30.54120030308987666, -10.08143909378498293, -14.42492330020037272 ) ) ;
#13378=CARTESIAN_POINT ( 'NONE',  ( 19.35412429307980986, 8.340480409601783052, -14.20924892776020343 ) ) ;
#13379=CARTESIAN_POINT ( 'NONE',  ( 18.16542447708646790, 4.701683080007062365, -19.22226433900947029 ) ) ;
#13382=CARTESIAN_POINT ( 'NONE',  ( 22.44149885728860028, -8.037961521189897596, -18.19026436706728234 ) ) ;
#13394=CARTESIAN_POINT ( 'NONE',  ( 33.87301206822314725, -11.11198276574163302, -17.60644260715651299 ) ) ;
#13396=CARTESIAN_POINT ( 'NONE',  ( 10.66961851098191083, 9.040384230280389843, -16.41081268017797257 ) ) ;
#13398=CARTESIAN_POINT ( 'NONE',  ( 25.24878800877705487, -9.370948223588685622, -14.18615728435988288 ) ) ;
#13400=CARTESIAN_POINT ( 'NONE',  ( 12.86837137031974621, 9.516086858917468305, -16.11534043535873906 ) ) ;
#13411=CARTESIAN_POINT ( 'NONE',  ( 13.11965390131543430, 8.569119222385459977, -15.91506261175275760 ) ) ;
#13413=CARTESIAN_POINT ( 'NONE',  ( 19.97442599234820193, -2.778558858265142373, -17.76606689721253574 ) ) ;
#13414=CARTESIAN_POINT ( 'NONE',  ( 15.83402620853355636, 4.298615461832955731, -20.35054180922590916 ) ) ;
#13417=CARTESIAN_POINT ( 'NONE',  ( 20.52488529563827058, 3.974637744936419637, -19.97762432673833288 ) ) ;
#13424=CARTESIAN_POINT ( 'NONE',  ( 10.47079889355419446, 16.45779217176459852, -17.33533584583738829 ) ) ;
#13425=CARTESIAN_POINT ( 'NONE',  ( 33.41663030065195272, -12.60673267154789201, -19.71350710734569134 ) ) ;
#13430=CARTESIAN_POINT ( 'NONE',  ( 15.14574614762244487, 6.587483969391940697, -15.14885142785537830 ) ) ;
#13431=CARTESIAN_POINT ( 'NONE',  ( 12.24726067228269422, 9.517041913610183812, -15.33161271801373182 ) ) ;
#13437=CARTESIAN_POINT ( 'NONE',  ( 15.87304960759194650, 9.003283391651189405, -12.44179493704351280 ) ) ;
#13442=CARTESIAN_POINT ( 'NONE',  ( 10.35865005771744762, 16.97212102856341787, -17.91352035578586310 ) ) ;
#13446=CARTESIAN_POINT ( 'NONE',  ( 32.71419323209526908, -10.28616775856061416, -16.33292762241428520 ) ) ;
#13447=CARTESIAN_POINT ( 'NONE',  ( 25.55230692589818631, -0.5649882819070038975, -17.32853901032857280 ) ) ;
#13452=CARTESIAN_POINT ( 'NONE',  ( 27.87518295380144551, -11.54787579004265652, -18.81772651352153858 ) ) ;
#13453=CARTESIAN_POINT ( 'NONE',  ( 27.54556670433429488, -3.970347839692917713, -18.20727554117155123 ) ) ;
#13463=CARTESIAN_POINT ( 'NONE',  ( 10.33811693838771717, 18.38618951776012267, -17.92015940598198753 ) ) ;
#13470=CARTESIAN_POINT ( 'NONE',  ( 18.77375537285786322, 7.252522315878067616, -16.50763127152984566 ) ) ;
#13473=CARTESIAN_POINT ( 'NONE',  ( 23.22413189157496305, -7.367447486509826504, -15.63851824576001981 ) ) ;
#13477=CARTESIAN_POINT ( 'NONE',  ( 12.24938746628909492, 9.517981781931423413, -15.32991762565031202 ) ) ;
#13479=CARTESIAN_POINT ( 'NONE',  ( 33.48796008207983022, -12.92717959506727965, -19.73506838908087246 ) ) ;
#13484=CARTESIAN_POINT ( 'NONE',  ( 21.43917814492346707, -4.799604530101110988, -17.97822123721208243 ) ) ;
#13487=B_SPLINE_CURVE_WITH_KNOTS ( 'NONE', 3,
 ( #1863, #8843, #16014, #23055, #13582, #13727, #9288, #27962, #13868, #25340, #156, #16313, #4430, #22906, #11140, #7023, #20444, #25630, #11577, #20892, #28113, #29838, #2010, #2154, #11427, #11290, #20734, #14010, #23343, #23191, #30126, #9434, #2458, #9133, #20593, #29976, #16168, #18461, #11732, #8982, #27814, #21050, #18304, #27659, #6880, #2304, #3, #18760, #15714, #25046, #4131, #13424, #309, #23809, #4871, #9592, #26247, #25790, #21350, #12483, #16622, #18913, #5481, #28267, #14313, #21807, #28560, #17077, #7470, #7319, #16464, #14168, #23494, #12329, #14764, #21645, #16917, #2604, #3056, #25941, #12185, #11878, #5022, #26402, #743, #14468, #19204, #10041, #12036, #904, #24103, #21192, #10196, #9742, #3205, #23648, #16773, #2907, #2749, #19354, #7764, #456, #19060, #28715, #19508, #28416, #26097, #5176, #21503, #7614, #605, #9894, #5334, #14618, #7173, #23967, #17670, #1212, #19655, #24256, #3353, #12640, #17812, #14916, #13090, #27185, #3950, #3647, #3800, #26552, #15068, #8364, #22256, #6238, #21957, #15533, #29495, #24406, #26873, #1069, #10349, #24865, #10494, #8055, #29020, #13251, #24555, #12942, #29166, #10951, #1364, #10652, #8206, #22571, #22416, #19966, #3502, #17364, #12792, #1671, #22110, #5938, #28882, #26713, #17518, #7914, #17225, #15222, #29335, #5633, #5785, #19806, #27027, #6082, #15378, #24712, #1522, #10805, #20115, #8513, #18577, #11256, #2124, #4396 ),
 .UNSPECIFIED., .F., .F.,
 ( 4, 2, 2, 2, 2, 2, 2, 2, 2, 2, 2, 2, 2, 2, 2, 2, 2, 2, 2, 2, 2, 2, 2, 2, 2, 2, 2, 2, 2, 2, 2, 2, 2, 2, 2, 2, 2, 2, 2, 2, 2, 2, 2, 2, 2, 2, 2, 2, 2, 2, 2, 2, 2, 2, 2, 2, 2, 2, 2, 2, 2, 2, 2, 2, 2, 2, 2, 2, 2, 2, 2, 2, 2, 2, 2, 2, 2, 2, 2, 2, 2, 2, 2, 2, 2, 2, 2, 2, 2, 2, 2, 4 ),
 ( 0.000000000000000000, 0.2329478137359917711, 0.2349098735327964371, 0.2358909034311987563, 0.2363814183803999158, 0.2366266758550005234, 0.2367493045923007855, 0.2368106189609509304, 0.2368719333296011031, 0.2369056680493117628, 0.2369394027690224502, 0.2370068722084438251, 0.2371418110872865193, 0.2374116888449719631, 0.2379514443603428231, 0.2390309553910846263, 0.2411899774525681217, 0.2455080215755351125, 0.2541441098214691219, 0.2714162863133370851, 0.2886884628052050483, 0.2973245510511390299, 0.3016425951741060207, 0.3038016172355895161, 0.3048811282663312361, 0.3054208837817021238, 0.3056907615393875677, 0.3058257004182302619, 0.3058931698576516367, 0.3059269045773623241, 0.3059606392970730115, 0.3060023410584323811, 0.3060440428197917506, 0.3061274463425105452, 0.3062942533879481344, 0.3066278674788231462, 0.3072950956605732808, 0.3086295520240735502, 0.3112984647510740888, 0.3166362902050752215, 0.3273119411130774314, 0.3486632429290818513, 0.3913658465610906356, 0.4767710538251083152, 0.5621762610891259948, 0.6048788647211348346, 0.6262301665371391435, 0.6369058174451412979, 0.6422436428991423751, 0.6449125556261429137, 0.6462470119896432941, 0.6469142401713934287, 0.6472478542622684961, 0.6474146613077059742, 0.6474980648304248243, 0.6475397665917842493, 0.6475814683531435634, 0.6476196945210076494, 0.6476579206888718465, 0.6477343730246000186, 0.6478872776960563629, 0.6481930870389690513, 0.6488047057247944283, 0.6500279430964454042, 0.6524744178397472449, 0.6573673673263507045, 0.6671532662995575125, 0.6769391652727646536, 0.6867250642459716836, 0.6965109632191786027, 0.7062968621923857437, 0.7160827611655926628, 0.7209757106521960113, 0.7234221853954977410, 0.7246454227671487169, 0.7252570414529740939, 0.7255628507958867823, 0.7257157554673431266, 0.7257922078030714097, 0.7258304339709356068, 0.7258686601387995818, 0.7259088784260314675, 0.7259490967132631312, 0.7260295332877264585, 0.7261904064366531131, 0.7265121527345066443, 0.7271556453302134848, 0.7284426305216270547, 0.7310166009044546387, 0.7361645416701096956, 0.7464604232014198093, 0.7670521862640400368 ),
 .UNSPECIFIED. ) ;
#13488=CARTESIAN_POINT ( 'NONE',  ( 24.34695368780276681, -2.542362794815061999, -14.38654857168906886 ) ) ;
#13491=CARTESIAN_POINT ( 'NONE',  ( 26.40146419187390947, -13.39824708621661919, -13.49681364666919059 ) ) ;
#13493=CARTESIAN_POINT ( 'NONE',  ( 27.66237087416717699, -12.37519551434573017, -14.68082181149132204 ) ) ;
#13505=CARTESIAN_POINT ( 'NONE',  ( 9.641350810849047548, 17.66889113945805789, -17.92279151347709032 ) ) ;
#13506=CARTESIAN_POINT ( 'NONE',  ( 24.47745745569867637, -8.908941985067972524, -13.71056886683244258 ) ) ;
#13507=CARTESIAN_POINT ( 'NONE',  ( 18.72775033408030154, 1.433941090885695768, -19.03071139844121262 ) ) ;
#13509=CARTESIAN_POINT ( 'NONE',  ( 36.54859390953724585, -22.18451583373416014, -17.22552805718784441 ) ) ;
#13512=CARTESIAN_POINT ( 'NONE',  ( 11.77869587587188249, 8.711114196793760200, -15.67004689359726299 ) ) ;
#13515=CARTESIAN_POINT ( 'NONE',  ( 9.664154528927689114, 16.24440939496457403, -17.89215119606715021 ) ) ;
#13518=CARTESIAN_POINT ( 'NONE',  ( 16.84948243412402036, 10.49281628697410262, -11.66356073909478575 ) ) ;
#13529=CARTESIAN_POINT ( 'NONE',  ( 8.944584683310379702, 16.95159276115599667, -17.91928203681695564 ) ) ;
#13530=CARTESIAN_POINT ( 'NONE',  ( 33.88611015167484197, -15.71585695178754882, -20.89774115172086510 ) ) ;
#13531=CARTESIAN_POINT ( 'NONE',  ( 19.21851095677833499, -0.002285697959038230937, -14.55609667925758544 ) ) ;
#13532=CARTESIAN_POINT ( 'NONE',  ( 18.54021783837685433, 9.946222303842617407, -15.54065090179396336 ) ) ;
#13535=CARTESIAN_POINT ( 'NONE',  ( 20.25494212361869728, -4.857969563408182090, -14.64469595162225701 ) ) ;
#13544=CARTESIAN_POINT ( 'NONE',  ( 34.16485483951214519, -11.28898102658429536, -18.35413676833350038 ) ) ;
#13546=CARTESIAN_POINT ( 'NONE',  ( 10.90022735844294388, 8.411956631741958290, -16.28271526948893921 ) ) ;
#13551=CARTESIAN_POINT ( 'NONE',  ( 10.48009811366078381, 16.41514476298091907, -17.33146409796769660 ) ) ;
#13567=CARTESIAN_POINT ( 'NONE',  ( 9.661883061612440926, 16.25482663361732705, -23.00000000000000711 ) ) ;
#13568=CARTESIAN_POINT ( 'NONE',  ( 20.98456156242603754, -1.805893270886621327, -19.41059277335735089 ) ) ;
#13569=CARTESIAN_POINT ( 'NONE',  ( 19.97442599234820193, -2.778558858265142373, -17.76606689721253574 ) ) ;
#13571=CARTESIAN_POINT ( 'NONE',  ( 16.54288150113237066, 3.399532473721276649, -19.15960874834559746 ) ) ;
#13574=CARTESIAN_POINT ( 'NONE',  ( 21.63873165585565417, 2.424707942738766331, -13.54651715722292060 ) ) ;
#13582=CARTESIAN_POINT ( 'NONE',  ( 10.35864918915110877, 16.97212501191939538, -17.97192418671891190 ) ) ;
#13589=CARTESIAN_POINT ( 'NONE',  ( 17.54642605795894994, 9.676486402519270058, -18.74681543856335608 ) ) ;
#13590=CARTESIAN_POINT ( 'NONE',  ( 11.05541531668977662, 17.68942339022145305, -17.91928203681695564 ) ) ;
#13591=CARTESIAN_POINT ( 'NONE',  ( 34.96805304670973413, -19.57645325810014114, -20.18246498508359466 ) ) ;
#13595=CARTESIAN_POINT ( 'NONE',  ( 12.75811015101040446, 7.626735917299793499, -14.92445666636202617 ) ) ;
#13600=CARTESIAN_POINT ( 'NONE',  ( 12.87691298531170148, 9.519861518574414205, -16.10853261994384411 ) ) ;
#13601=CARTESIAN_POINT ( 'NONE',  ( 34.33515578781254618, -12.24072284059296933, -19.92088757525016973 ) ) ;
#13602=CARTESIAN_POINT ( 'NONE',  ( 27.91615220763155847, -6.225400021157185826, -17.67258836524805332 ) ) ;
#13606=CARTESIAN_POINT ( 'NONE',  ( 24.40455984355908114, -10.10244183743681035, -17.68366952546245585 ) ) ;
#13607=CARTESIAN_POINT ( 'NONE',  ( 25.81628275165185116, -0.2054900511636704452, -18.66752024111776009 ) ) ;
#13615=CARTESIAN_POINT ( 'NONE',  ( 12.60945047077962933, 8.619070305187777947, -15.04294105552940231 ) ) ;
#13617=CARTESIAN_POINT ( 'NONE',  ( 28.92040988821396752, -12.03996551347764132, -12.87516188627701474 ) ) ;
#13621=CARTESIAN_POINT ( 'NONE',  ( 9.641404825192898542, 17.66864342279195199, -17.88841768828662282 ) ) ;
#13622=CARTESIAN_POINT ( 'NONE',  ( 17.24236049518817282, 9.271217979531970244, -15.28210331290996571 ) ) ;
#13625=CARTESIAN_POINT ( 'NONE',  ( 25.73595588610537277, -4.826321120321507507, -18.84379041344559269 ) ) ;
#13629=CARTESIAN_POINT ( 'NONE',  ( 11.05541531668977662, 17.68942339022145305, -17.92454625180715411 ) ) ;
#13631=CARTESIAN_POINT ( 'NONE',  ( 35.53434814243864537, -22.12051714835155281, -18.84852710552948096 ) ) ;
#13635=CARTESIAN_POINT ( 'NONE',  ( 26.72610680620850232, -7.491537437428757329, -18.63066883040512067 ) ) ;
#13637=CARTESIAN_POINT ( 'NONE',  ( 23.66523006742493251, -0.7244823556979478330, -15.35173719993635011 ) ) ;
#13642=CARTESIAN_POINT ( 'NONE',  ( 14.59671049609067950, 6.266606045730605423, -20.00302036566705155 ) ) ;
#13643=CARTESIAN_POINT ( 'NONE',  ( 25.27233071153842303, -10.58027458246514207, -17.53878701932553952 ) ) ;
#13659=CARTESIAN_POINT ( 'NONE',  ( 25.54411345550068191, -6.057473962578058035, -19.57277538061955013 ) ) ;
#13660=CARTESIAN_POINT ( 'NONE',  ( 16.05281274719596496, 2.901206577426825639, -17.92093306952238407 ) ) ;
#13661=CARTESIAN_POINT ( 'NONE',  ( 32.76003276007612186, -9.647047962658168885, -18.46200315532429315 ) ) ;
#13664=CARTESIAN_POINT ( 'NONE',  ( 11.47181023233108021, 9.274170903235749108, -15.86135313853478657 ) ) ;
#13667=CARTESIAN_POINT ( 'NONE',  ( 9.829968513350019421, 15.48396532603707421, -17.81804186139787660 ) ) ;
#13671=CARTESIAN_POINT ( 'NONE',  ( 11.69419402147360110, 8.800013620902292999, -15.72776802682527730 ) ) ;
#13675=CARTESIAN_POINT ( 'NONE',  ( 15.73644607668725826, 9.740111719757674535, -14.94734896276200153 ) ) ;
#13678=CARTESIAN_POINT ( 'NONE',  ( 9.105507159292685060, 16.21358177345661389, -17.05825009255364932 ) ) ;
#13679=CARTESIAN_POINT ( 'NONE',  ( 33.52946124453396237, -14.11362233419136381, -20.78993474304632372 ) ) ;
#13681=CARTESIAN_POINT ( 'NONE',  ( 20.08305308227469510, 0.3843232119764288246, -14.09874237319206358 ) ) ;
#13683=CARTESIAN_POINT ( 'NONE',  ( 16.80936620776159884, 5.784822248606665163, -14.58992565756060245 ) ) ;
#13685=CARTESIAN_POINT ( 'NONE',  ( 24.74990718239607546, -5.907774739380937667, -20.30682099139976060 ) ) ;
#13689=SURFACE_SIDE_STYLE ('',( #8806 ) ) ;
#13698=CARTESIAN_POINT ( 'NONE',  ( 35.54859306210901337, -21.18451202668684985, -18.38798429269037271 ) ) ;
#13700=CARTESIAN_POINT ( 'NONE',  ( 10.67100603215144794, 9.034109945373653972, -16.41023209856668785 ) ) ;
#13702=CARTESIAN_POINT ( 'NONE',  ( 27.76312469413510442, -10.32446017237915648, -18.80420148706337358 ) ) ;
#13704=CARTESIAN_POINT ( 'NONE',  ( 10.47184394332236224, 16.45299944031493311, -17.33487789703667303 ) ) ;
#13709=CARTESIAN_POINT ( 'NONE',  ( 12.50140887008201851, 8.571324787501421127, -15.12905211845398412 ) ) ;
#13713=CARTESIAN_POINT ( 'NONE',  ( 9.708396314890595846, 16.04151092502291931, -17.86831624201546020 ) ) ;
#13714=CARTESIAN_POINT ( 'NONE',  ( 23.24226111988221888, -3.343277867803439829, -18.62279721135557509 ) ) ;
#13715=CARTESIAN_POINT ( 'NONE',  ( 20.60316120045176902, -2.756227665500133206, -14.85995437523845553 ) ) ;
#13716=CARTESIAN_POINT ( 'NONE',  ( 22.47820520476076567, 2.340993144345510313, -15.49451772223075707 ) ) ;
#13720=CARTESIAN_POINT ( 'NONE',  ( 19.83745040964868522, -2.306422872736943575, -14.39351019504378293 ) ) ;
#13727=CARTESIAN_POINT ( 'NONE',  ( 10.35864918915110877, 16.97212501191939538, -17.95086732675817132 ) ) ;
#13728=CARTESIAN_POINT ( 'NONE',  ( 35.22227017426903473, -20.71851614966110233, -20.19360243392694088 ) ) ;
#13734=CARTESIAN_POINT ( 'NONE',  ( 15.54217852991911997, 3.796156774867226247, -18.16774540469225485 ) ) ;
#13735=CARTESIAN_POINT ( 'NONE',  ( 11.23925813788225447, 16.84629677772421275, -16.81283633444384407 ) ) ;
#13736=CARTESIAN_POINT ( 'NONE',  ( 35.13870703111577143, -20.34311121210408757, -20.23074448643712486 ) ) ;
#13737=ORIENTED_EDGE ( 'NONE', *, *, #28410, .T. ) ;
#13739=CARTESIAN_POINT ( 'NONE',  ( 9.641485839925177714, 17.66827187890266160, -17.87200850766020110 ) ) ;
#13740=CARTESIAN_POINT ( 'NONE',  ( 14.64119204185053391, 8.458903494591371697, -13.42360716063767967 ) ) ;
#13746=CARTESIAN_POINT ( 'NONE',  ( 10.47212132250356120, 16.45172734403231729, -17.33476278219207956 ) ) ;
#13747=CARTESIAN_POINT ( 'NONE',  ( 34.35798975979065517, -12.34328324435382207, -19.92780167937219815 ) ) ;
#13748=CARTESIAN_POINT ( 'NONE',  ( 26.72181814967143509, -3.137724904577397389, -15.69709663067708050 ) ) ;
#13752=CARTESIAN_POINT ( 'NONE',  ( 14.86918570794847305, 4.945381287188965302, -16.48322999939953704 ) ) ;
#13753=CARTESIAN_POINT ( 'NONE',  ( 26.42757832573366983, -5.232593867482060013, -19.46531670327460617 ) ) ;
#13763=CARTESIAN_POINT ( 'NONE',  ( 10.80186837770346919, 16.25936630249904269, -15.92067135797631217 ) ) ;
#13764=CARTESIAN_POINT ( 'NONE',  ( 26.35635630057183576, -13.06715036242849948, -16.03892985609963873 ) ) ;
#13768=CARTESIAN_POINT ( 'NONE',  ( 10.56508425215480074, 13.43253182900300402, -16.23631622730588830 ) ) ;
#13770=CARTESIAN_POINT ( 'NONE',  ( 18.33619432801213023, 6.228962682262685568, -18.83744168170139233 ) ) ;
#13773=CARTESIAN_POINT ( 'NONE',  ( 27.26129135193747999, -10.77754955263135095, -18.64424489656416739 ) ) ;
#13777=CARTESIAN_POINT ( 'NONE',  ( 12.24519447470441413, 9.516128708456710328, -15.33325952276184445 ) ) ;
#13779=CARTESIAN_POINT ( 'NONE',  ( 33.35202879388211983, -12.33251541790028760, -19.68467382345759376 ) ) ;
#13783=CARTESIAN_POINT ( 'NONE',  ( 22.42041779846375604, -0.009017426515379003624, -18.82878497401882001 ) ) ;
#13787=CARTESIAN_POINT ( 'NONE',  ( 26.29067154119281824, -12.76617647537077538, -18.64558906701574514 ) ) ;
#13788=CARTESIAN_POINT ( 'NONE',  ( 26.40217035250003974, -9.511505991202637844, -18.98702918838447573 ) ) ;
#13789=ORIENTED_EDGE ( 'NONE', *, *, #28410, .F. ) ;
#13796=CARTESIAN_POINT ( 'NONE',  ( 9.745779815811758340, 17.18996641109745482, -16.82979807527155458 ) ) ;
#13797=CARTESIAN_POINT ( 'NONE',  ( 24.72855373928933531, -1.476844508782828802, -20.15487193605729033 ) ) ;
#13798=CARTESIAN_POINT ( 'NONE',  ( 15.02162844583664736, 5.759011576665847620, -14.59661587647459591 ) ) ;
#13799=CARTESIAN_POINT ( 'NONE',  ( 36.54859390953724585, -23.18451583373416014, -18.19919658220850422 ) ) ;
#13801=CARTESIAN_POINT ( 'NONE',  ( 12.23783994716398560, 8.515526397163364791, -15.33449341356891615 ) ) ;
#13804=CARTESIAN_POINT ( 'NONE',  ( 17.32873655921053313, 10.26331207550778579, -16.20725374984683143 ) ) ;
#13807=CARTESIAN_POINT ( 'NONE',  ( 12.50906579366657390, 8.574708520419219937, -15.12294941509656354 ) ) ;
#13811=CARTESIAN_POINT ( 'NONE',  ( 15.54217852991911997, 3.796156774867226247, -18.16774540469225485 ) ) ;
#13815=CARTESIAN_POINT ( 'NONE',  ( 9.122709158550120989, 16.13469121211704049, -17.05051537109504523 ) ) ;
#13816=CARTESIAN_POINT ( 'NONE',  ( 35.54859390953724585, -23.18451583373416014, -16.94733705004010105 ) ) ;
#13819=CARTESIAN_POINT ( 'NONE',  ( 20.91577097522866424, 8.170114823437694795, -18.25116917207579093 ) ) ;
#13821=CARTESIAN_POINT ( 'NONE',  ( 29.95311431238071975, -11.57681909846818691, -12.96816900313696230 ) ) ;
#13825=CARTESIAN_POINT ( 'NONE',  ( 22.08361411416106534, -2.618483922437499611, -20.46533185456077319 ) ) ;
#13834=CARTESIAN_POINT ( 'NONE',  ( 36.54859390953724585, -21.18451583373416014, -16.11276402859391510 ) ) ;
#13835=CARTESIAN_POINT ( 'NONE',  ( 12.69188586677704400, 7.599409645471840058, -14.97709067247704340 ) ) ;
#13839=CARTESIAN_POINT ( 'NONE',  ( 10.51251736658329961, 16.26646593658467310, -17.31805759646961462 ) ) ;
#13848=CARTESIAN_POINT ( 'NONE',  ( 9.678003265275730627, 16.18089732476941833, -17.88088483716984811 ) ) ;
#13850=CARTESIAN_POINT ( 'NONE',  ( 24.16235420939608858, 2.058193855977920261, -15.89352170542055198 ) ) ;
#13851=CARTESIAN_POINT ( 'NONE',  ( 21.88384027766407414, -2.187040905716116868, -14.00385029740408704 ) ) ;
#13855=CARTESIAN_POINT ( 'NONE',  ( 21.50147616854745891, 4.214167280306792662, -18.19698480873994839 ) ) ;
#13861=CARTESIAN_POINT ( 'NONE',  ( 21.18945582756405344, -5.194394521544061227, -16.21196392551894405 ) ) ;
#13868=CARTESIAN_POINT ( 'NONE',  ( 10.35864918915110877, 16.97212501191939538, -17.92981046679734547 ) ) ;
#13869=CARTESIAN_POINT ( 'NONE',  ( 35.54859215833182873, -22.18450796649496226, -18.40462262104107083 ) ) ;
#13872=CARTESIAN_POINT ( 'NONE',  ( 11.22197018571015725, 9.100068217651248403, -17.24240020332717904 ) ) ;
#13876=CARTESIAN_POINT ( 'NONE',  ( 19.25770813156441008, -2.543370271471735222, -15.40753146551623587 ) ) ;
#13877=CARTESIAN_POINT ( 'NONE',  ( 11.27605965875426541, 16.67752031190189399, -16.78457976421582742 ) ) ;
#13878=CARTESIAN_POINT ( 'NONE',  ( 34.39741479528305490, -17.01287786994462792, -20.00997473120332515 ) ) ;
#13880=CARTESIAN_POINT ( 'NONE',  ( 9.916411867603999397, 16.40742607105030260, -16.50456570466356965 ) ) ;
#13881=CARTESIAN_POINT ( 'NONE',  ( 9.641350810849047548, 17.66889113945805789, -17.94384837343789485 ) ) ;
#13887=CARTESIAN_POINT ( 'NONE',  ( 10.46436961932593945, 16.48727764291732711, -17.33901581970886241 ) ) ;
#13889=CARTESIAN_POINT ( 'NONE',  ( 36.54645402898028550, -21.17490248391822050, -18.49223762587710951 ) ) ;
#13890=CARTESIAN_POINT ( 'NONE',  ( 25.07290406138036687, -9.006318079059196791, -17.79994936451110732 ) ) ;
#13898=CARTESIAN_POINT ( 'NONE',  ( 16.70639138691818459, 6.939553047386250562, -20.38695695975560085 ) ) ;
#13899=CARTESIAN_POINT ( 'NONE',  ( 29.29611939376944107, -10.57052713796966081, -13.72407686852593400 ) ) ;
#13908=CARTESIAN_POINT ( 'NONE',  ( 10.52543090623380451, 17.52714378424053265, -16.25779133722369707 ) ) ;
#13913=CARTESIAN_POINT ( 'NONE',  ( 9.949118446627077006, 16.25742953053141804, -16.49103975576934644 ) ) ;
#13915=CARTESIAN_POINT ( 'NONE',  ( 15.53255613197921647, 5.987779765840379298, -16.04456276566740058 ) ) ;
#13918=CARTESIAN_POINT ( 'NONE',  ( 31.81434894052502571, -10.04473835610349397, -15.03854332269495764 ) ) ;
#13922=CARTESIAN_POINT ( 'NONE',  ( 11.29232397858413250, 16.60293006794363535, -16.77785382704750461 ) ) ;
#13923=CARTESIAN_POINT ( 'NONE',  ( 35.54859390953724585, -22.18451583373416014, -16.94733705004010460 ) ) ;
#13927=CARTESIAN_POINT ( 'NONE',  ( 23.29143545295710638, -10.05536756138072718, -15.72373794962660831 ) ) ;
#13932=CARTESIAN_POINT ( 'NONE',  ( 18.12654306171327079, 0.8625984663607378922, -18.09208126113620452 ) ) ;
#13933=CARTESIAN_POINT ( 'NONE',  ( 27.51083730600015897, -9.905735641176994122, -13.30399992039142099 ) ) ;
#13942=CARTESIAN_POINT ( 'NONE',  ( 9.917015787971365626, 16.40465641526357743, -16.50431533440121257 ) ) ;
#13943=CARTESIAN_POINT ( 'NONE',  ( 23.94974919959990345, -8.117095362258064384, -14.41405346848900848 ) ) ;
#13944=CARTESIAN_POINT ( 'NONE',  ( 20.05514754915220266, -1.452567280579552866, -14.87399747198034738 ) ) ;
#13946=CARTESIAN_POINT ( 'NONE',  ( 36.40320260674921116, -22.53134972621836241, -20.30234751949853589 ) ) ;
#13948=CARTESIAN_POINT ( 'NONE',  ( 12.52778158092594474, 8.582979361647906202, -15.10803260229456946 ) ) ;
#13955=CARTESIAN_POINT ( 'NONE',  ( 10.72588575366639674, 16.60783230186494563, -15.95209284586258214 ) ) ;
#13961=CARTESIAN_POINT ( 'NONE',  ( 18.47369133221681281, 7.987600538477567014, -15.27093437040897861 ) ) ;
#13964=CARTESIAN_POINT ( 'NONE',  ( 35.54859390953724585, -23.18451583373416014, -17.22552805718784441 ) ) ;
#13965=CARTESIAN_POINT ( 'NONE',  ( 24.85091453934022709, -2.360935040140837771, -14.69038261433388293 ) ) ;
#13966=CARTESIAN_POINT ( 'NONE',  ( 28.92040988821396752, -12.03996551347764132, -12.87516188627701474 ) ) ;
#13967=CARTESIAN_POINT ( 'NONE',  ( 27.03394943597420408, -2.104382873295748801, -14.19367964525161163 ) ) ;
#13978=CARTESIAN_POINT ( 'NONE',  ( 36.54859390953724585, -21.18451583373416014, -17.78191007148576119 ) ) ;
#13979=CARTESIAN_POINT ( 'NONE',  ( 9.641359250860388030, 17.66885243249017634, -17.90483003768722625 ) ) ;
#13985=CARTESIAN_POINT ( 'NONE',  ( 10.47079889355419446, 16.45779217176459852, -17.33533584583738829 ) ) ;
#13995=CARTESIAN_POINT ( 'NONE',  ( 9.667904883771802460, 16.22720978959070592, -17.88506087084571305 ) ) ;
#13997=CARTESIAN_POINT ( 'NONE',  ( 25.76085037594245719, -3.206535967183471669, -15.98314152415894540 ) ) ;
#13998=CARTESIAN_POINT ( 'NONE',  ( 24.16216977846044145, 1.369666316211566093, -18.31128106405367006 ) ) ;
#13999=CARTESIAN_POINT ( 'NONE',  ( 16.63724033897865340, 2.930722838386041751, -15.17604395537502526 ) ) ;
#14002=DIRECTION ( 'NONE',  ( 1.949100835863659470E-16, -2.773645458326357876E-16, -1.000000000000000000 ) ) ;
#14003=CARTESIAN_POINT ( 'NONE',  ( 24.81358459371387326, -5.676498915796258871, -18.90393244824272756 ) ) ;
#14010=CARTESIAN_POINT ( 'NONE',  ( 10.35866308580767026, 16.97206128008099313, -17.90676409391864610 ) ) ;
#14017=CARTESIAN_POINT ( 'NONE',  ( 11.23996880139866761, 9.021883543159612273, -17.23462466665071346 ) ) ;
#14022=CARTESIAN_POINT ( 'NONE',  ( 17.72480397827495224, 1.356124466512965476, -19.40231245121514903 ) ) ;
#14023=CARTESIAN_POINT ( 'NONE',  ( 11.30853360504539751, 16.52859065474556033, -16.77115057629831441 ) ) ;
#14028=CARTESIAN_POINT ( 'NONE',  ( 9.917712295358372288, 16.40146214360271770, -16.50402730409559027 ) ) ;
#14030=CARTESIAN_POINT ( 'NONE',  ( 9.981537699549546616, 16.10875070413535681, -16.47763325427154868 ) ) ;
#14036=CARTESIAN_POINT ( 'NONE',  ( 10.47300640208398370, 16.44766825625507778, -17.33439677017039671 ) ) ;
#14038=CARTESIAN_POINT ( 'NONE',  ( 36.54859390953723874, -22.18451583373416014, -15.00000000000000000 ) ) ;
#14039=CARTESIAN_POINT ( 'NONE',  ( 26.72610680620850232, -7.491537437428757329, -18.63066883040512067 ) ) ;
#14042=CARTESIAN_POINT ( 'NONE',  ( 32.71419323209526908, -10.28616775856061416, -16.33292762241428520 ) ) ;
#14044=CARTESIAN_POINT ( 'NONE',  ( 18.54021783837685433, 9.946222303842617407, -15.54065090179396336 ) ) ;
#14046=CARTESIAN_POINT ( 'NONE',  ( 26.06970682676011464, -9.363093171025507644, -17.79562309782675911 ) ) ;
#14058=CARTESIAN_POINT ( 'NONE',  ( 10.59516011209494302, 17.20735675775515361, -16.09619895116188815 ) ) ;
#14065=CARTESIAN_POINT ( 'NONE',  ( 9.932908820165812003, 16.33176894372950727, -16.49774300651844072 ) ) ;
#14066=CARTESIAN_POINT ( 'NONE',  ( 30.58694070296994028, -11.15840821071237698, -14.58880109071565556 ) ) ;
#14069=CARTESIAN_POINT ( 'NONE',  ( 26.36224721256908410, -8.875037662531589433, -13.49479840426202948 ) ) ;
#14073=CARTESIAN_POINT ( 'NONE',  ( 11.05714535396004727, 17.68148921877153157, -17.77574279453144968 ) ) ;
#14075=CARTESIAN_POINT ( 'NONE',  ( 33.91010249890941708, -13.82364185882242147, -18.82035036639317482 ) ) ;
#14076=CARTESIAN_POINT ( 'NONE',  ( 17.69365662292968366, 10.27476822432933545, -17.01437286930526227 ) ) ;
#14078=CARTESIAN_POINT ( 'NONE',  ( 28.21504805113574221, -4.147720155524260655, -15.34900075604336500 ) ) ;
#14081=CARTESIAN_POINT ( 'NONE',  ( 19.14470263920462401, 1.819183656627200829, -19.33730474122706866 ) ) ;
#14082=CARTESIAN_POINT ( 'NONE',  ( 16.42791133306356599, 6.383902638027607601, -15.35376453018263199 ) ) ;
#14094=CARTESIAN_POINT ( 'NONE',  ( 9.843778300897430000, 16.74053286659246709, -16.57516421589427225 ) ) ;
#14096=CARTESIAN_POINT ( 'NONE',  ( 25.25929662509423324, 0.6462067467026075818, -14.45468018858982795 ) ) ;
#14097=CARTESIAN_POINT ( 'NONE',  ( 23.93603600111211804, 0.1510904554606163908, -14.93755387302875448 ) ) ;
#14098=CARTESIAN_POINT ( 'NONE',  ( 36.54859390953724585, -23.18451583373416014, -16.11276402859391510 ) ) ;
#14104=CARTESIAN_POINT ( 'NONE',  ( 16.53342136567307108, 10.04554801986687629, -15.32032680638607047 ) ) ;
#14108=CARTESIAN_POINT ( 'NONE',  ( 10.34291491886349235, 18.36418536769788901, -17.61263766090776528 ) ) ;
#14114=CARTESIAN_POINT ( 'NONE',  ( 19.23836061553175369, 5.151828676608854352, -13.99136221198299168 ) ) ;
#14117=CARTESIAN_POINT ( 'NONE',  ( 29.49229018507869071, -8.391778287988243434, -19.20830874944899236 ) ) ;
#14120=CARTESIAN_POINT ( 'NONE',  ( 34.59940796595157053, -18.92032618698594248, -21.11335396907232465 ) ) ;
#14121=CARTESIAN_POINT ( 'NONE',  ( 22.82249278870453679, 0.4072072893072278821, -18.57859108775207702 ) ) ;
#14122=CARTESIAN_POINT ( 'NONE',  ( 20.54317392443767076, 4.330699614500605144, -17.92201748610454715 ) ) ;
#14124=CARTESIAN_POINT ( 'NONE',  ( 25.33177305468611351, -7.180647579645999201, -12.45679661262278870 ) ) ;
#14136=CARTESIAN_POINT ( 'NONE',  ( 34.61906131182126245, -12.51614797404085877, -18.96439083239160439 ) ) ;
#14137=CARTESIAN_POINT ( 'NONE',  ( 9.641350810849047548, 17.66889113945805789, -17.93331994345748370 ) ) ;
#14141=CARTESIAN_POINT ( 'NONE',  ( 10.47325967749744180, 16.44650670292386607, -17.33429203187744250 ) ) ;
#14153=CARTESIAN_POINT ( 'NONE',  ( 10.18658029549746935, 13.84849823568026217, -17.67057034492011525 ) ) ;
#14155=CARTESIAN_POINT ( 'NONE',  ( 23.80376867147650444, -3.845223433682474212, -14.48388124448521452 ) ) ;
#14156=CARTESIAN_POINT ( 'NONE',  ( 16.00562779705659011, 2.776126820729137190, -17.20623408552720690 ) ) ;
#14161=CARTESIAN_POINT ( 'NONE',  ( 21.16681283796276603, -5.103637247178538061, -17.00692323485822754 ) ) ;
#14168=CARTESIAN_POINT ( 'NONE',  ( 10.47604570704546845, 16.43372961628045559, -17.33313991065496751 ) ) ;
#14169=CARTESIAN_POINT ( 'NONE',  ( 35.54859390953724585, -22.18451583373416014, -17.78191007148576475 ) ) ;
#14170=STYLED_ITEM ( 'NONE', ( #1922 ), #15681 ) ;
#14172=CARTESIAN_POINT ( 'NONE',  ( 8.944584683310379702, 16.95159276115599667, -23.00000000000000711 ) ) ;
#14175=CARTESIAN_POINT ( 'NONE',  ( 18.34549112274340033, 0.9605221043122941227, -13.99314825615798341 ) ) ;
#14176=CARTESIAN_POINT ( 'NONE',  ( 11.27599706080618525, 16.67780739407118062, -16.78460567626121502 ) ) ;
#14180=CARTESIAN_POINT ( 'NONE',  ( 9.641350829061996919, 17.66889105593114806, -17.91548090047172437 ) ) ;
#14182=CARTESIAN_POINT ( 'NONE',  ( 9.898178882064430084, 16.49104486689975246, -16.51464960819000893 ) ) ;
#14188=CARTESIAN_POINT ( 'NONE',  ( 10.45680941692980959, 16.52194969480735764, -17.34528143170414083 ) ) ;
#14191=CARTESIAN_POINT ( 'NONE',  ( 33.21349783521664278, -10.00660656636812007, -19.57461044683394746 ) ) ;
#14193=CARTESIAN_POINT ( 'NONE',  ( 25.79824969357368047, -12.24460132778619226, -15.92960863319586906 ) ) ;
#14194=CARTESIAN_POINT ( 'NONE',  ( 23.11440248821028831, -7.346120041196752659, -16.32852059634029018 ) ) ;
#14198=CARTESIAN_POINT ( 'NONE',  ( 33.49783966318349115, -10.45910432307822902, -18.51641766868578287 ) ) ;
#14202=CARTESIAN_POINT ( 'NONE',  ( 19.26077778332419044, 5.765437233969479713, -18.81236659294151892 ) ) ;
#14204=CARTESIAN_POINT ( 'NONE',  ( 14.93287775521291394, 9.378568215907955974, -14.88591063491414168 ) ) ;
#14211=CARTESIAN_POINT ( 'NONE',  ( 10.75323949831978432, 16.48238454209313630, -15.94078111022350619 ) ) ;
#14216=CARTESIAN_POINT ( 'NONE',  ( 11.43229926783177497, 9.455373222906182207, -15.87769231223556332 ) ) ;
#14217=CARTESIAN_POINT ( 'NONE',  ( 10.57561133056755942, 12.06435231892607618, -17.50969232694400546 ) ) ;
#14218=CARTESIAN_POINT ( 'NONE',  ( 20.59810038911313157, 5.339108984243529754, -18.13170489685289510 ) ) ;
#14221=CARTESIAN_POINT ( 'NONE',  ( 25.90632082398269276, -12.28056132945115841, -15.12647891527467969 ) ) ;
#14223=CARTESIAN_POINT ( 'NONE',  ( 11.05541599318665469, 17.68942028772053376, -17.91303167831651422 ) ) ;
#14225=CARTESIAN_POINT ( 'NONE',  ( 35.39068211221506743, -20.47510177656754493, -19.23609803736608725 ) ) ;
#14229=CARTESIAN_POINT ( 'NONE',  ( 29.43474752111978177, -7.508961153211615169, -12.65842848261850229 ) ) ;
#14233=CARTESIAN_POINT ( 'NONE',  ( 22.61876936045522513, 2.364863857962155258, -15.74433402521326819 ) ) ;
#14234=CARTESIAN_POINT ( 'NONE',  ( 16.22630451241072436, 4.170241327582352220, -17.06284370071109535 ) ) ;
#14246=CARTESIAN_POINT ( 'NONE',  ( 9.641485839925177714, 17.66827187890266160, -17.87200850766020110 ) ) ;
#14247=CARTESIAN_POINT ( 'NONE',  ( 18.07093408371026300, -2.157424655934858215, -16.53044640867639359 ) ) ;
#14248=CARTESIAN_POINT ( 'NONE',  ( 18.97628335640213493, 0.9430780577607489334, -14.77698032187241850 ) ) ;
#14249=CARTESIAN_POINT ( 'NONE',  ( 36.54859390953724585, -23.18451583373416014, -17.64281456791166391 ) ) ;
#14255=CARTESIAN_POINT ( 'NONE',  ( 18.76632379254337835, 6.868107169226369102, -19.55161205380106892 ) ) ;
#14257=CARTESIAN_POINT ( 'NONE',  ( 10.33811689237846743, 18.38618972876440338, -17.91642382710546855 ) ) ;
#14262=CARTESIAN_POINT ( 'NONE',  ( 16.09764958744793262, 8.143416238145906760, -19.84970969296679044 ) ) ;
#14264=CARTESIAN_POINT ( 'NONE',  ( 12.86846089198198584, 5.826474397738612865, -17.89591831848172276 ) ) ;
#14266=CARTESIAN_POINT ( 'NONE',  ( 35.12509383387676820, -20.28195432802065312, -20.22992657050740917 ) ) ;
#14267=CARTESIAN_POINT ( 'NONE',  ( 22.60936069168443652, -2.585520780102871896, -18.46111163327002913 ) ) ;
#14269=CARTESIAN_POINT ( 'NONE',  ( 22.11273855634006935, 3.201273238686522138, -15.95510540678940181 ) ) ;
#14274=CARTESIAN_POINT ( 'NONE',  ( 25.16264305761801268, -10.69278474016982727, -17.18274900023375906 ) ) ;
#14281=CARTESIAN_POINT ( 'NONE',  ( 36.25073006198487491, -19.84637134955221072, -19.45760515208133512 ) ) ;
#14282=CARTESIAN_POINT ( 'NONE',  ( 12.75684812230466925, 7.626178201396932366, -14.92546252573342258 ) ) ;
#14286=CARTESIAN_POINT ( 'NONE',  ( 12.02817646543008934, 9.315460371489308500, -16.69127922251917795 ) ) ;
#14299=CARTESIAN_POINT ( 'NONE',  ( 9.667670487869566287, 16.22828475907693146, -17.88517164372263579 ) ) ;
#14300=CARTESIAN_POINT ( 'NONE',  ( 25.68863286643039601, -3.692565893519352827, -17.49701707463368550 ) ) ;
#14301=CARTESIAN_POINT ( 'NONE',  ( 20.49605984403359216, -1.259233478192978373, -14.44550164344372511 ) ) ;
#14306=CARTESIAN_POINT ( 'NONE',  ( 24.95482030053459965, -6.624749414579512496, -13.76522253407564733 ) ) ;
#14313=CARTESIAN_POINT ( 'NONE',  ( 10.47230989469697882, 16.45086252791593751, -17.33468480047602256 ) ) ;
#14315=CARTESIAN_POINT ( 'NONE',  ( 34.54007435814109783, -17.65377171698271752, -20.05309729467257540 ) ) ;
#14317=CARTESIAN_POINT ( 'NONE',  ( 8.944589832665828411, 16.95156914555548866, -17.90909639166975609 ) ) ;
#14320=CARTESIAN_POINT ( 'NONE',  ( 20.24985932600369409, 3.694099309552050237, -20.13309853732883781 ) ) ;
#14321=CARTESIAN_POINT ( 'NONE',  ( 12.83021228909557010, 9.549978240774745331, -16.14188291223562288 ) ) ;
#14326=CARTESIAN_POINT ( 'NONE',  ( 9.641350810849047548, 17.66889113945805789, -17.92279151347709032 ) ) ;
#14329=CARTESIAN_POINT ( 'NONE',  ( 9.932908820165812003, 16.33176894372950727, -16.49774300651844072 ) ) ;
#14334=CARTESIAN_POINT ( 'NONE',  ( 10.35900481074863322, 16.97049408594186914, -17.87076805301065363 ) ) ;
#14336=CARTESIAN_POINT ( 'NONE',  ( 34.03885009341546208, -11.93819216554969742, -20.85700406890413916 ) ) ;
#14337=CARTESIAN_POINT ( 'NONE',  ( 24.60501232743784783, -9.531698448777172317, -16.22453333552994792 ) ) ;
#14338=CARTESIAN_POINT ( 'NONE',  ( 13.73972855572809060, 6.741564148929986011, -15.48174541850189811 ) ) ;
#14342=CARTESIAN_POINT ( 'NONE',  ( 34.70514358766799745, -13.90287004036446739, -20.03273298744158737 ) ) ;
#14343=CARTESIAN_POINT ( 'NONE',  ( 18.31728471214517029, 9.901174664208697962, -15.18855771585127634 ) ) ;
#14344=CARTESIAN_POINT ( 'NONE',  ( 28.95742876386502118, -9.428754790923060014, -17.52548735455339823 ) ) ;
#14354=UNCERTAINTY_MEASURE_WITH_UNIT (LENGTH_MEASURE( 1.000000000000000082E-05 ), #8465, 'distance_accuracy_value', 'NONE');
#14355=CARTESIAN_POINT ( 'NONE',  ( 10.71981169803933120, 16.63568869523268390, -15.95461020916288675 ) ) ;
#14362=CARTESIAN_POINT ( 'NONE',  ( 9.916824447075894611, 16.40553392900050156, -16.50439446175997205 ) ) ;
#14365=CARTESIAN_POINT ( 'NONE',  ( 9.667864356596815867, 16.22739565238121529, -17.88507765419223716 ) ) ;
#14366=CARTESIAN_POINT ( 'NONE',  ( 22.85609869791697335, 3.752015377681134467, -15.55886478590537969 ) ) ;
#14368=CARTESIAN_POINT ( 'NONE',  ( 27.95388715220626707, -5.541385876428546631, -15.41148221666858831 ) ) ;
#14370=CARTESIAN_POINT ( 'NONE',  ( 11.27738072919014911, 16.67146171448561276, -16.78403338633166442 ) ) ;
#14372=CARTESIAN_POINT ( 'NONE',  ( 33.80310782676656345, -13.34297147354166135, -18.78800844379110302 ) ) ;
#14373=CARTESIAN_POINT ( 'NONE',  ( 17.29421355564066332, 9.360779442694735053, -19.18964209290773937 ) ) ;
#14376=CARTESIAN_POINT ( 'NONE',  ( 9.008298112641352162, 16.65939485267133335, -17.25320607661530303 ) ) ;
#14377=CARTESIAN_POINT ( 'NONE',  ( 24.24063474714532873, -9.755679120534059834, -13.19378374426895206 ) ) ;
#14381=CARTESIAN_POINT ( 'NONE',  ( 16.29141254853644227, 2.771581735061156682, -15.76764191790683611 ) ) ;
#14382=CARTESIAN_POINT ( 'NONE',  ( 14.03260640687251204, 7.914523597318124715, -15.18742456358547521 ) ) ;
#14394=CARTESIAN_POINT ( 'NONE',  ( 9.916336358462064737, 16.40777236560037622, -16.50459729666445696 ) ) ;
#14395=CARTESIAN_POINT ( 'NONE',  ( 27.79246359028025992, -7.761574269410560944, -18.12988733074048753 ) ) ;
#14396=CARTESIAN_POINT ( 'NONE',  ( 20.61437924707763258, -4.384239709691692966, -16.09784705243023240 ) ) ;
#14398=CARTESIAN_POINT ( 'NONE',  ( 33.26197456417788345, -12.91194637099222575, -20.70907993653955970 ) ) ;
#14401=CARTESIAN_POINT ( 'NONE',  ( 12.50906579366657390, 8.574708520419219937, -15.12294941509656354 ) ) ;
#14406=CARTESIAN_POINT ( 'NONE',  ( 18.47369133221681281, 7.987600538477567014, -15.27093437040897861 ) ) ;
#14409=CARTESIAN_POINT ( 'NONE',  ( 10.34111691064986438, 18.37243126255838988, -17.67295385331717483 ) ) ;
#14413=CARTESIAN_POINT ( 'NONE',  ( 18.76632379254337835, 6.868107169226369102, -19.55161205380106892 ) ) ;
#14414=CARTESIAN_POINT ( 'NONE',  ( 15.52843720209238931, 6.760224976758691717, -13.32525641785786696 ) ) ;
#14416=CARTESIAN_POINT ( 'NONE',  ( 32.96569147872224903, -11.36116021242123608, -19.12347989294568151 ) ) ;
#14417=CARTESIAN_POINT ( 'NONE',  ( 23.38119176934044674, -2.968156504308268495, -14.25447959695224043 ) ) ;
#14419=CARTESIAN_POINT ( 'NONE',  ( 17.99585798733817299, 1.806717527199089401, -17.78491074480216838 ) ) ;
#14422=CARTESIAN_POINT ( 'NONE',  ( 27.32970014129078962, -12.32490512882196754, -16.69500413328365696 ) ) ;
#14431=CARTESIAN_POINT ( 'NONE',  ( 34.59231264378541937, -12.39598037772099559, -18.95630535174095499 ) ) ;
#14433=CARTESIAN_POINT ( 'NONE',  ( 9.641384570184822422, 17.66873631484086715, -17.89388817125738385 ) ) ;
#14441=CARTESIAN_POINT ( 'NONE',  ( 12.02799090998256304, 9.316311091778235465, -16.69135597610317134 ) ) ;
#14452=CARTESIAN_POINT ( 'NONE',  ( 12.48979292151040177, 7.561326536588189207, -16.39201226339353212 ) ) ;
#14453=CARTESIAN_POINT ( 'NONE',  ( 25.85400256215867643, -3.413040292952954413, -16.90843739280879277 ) ) ;
#14454=CARTESIAN_POINT ( 'NONE',  ( 26.84208138670940968, -2.489200896322508516, -17.35162900556907317 ) ) ;
#14468=CARTESIAN_POINT ( 'NONE',  ( 10.99070134719017311, 14.07345324724201063, -17.12031169937328201 ) ) ;
#14470=CARTESIAN_POINT ( 'NONE',  ( 32.58918748260075660, -11.04229556371213583, -18.21152344180378080 ) ) ;
#14472=CARTESIAN_POINT ( 'NONE',  ( 8.944585005148796952, 16.95159128516397118, -17.91410349795882340 ) ) ;
#14476=CARTESIAN_POINT ( 'NONE',  ( 17.36512755686010934, 0.5347363583120325892, -15.24149349723765390 ) ) ;
#14478=CARTESIAN_POINT ( 'NONE',  ( 12.83866652039362855, 9.525916288823983891, -16.13726486007240624 ) ) ;
#14483=CARTESIAN_POINT ( 'NONE',  ( 11.65548303173490652, 8.849831895876286936, -15.75351705932409985 ) ) ;
#14485=CARTESIAN_POINT ( 'NONE',  ( 11.21346931060482000, 10.45895530107994098, -15.96818619734747458 ) ) ;
#14490=CARTESIAN_POINT ( 'NONE',  ( 12.01798642417223739, 9.362192935812041483, -16.69549318315592856 ) ) ;
#14493=CARTESIAN_POINT ( 'NONE',  ( 36.54222296954648641, -22.15589457513855010, -18.69601260479128513 ) ) ;
#14494=CARTESIAN_POINT ( 'NONE',  ( 16.83828815103352028, 11.11029360287396983, -16.41243972054167344 ) ) ;
#14495=CARTESIAN_POINT ( 'NONE',  ( 29.66490191837812773, -8.365349891895018430, -17.62461620872172574 ) ) ;
#14498=CARTESIAN_POINT ( 'NONE',  ( 34.27125395597954594, -11.98684039141630819, -19.88226891060491752 ) ) ;
#14500=CARTESIAN_POINT ( 'NONE',  ( 20.25556019283287768, 3.967930604842117681, -18.44304694949289569 ) ) ;
#14501=CARTESIAN_POINT ( 'NONE',  ( 28.61166709039449785, -6.781025521995295513, -16.93684798036101213 ) ) ;
#14511=CARTESIAN_POINT ( 'NONE',  ( 12.25326555804286421, 9.517817489571868350, -15.32696995758615621 ) ) ;
#14515=CARTESIAN_POINT ( 'NONE',  ( 12.50035968906703765, 8.570861208087439564, -15.12988832871674560 ) ) ;
#14518=CARTESIAN_POINT ( 'NONE',  ( 18.16797961131436523, 4.950584380424773556, -14.83967967756414730 ) ) ;
#14524=CARTESIAN_POINT ( 'NONE',  ( 11.06643561541932463, 17.63888289548684796, -17.56974948598543662 ) ) ;
#14527=CARTESIAN_POINT ( 'NONE',  ( 35.54824714876834690, -21.18295802128256611, -18.40066978570660083 ) ) ;
#14528=CARTESIAN_POINT ( 'NONE',  ( 18.55171814111300321, 6.637122934506423988, -19.73184648383247364 ) ) ;
#14530=CARTESIAN_POINT ( 'NONE',  ( 9.109039160554445402, 16.19738356544468516, -17.05632368146133615 ) ) ;
#14531=CARTESIAN_POINT ( 'NONE',  ( 28.15806058933612022, -5.108324757233392077, -18.51472486207664758 ) ) ;
#14535=CARTESIAN_POINT ( 'NONE',  ( 22.75707610144304383, -3.504958924507949991, -13.40925247317622571 ) ) ;
#14536=CARTESIAN_POINT ( 'NONE',  ( 16.71823672545656336, 7.456161109308904855, -19.47106720222115683 ) ) ;
#14547=CARTESIAN_POINT ( 'NONE',  ( 11.21346931060482000, 10.45895530107994098, -15.96818619734747458 ) ) ;
#14548=AXIS2_PLACEMENT_3D ( 'NONE', #26707, #14910, #3638 ) ;
#14549=CARTESIAN_POINT ( 'NONE',  ( 27.46788175125265141, -10.83975311022233079, -17.61709057740623408 ) ) ;
#14550=CARTESIAN_POINT ( 'NONE',  ( 23.39789874936200320, -0.01207823811560896493, -14.43595595811700782 ) ) ;
#14551=CARTESIAN_POINT ( 'NONE',  ( 32.58918748260075660, -11.04229556371213583, -18.21152344180378080 ) ) ;
#14555=CARTESIAN_POINT ( 'NONE',  ( 12.50162201464318557, 8.571418981294288031, -15.12888223836978341 ) ) ;
#14558=CARTESIAN_POINT ( 'NONE',  ( 20.50636976340433293, -0.9757509181830721356, -19.91080244439677571 ) ) ;
#14561=CARTESIAN_POINT ( 'NONE',  ( 10.59516011209494302, 17.20735675775515361, -16.09619895116188815 ) ) ;
#14564=CARTESIAN_POINT ( 'NONE',  ( 22.86252235622482587, -0.9498377794471745128, -13.29674124224850118 ) ) ;
#14565=CARTESIAN_POINT ( 'NONE',  ( 17.25718654270123409, 10.07213275844434364, -20.48022200034118612 ) ) ;
#14567=CARTESIAN_POINT ( 'NONE',  ( 32.58918748260075660, -11.04229556371213583, -18.21152344180378080 ) ) ;
#14569=CARTESIAN_POINT ( 'NONE',  ( 24.07691212630517796, -1.086650970500502300, -17.53382830850624785 ) ) ;
#14570=CARTESIAN_POINT ( 'NONE',  ( 18.48843674521961589, -1.244547778534776938, -16.48413177534300900 ) ) ;
#14572=CARTESIAN_POINT ( 'NONE',  ( 25.85465836959373220, -10.01954208144345770, -18.53069695322523103 ) ) ;
#14583=CARTESIAN_POINT ( 'NONE',  ( 34.28781561389841670, -12.04879923890588422, -19.89451123369701691 ) ) ;
#14585=CARTESIAN_POINT ( 'NONE',  ( 12.76278909782508997, 7.628803627606831839, -14.92072746316176790 ) ) ;
#14589=CARTESIAN_POINT ( 'NONE',  ( 13.05603179413191839, 8.545058472539723837, -15.96546128479914373 ) ) ;
#14598=CARTESIAN_POINT ( 'NONE',  ( 11.22518019566232716, 9.085373951847735441, -17.24107067304604257 ) ) ;
#14599=CARTESIAN_POINT ( 'NONE',  ( 25.27232213581778808, -7.536446408081735271, -18.87890555733638465 ) ) ;
#14600=CARTESIAN_POINT ( 'NONE',  ( 23.43951749033787735, -6.062008688038916127, -19.28752554440484701 ) ) ;
#14608=EDGE_CURVE ( 'NONE', #3493, #8851, #6655, .T. ) ;
#14618=CARTESIAN_POINT ( 'NONE',  ( 12.02817646543008934, 9.315460371489308500, -16.69127922251917795 ) ) ;
#14623=CARTESIAN_POINT ( 'NONE',  ( 13.38776246403941350, 7.629555522264023892, -15.70137656829213491 ) ) ;
#14625=CARTESIAN_POINT ( 'NONE',  ( 24.81358459371387326, -5.676498915796258871, -18.90393244824272756 ) ) ;
#14626=CARTESIAN_POINT ( 'NONE',  ( 12.81602886594196988, 9.615025227323064527, -16.14774825664093783 ) ) ;
#14631=CARTESIAN_POINT ( 'NONE',  ( 11.47327446659168615, 9.267463859335506982, -15.86074700677745852 ) ) ;
#14633=CARTESIAN_POINT ( 'NONE',  ( 9.907423389235603395, 16.44864837861227969, -16.50891839478055090 ) ) ;
#14638=CARTESIAN_POINT ( 'NONE',  ( 12.02799090998256304, 9.316311091778235465, -16.69135597610317134 ) ) ;
#14640=CARTESIAN_POINT ( 'NONE',  ( 36.54276536429808431, -23.15833126744076509, -18.75760452913613463 ) ) ;
#14641=CARTESIAN_POINT ( 'NONE',  ( 26.38113052396219516, -11.59678093645141672, -17.84452879788985769 ) ) ;
#14642=CARTESIAN_POINT ( 'NONE',  ( 17.06037746458228810, 10.50611453990982191, -19.02300506704843741 ) ) ;
#14647=CARTESIAN_POINT ( 'NONE',  ( 17.84334503882807255, 1.539790780908459000, -16.51430848555953190 ) ) ;
#14649=CARTESIAN_POINT ( 'NONE',  ( 16.06572049258021195, 3.735912457719189117, -15.00855390560170477 ) ) ;
#14660=CARTESIAN_POINT ( 'NONE',  ( 12.27187887740847039, 9.517710768097034091, -15.31277030567625452 ) ) ;
#14666=CARTESIAN_POINT ( 'NONE',  ( 11.92109019680886206, 8.606374460406147620, -15.56934379943068336 ) ) ;
#14668=CARTESIAN_POINT ( 'NONE',  ( 20.65939765650831461, 5.541921473274042498, -17.57530766875797568 ) ) ;
#14674=CARTESIAN_POINT ( 'NONE',  ( 12.83224840168406544, 9.540640483216481726, -16.14104089933701758 ) ) ;
#14677=CARTESIAN_POINT ( 'NONE',  ( 35.52138705868412671, -21.06228986472472897, -18.81697501280657647 ) ) ;
#14678=CARTESIAN_POINT ( 'NONE',  ( 20.52488529563827058, 3.974637744936419637, -19.97762432673833288 ) ) ;
#14682=CARTESIAN_POINT ( 'NONE',  ( 13.93491968177131923, 5.624373287173536795, -18.66784319378200863 ) ) ;
#14686=CARTESIAN_POINT ( 'NONE',  ( 24.47846259200217034, 0.2319951948203725633, -15.89054235832688278 ) ) ;
#14687=CARTESIAN_POINT ( 'NONE',  ( 18.77375537285786322, 7.252522315878067616, -16.50763127152984566 ) ) ;
#14698=CARTESIAN_POINT ( 'NONE',  ( 9.997747326010761881, 16.03441129093729245, -16.47093000352221637 ) ) ;
#14699=CARTESIAN_POINT ( 'NONE',  ( 28.63860307613198941, -6.423989724335291918, -15.76775560094196749 ) ) ;
#14700=CARTESIAN_POINT ( 'NONE',  ( 28.67999647541807207, -5.919990246138143952, -18.25217309140403188 ) ) ;
#14701=CARTESIAN_POINT ( 'NONE',  ( 33.35202879388211983, -12.33251541790028760, -19.68467382345759376 ) ) ;
#14710=CARTESIAN_POINT ( 'NONE',  ( 16.94076125623460527, 0.4124075662712927692, -16.40086227390004936 ) ) ;
#14712=CARTESIAN_POINT ( 'NONE',  ( 12.26747700539757346, 9.511763647452495363, -15.31658389161178668 ) ) ;
#14716=CARTESIAN_POINT ( 'NONE',  ( 17.33713706444265412, 0.9871066061555996418, -18.79342181739402307 ) ) ;
#14717=CARTESIAN_POINT ( 'NONE',  ( 12.84881458348222516, 5.748695638350556969, -17.40385974964576477 ) ) ;
#14719=CARTESIAN_POINT ( 'NONE',  ( 35.54859390953724585, -22.18451583373416014, -18.19919658220850778 ) ) ;
#14720=CARTESIAN_POINT ( 'NONE',  ( 22.14981412484149104, -6.473446789742020258, -15.39974742277494713 ) ) ;
#14722=CARTESIAN_POINT ( 'NONE',  ( 18.58892183794801056, 4.077935791202882854, -15.09018232067737841 ) ) ;
#14731=CARTESIAN_POINT ( 'NONE',  ( 36.54859390953724585, -22.18451583373416014, -17.78191007148576475 ) ) ;
#14732=CARTESIAN_POINT ( 'NONE',  ( 9.917205744531459644, 16.40378525026516243, -16.50423678068149869 ) ) ;
#14736=CARTESIAN_POINT ( 'NONE',  ( 12.11773132146483789, 9.045882004348337446, -16.64348121447567053 ) ) ;
#14752=CARTESIAN_POINT ( 'NONE',  ( 11.20778676255656059, 9.165115204199564047, -17.24826554773256149 ) ) ;
#14753=CARTESIAN_POINT ( 'NONE',  ( 25.32913879335529472, -12.33208189297920221, -17.76794973357399243 ) ) ;
#14754=CARTESIAN_POINT ( 'NONE',  ( 22.16683763302808430, -0.5050174593055701822, -13.96310542101677044 ) ) ;
#14764=CARTESIAN_POINT ( 'NONE',  ( 10.48212431696843439, 16.40585233633115436, -17.33062619162406293 ) ) ;
#14765=CARTESIAN_POINT ( 'NONE',  ( 35.54859215833182873, -22.18450796649496226, -18.40462262104107083 ) ) ;
#14767=CARTESIAN_POINT ( 'NONE',  ( 8.944584683310379702, 16.95159276115599667, -17.91664992932185996 ) ) ;
#14768=CARTESIAN_POINT ( 'NONE',  ( 26.80628776457338347, -3.176708023846821494, -16.02594779711905559 ) ) ;
#14769=CARTESIAN_POINT ( 'NONE',  ( 12.18385343395297049, 12.51426234204957844, -16.40917503585457737 ) ) ;
#14774=CARTESIAN_POINT ( 'NONE',  ( 11.47464782381437587, 9.261287281732329291, -15.86016978468419936 ) ) ;
#14777=ADVANCED_FACE ( 'NONE', ( #1460 ), #18876, .F. ) ;
#14778=CARTESIAN_POINT ( 'NONE',  ( 11.47327446659168615, 9.267463859335506982, -15.86074700677745852 ) ) ;
#14784=CARTESIAN_POINT ( 'NONE',  ( 11.76876341733043141, 10.50516141373230106, -16.79855566342228101 ) ) ;
#14786=CARTESIAN_POINT ( 'NONE',  ( 35.26378566547066384, -17.41255297500571331, -21.24391863398521352 ) ) ;
#14787=CARTESIAN_POINT ( 'NONE',  ( 29.72799312938100513, -7.689056491358781997, -15.42978383025728384 ) ) ;
#14788=CARTESIAN_POINT ( 'NONE',  ( 14.47211339546095488, 7.927559549074161716, -19.99378091926031686 ) ) ;
#14795=CARTESIAN_POINT ( 'NONE',  ( 18.10666546173949953, 1.615696121519054618, -15.79491705146812563 ) ) ;
#14796=CARTESIAN_POINT ( 'NONE',  ( 14.17177033308128031, 6.273687421093853800, -17.36430109743762173 ) ) ;
#14805=CARTESIAN_POINT ( 'NONE',  ( 12.27693567009463393, 9.494519571701449223, -15.31067915168583582 ) ) ;
#14809=CARTESIAN_POINT ( 'NONE',  ( 11.51951884677450266, 9.108496074915260365, -15.83757232928968683 ) ) ;
#14812=CARTESIAN_POINT ( 'NONE',  ( 16.84217415841480303, 1.412180072802544872, -16.35713574856416841 ) ) ;
#14824=CARTESIAN_POINT ( 'NONE',  ( 12.83280428553913666, 9.538383548424125280, -16.14078871935966220 ) ) ;
#14825=CARTESIAN_POINT ( 'NONE',  ( 34.85979932414094407, -13.59765634092047470, -19.03716015824713281 ) ) ;
#14826=CARTESIAN_POINT ( 'NONE',  ( 15.46244301724551740, 3.702889819443702990, -17.82701508041758842 ) ) ;
#14829=CARTESIAN_POINT ( 'NONE',  ( 17.78134717446047119, 9.288666448780150020, -20.14505390916605521 ) ) ;
#14832=CARTESIAN_POINT ( 'NONE',  ( 26.68716238812262631, -2.792712658874448639, -18.04699283665395981 ) ) ;
#14833=CARTESIAN_POINT ( 'NONE',  ( 20.19814137509539975, 5.716210941879356078, -15.87681946797394517 ) ) ;
#14838=CARTESIAN_POINT ( 'NONE',  ( 10.00000000000007816, 17.32050807568872486, -23.00000000000000711 ) ) ;
#14843=CARTESIAN_POINT ( 'NONE',  ( 11.69419402147360110, 8.800013620902292999, -15.72776802682527730 ) ) ;
#14844=CARTESIAN_POINT ( 'NONE',  ( 28.03106068525412908, -6.431813172927290267, -14.41205174211060402 ) ) ;
#14845=CARTESIAN_POINT ( 'NONE',  ( 27.71186802668094273, -7.007055141436442369, -19.33373627201896383 ) ) ;
#14846=CARTESIAN_POINT ( 'NONE',  ( 35.41344336761681433, -22.57735604011907071, -20.16400759377322061 ) ) ;
#14856=CARTESIAN_POINT ( 'NONE',  ( 22.29983652437130814, 0.6627547066652448304, -20.09853802436992964 ) ) ;
#14860=CARTESIAN_POINT ( 'NONE',  ( 12.27491818236995691, 9.503772128122387031, -15.31151344616081822 ) ) ;
#14862=CARTESIAN_POINT ( 'NONE',  ( 32.54305136433941215, -11.03529315477374517, -18.08112484791816499 ) ) ;
#14864=CARTESIAN_POINT ( 'NONE',  ( 25.55230692589818631, -0.5649882819070038975, -17.32853901032857280 ) ) ;
#14865=CARTESIAN_POINT ( 'NONE',  ( 19.50094987086785636, 1.087406662839465632, -19.92270839898774781 ) ) ;
#14867=CARTESIAN_POINT ( 'NONE',  ( 35.09336438560361415, -20.13941072448723801, -20.22035334018532637 ) ) ;
#14869=CARTESIAN_POINT ( 'NONE',  ( 23.53678897557974281, -9.624609092408482169, -17.82855203159936863 ) ) ;
#14870=CARTESIAN_POINT ( 'NONE',  ( 20.29686952095399377, -4.285349973794369660, -18.75376381207850329 ) ) ;
#14871=CARTESIAN_POINT ( 'NONE',  ( 24.36497833745277930, -6.082191617938494055, -18.74521747929614435 ) ) ;
#14878=CARTESIAN_POINT ( 'NONE',  ( 16.96387855261641775, 8.441957738943033362, -20.67322241009641814 ) ) ;
#14880=CARTESIAN_POINT ( 'NONE',  ( 35.91774987194125401, -19.35046774019819438, -20.39927477693754554 ) ) ;
#14881=CARTESIAN_POINT ( 'NONE',  ( 9.826288910175632552, 16.82074144182198694, -16.60662094963572244 ) ) ;
#14884=CARTESIAN_POINT ( 'NONE',  ( 12.02835731808789355, 9.314632867394664117, -16.69120428796748357 ) ) ;
#14897=CARTESIAN_POINT ( 'NONE',  ( 11.60705119439842292, 8.210639978236427439, -17.01629833992986462 ) ) ;
#14899=CARTESIAN_POINT ( 'NONE',  ( 32.75486304968715245, -9.956179044816899193, -14.71053347703266212 ) ) ;
#14900=CARTESIAN_POINT ( 'NONE',  ( 19.87821071931953298, -1.530402839103173651, -15.12151443550766494 ) ) ;
#14908=CARTESIAN_POINT ( 'NONE',  ( 32.20428705557502269, -10.20872362009771095, -14.89176492545819919 ) ) ;
#14910=DIRECTION ( 'NONE',  ( 0.3331260486002958765, -0.05059491534325381845, -0.9415238660200613285 ) ) ;
#14916=CARTESIAN_POINT ( 'NONE',  ( 12.03206445085756116, 9.298183410334813104, -16.68962916345529024 ) ) ;
#14917=CARTESIAN_POINT ( 'NONE',  ( 35.22227017426903473, -20.71851614966110233, -20.19360243392694088 ) ) ;
#14919=CARTESIAN_POINT ( 'NONE',  ( 8.944716491630211763, 16.95098827139963049, -17.88239910762268181 ) ) ;
#14921=CARTESIAN_POINT ( 'NONE',  ( 26.58455406938135468, -5.910422570377376950, -13.89432871846328688 ) ) ;
#14922=CARTESIAN_POINT ( 'NONE',  ( 12.83280428553913666, 9.538383548424125280, -16.14078871935966220 ) ) ;
#14931=CARTESIAN_POINT ( 'NONE',  ( 12.07641845611955489, 8.540206757827041528, -15.45582622123028216 ) ) ;
#14936=CARTESIAN_POINT ( 'NONE',  ( 12.02558468657594659, 9.327346335875439820, -16.69235103436730938 ) ) ;
#14939=CARTESIAN_POINT ( 'NONE',  ( 16.89391627328321732, 8.154734282165337689, -13.86877251323280014 ) ) ;
#14940=CARTESIAN_POINT ( 'NONE',  ( 27.26129135193747999, -10.77754955263135095, -18.64424489656416739 ) ) ;
#14945=CARTESIAN_POINT ( 'NONE',  ( 18.96452888794134495, 2.710274068595869057, -18.82741851907772457 ) ) ;
#14946=CARTESIAN_POINT ( 'NONE',  ( 17.63704213852533442, 9.806822523219006271, -18.50018230520716145 ) ) ;
#14959=CARTESIAN_POINT ( 'NONE',  ( 12.27289197906229745, 9.513064554772155290, -15.31235135250446078 ) ) ;
#14962=VERTEX_POINT ( 'NONE', #15776 ) ;
#14963=CARTESIAN_POINT ( 'NONE',  ( 12.37169234869624646, 8.529253869913038244, -15.23127513898213081 ) ) ;
#14965=CARTESIAN_POINT ( 'NONE',  ( 10.66844579733420062, 9.045745945026473223, -16.41129889692150812 ) ) ;
#14971=CARTESIAN_POINT ( 'NONE',  ( 12.31353044564305499, 11.91954703646417713, -16.35554902986205761 ) ) ;
#14972=CARTESIAN_POINT ( 'NONE',  ( 34.00275312277798889, -11.14511497259480244, -17.96532559481354596 ) ) ;
#14973=CARTESIAN_POINT ( 'NONE',  ( 19.20291185354690811, 8.143073066566493878, -16.32372945079811188 ) ) ;
#14978=CARTESIAN_POINT ( 'NONE',  ( 32.82164812444874968, -10.95096414870911161, -14.63344683186480211 ) ) ;
#14982=CARTESIAN_POINT ( 'NONE',  ( 24.30592326428028827, -5.273034306582022879, -19.67074064463221106 ) ) ;
#14984=CARTESIAN_POINT ( 'NONE',  ( 20.09928279393940898, 2.810699353624661168, -13.58730878818371401 ) ) ;
#14998=CARTESIAN_POINT ( 'NONE',  ( 11.47155695691762212, 9.275332456566969697, -15.86145787682774078 ) ) ;
#14999=CARTESIAN_POINT ( 'NONE',  ( 29.00298259868716499, -8.617193473538632631, -14.90553363820342092 ) ) ;
#15000=CARTESIAN_POINT ( 'NONE',  ( 27.85014272824177795, -5.137623357037004013, -13.74226875356335320 ) ) ;
#15009=CARTESIAN_POINT ( 'NONE',  ( 18.97268594440662426, -2.511067197207834667, -17.06021009607598415 ) ) ;
#15013=CARTESIAN_POINT ( 'NONE',  ( 12.27693567009463393, 9.494519571701449223, -15.31067915168583582 ) ) ;
#15014=AXIS2_PLACEMENT_3D ( 'NONE', #12076, #12369, #28915 ) ;
#15017=CARTESIAN_POINT ( 'NONE',  ( 20.50636976340433293, -0.9757509181830721356, -19.91080244439677571 ) ) ;
#15019=CARTESIAN_POINT ( 'NONE',  ( 19.21851095677833499, -0.002285697959038230937, -14.55609667925758544 ) ) ;
#15022=CARTESIAN_POINT ( 'NONE',  ( 28.04121823296437199, -4.154284946049297211, -14.96295611916008994 ) ) ;
#15023=CARTESIAN_POINT ( 'NONE',  ( 19.06759106800826586, -1.100202736525451641, -14.71838255749352165 ) ) ;
#15025=CARTESIAN_POINT ( 'NONE',  ( 31.59793210864275537, -10.01186915388335485, -14.42687813506083039 ) ) ;
#15036=CARTESIAN_POINT ( 'NONE',  ( 14.06424326207706699, 5.752694757912038881, -19.02294901845717945 ) ) ;
#15037=CARTESIAN_POINT ( 'NONE',  ( 36.07559364978101968, -20.05957622185551870, -20.44697815928661200 ) ) ;
#15038=CARTESIAN_POINT ( 'NONE',  ( 11.45256130090833935, 9.362448956408465861, -15.86931324879919991 ) ) ;
#15041=CARTESIAN_POINT ( 'NONE',  ( 13.15785925275590529, 8.585986940276173485, -15.88461348575242305 ) ) ;
#15052=CARTESIAN_POINT ( 'NONE',  ( 11.21589157578718421, 9.127945497600544300, -17.24491392235805876 ) ) ;
#15053=CARTESIAN_POINT ( 'NONE',  ( 28.86700826148938859, -9.048814421258168039, -19.66053155205330683 ) ) ;
#15054=CARTESIAN_POINT ( 'NONE',  ( 29.00434111665888182, -5.389956126880047549, -17.18324766788818181 ) ) ;
#15068=CARTESIAN_POINT ( 'NONE',  ( 12.07790154976966868, 9.144051220271959934, -16.66639656463015839 ) ) ;
#15069=CARTESIAN_POINT ( 'NONE',  ( 35.54859390953724585, -22.18451583373416014, -16.11276402859391865 ) ) ;
#15071=CARTESIAN_POINT ( 'NONE',  ( 9.122709158550120989, 16.13469121211704049, -17.05051537109504523 ) ) ;
#15072=CARTESIAN_POINT ( 'NONE',  ( 22.97938783112199701, -3.359759438970757017, -19.62490732200095067 ) ) ;
#15073=CARTESIAN_POINT ( 'NONE',  ( 10.35864918915110877, 16.97212501191939538, -21.33333333332589277 ) ) ;
#15078=CARTESIAN_POINT ( 'NONE',  ( 12.49899259368311988, 8.570259324921714494, -15.13097775544467005 ) ) ;
#15084=CARTESIAN_POINT ( 'NONE',  ( 12.98644063677341798, 8.526496012441747041, -16.01999686492960961 ) ) ;
#15089=CARTESIAN_POINT ( 'NONE',  ( 20.44279466453895822, 5.363259340322034774, -13.44374883282906552 ) ) ;
#15090=CARTESIAN_POINT ( 'NONE',  ( 22.66942224714451370, 5.529188492372526298, -17.57712505567429773 ) ) ;
#15096=CARTESIAN_POINT ( 'NONE',  ( 36.48591233058812833, -21.90292070287360460, -19.44112467175505898 ) ) ;
#15099=CARTESIAN_POINT ( 'NONE',  ( 18.47369133221681281, 7.987600538477567014, -15.27093437040897861 ) ) ;
#15106=CARTESIAN_POINT ( 'NONE',  ( 33.68411698100747032, -13.80840863474736935, -19.79436191385186916 ) ) ;
#15111=CARTESIAN_POINT ( 'NONE',  ( 11.04501277462238029, 15.14427510452705583, -15.82012259674246657 ) ) ;
#15116=CARTESIAN_POINT ( 'NONE',  ( 11.47748818427356987, 9.248962635895034978, -15.85894168489154765 ) ) ;
#15117=CARTESIAN_POINT ( 'NONE',  ( 12.69188586677704400, 7.599409645471840058, -14.97709067247704340 ) ) ;
#15123=CARTESIAN_POINT ( 'NONE',  ( 12.50804596317817463, 11.02747407808666580, -16.27511002087113567 ) ) ;
#15127=CARTESIAN_POINT ( 'NONE',  ( 35.54859390953723164, -21.18451583373416014, -14.99999999999999822 ) ) ;
#15129=CARTESIAN_POINT ( 'NONE',  ( 18.50902107916489570, 2.085137940960992697, -20.06823964296112450 ) ) ;
#15133=CARTESIAN_POINT ( 'NONE',  ( 18.04976943019953239, 10.79320383120880145, -15.74583687248850161 ) ) ;
#15137=CARTESIAN_POINT ( 'NONE',  ( 22.45293885382703536, -0.3771200753331621081, -14.01028023225368635 ) ) ;
#15138=CARTESIAN_POINT ( 'NONE',  ( 23.64629180402988951, 0.1506760071912668364, -12.95843554106259710 ) ) ;
#15148=CARTESIAN_POINT ( 'NONE',  ( 11.14863080475985591, 10.75631295387255548, -15.99499920034263489 ) ) ;
#15149=CARTESIAN_POINT ( 'NONE',  ( 16.06572049258021195, 3.735912457719189117, -15.00855390560170477 ) ) ;
#15150=CARTESIAN_POINT ( 'NONE',  ( 26.78588127033857091, -2.187643107580064861, -16.18476928258297676 ) ) ;
#15158=CARTESIAN_POINT ( 'NONE',  ( 20.14386580841007657, 1.771853782379294140, -13.30505882909219295 ) ) ;
#15162=CARTESIAN_POINT ( 'NONE',  ( 10.88291651000981730, 15.88766923650820928, -15.88715510423204513 ) ) ;
#15167=CARTESIAN_POINT ( 'NONE',  ( 20.99533150354982070, 4.487273811465053441, -19.54336078777620500 ) ) ;
#15170=CARTESIAN_POINT ( 'NONE',  ( 19.77504133826384347, 1.335633644655777053, -20.04176789066487530 ) ) ;
#15173=CARTESIAN_POINT ( 'NONE',  ( 26.42637521690935998, -6.951663299830703302, -19.91275981816901464 ) ) ;
#15175=CARTESIAN_POINT ( 'NONE',  ( 27.77130384954419995, -2.130748013457071099, -15.99611347415175366 ) ) ;
#15185=AXIS2_PLACEMENT_3D ( 'NONE', #18604, #14002, #447 ) ;
#15187=CARTESIAN_POINT ( 'NONE',  ( 26.57181397551241275, -7.970695015363167713, -12.68872038106934852 ) ) ;
#15189=CARTESIAN_POINT ( 'NONE',  ( 34.27125395597954594, -11.98684039141630819, -19.88226891060491752 ) ) ;
#15191=CARTESIAN_POINT ( 'NONE',  ( 10.24089172292967298, 14.91932009296530559, -16.37038124228770997 ) ) ;
#15194=CARTESIAN_POINT ( 'NONE',  ( 13.13233772467555660, 8.574708520419219937, -15.90495459411799395 ) ) ;
#15209=CARTESIAN_POINT ( 'NONE',  ( 8.944584683310379702, 16.95159276115599667, -17.94384837343789130 ) ) ;
#15210=CARTESIAN_POINT ( 'NONE',  ( 26.36605488913174611, -12.34709378291890758, -12.75955235896099005 ) ) ;
#15211=CARTESIAN_POINT ( 'NONE',  ( 26.42570577731286718, -9.588051360687080305, -12.79080846482418643 ) ) ;
#15222=CARTESIAN_POINT ( 'NONE',  ( 13.12723341905928898, 8.572452836447732594, -15.90902281579132449 ) ) ;
#15223=CARTESIAN_POINT ( 'NONE',  ( 33.14486676600987636, -11.77651092997264293, -17.78036478212233717 ) ) ;
#15225=CARTESIAN_POINT ( 'NONE',  ( 10.53902527060216343, 9.639284983934057749, -16.46481883690060144 ) ) ;
#15228=CARTESIAN_POINT ( 'NONE',  ( 25.04992766293576878, -3.547109489677171101, -13.67097983722207033 ) ) ;
#15229=CARTESIAN_POINT ( 'NONE',  ( 12.86851577213266928, 9.516150637207879015, -16.11522534726903899 ) ) ;
#15236=CARTESIAN_POINT ( 'NONE',  ( 11.47372892693763902, 9.265404009280679531, -15.86055721330185619 ) ) ;
#15244=CARTESIAN_POINT ( 'NONE',  ( 9.661883060892410668, 16.25482663691947849, -17.91599866193395485 ) ) ;
#15246=CARTESIAN_POINT ( 'NONE',  ( 15.30633068984937317, 3.801504677414661693, -19.72534293519717608 ) ) ;
#15247=CARTESIAN_POINT ( 'NONE',  ( 14.66608887309643272, 3.149405488550426568, -18.09902814372540192 ) ) ;
#15252=CARTESIAN_POINT ( 'NONE',  ( 18.69974902744413470, 8.051839821468062652, -15.50866580261103955 ) ) ;
#15259=CARTESIAN_POINT ( 'NONE',  ( 33.27037009343090546, -12.05169513820189309, -19.60996450177851713 ) ) ;
#15262=CARTESIAN_POINT ( 'NONE',  ( 11.05541573950045375, 17.68942145115775944, -17.91357985325011626 ) ) ;
#15269=CARTESIAN_POINT ( 'NONE',  ( 12.74324588813389170, 7.620242904383297322, -14.93629796730785486 ) ) ;
#15274=CARTESIAN_POINT ( 'NONE',  ( 11.43821061673542872, 15.93387534916056758, -16.71752457030684980 ) ) ;
#15275=CARTESIAN_POINT ( 'NONE',  ( 35.92974604556026463, -18.40436019371391652, -19.36057938427370217 ) ) ;
#15276=CARTESIAN_POINT ( 'NONE',  ( 19.50856600871340873, -1.908691058934758100, -18.90332006808282728 ) ) ;
#15280=CARTESIAN_POINT ( 'NONE',  ( 28.15263004948277725, -12.62334012340276779, -12.05588540746726345 ) ) ;
#15284=CARTESIAN_POINT ( 'NONE',  ( 26.42570577731286718, -9.588051360687080305, -12.79080846482418643 ) ) ;
#15285=CARTESIAN_POINT ( 'NONE',  ( 17.37750100583229340, 1.587821987789380440, -15.03969266580305764 ) ) ;
#15296=CARTESIAN_POINT ( 'NONE',  ( 10.70528834225764392, 11.46963701334067842, -17.45606632095149280 ) ) ;
#15297=CARTESIAN_POINT ( 'NONE',  ( 10.33811693838771717, 18.38618951776012267, -19.66666666666843000 ) ) ;
#15298=CARTESIAN_POINT ( 'NONE',  ( 28.12627659338356878, -5.062120396530918498, -14.05642262879015369 ) ) ;
#15306=CARTESIAN_POINT ( 'NONE',  ( 26.61709978538234012, -3.831456866606135492, -17.85214630790261836 ) ) ;
#15309=CARTESIAN_POINT ( 'NONE',  ( 31.49119590023542870, -10.87553819600004701, -15.10823507476435523 ) ) ;
#15310=CARTESIAN_POINT ( 'NONE',  ( 10.76134431155039373, 16.44521483549405971, -15.93742948484896615 ) ) ;
#15314=CARTESIAN_POINT ( 'NONE',  ( 28.16462234717350199, -5.661059359726887230, -16.30864077692347536 ) ) ;
#15317=CARTESIAN_POINT ( 'NONE',  ( 15.25645860304719292, 2.347722246533389789, -18.19294613283020112 ) ) ;
#15322=CARTESIAN_POINT ( 'NONE',  ( 25.80045869113294543, -2.244538201703065283, -16.37342509101419807 ) ) ;
#15323=CARTESIAN_POINT ( 'NONE',  ( 20.46682838619579670, -4.770343855991169058, -14.23415315410508342 ) ) ;
#15325=CARTESIAN_POINT ( 'NONE',  ( 28.06689949639850212, -8.111051215268487269, -13.49421662364394514 ) ) ;
#15336=CARTESIAN_POINT ( 'NONE',  ( 25.35799213500633442, -5.391047399292974163, -13.97031313328441726 ) ) ;
#15337=CARTESIAN_POINT ( 'NONE',  ( 17.25677449038176547, 8.733363079223632752, -20.54546673180767158 ) ) ;
#15338=CARTESIAN_POINT ( 'NONE',  ( 36.54859390953724585, -22.18451583373416014, -16.11276402859391865 ) ) ;
#15340=CARTESIAN_POINT ( 'NONE',  ( 9.907423389235603395, 16.44864837861227969, -16.50891839478055090 ) ) ;
#15343=CARTESIAN_POINT ( 'NONE',  ( 9.661883061612440926, 16.25482663361732705, -17.97192418671890835 ) ) ;
#15347=CARTESIAN_POINT ( 'NONE',  ( 11.46269231744662420, 9.315986823159681407, -15.86512371708112212 ) ) ;
#15354=CARTESIAN_POINT ( 'NONE',  ( 13.43370121458407418, 7.649856678006609734, -15.66476257323406784 ) ) ;
#15355=CARTESIAN_POINT ( 'NONE',  ( 34.30083361619418980, -13.08651950748960680, -20.95284133056243192 ) ) ;
#15356=CARTESIAN_POINT ( 'NONE',  ( 25.85217995398321378, -12.57279400931185620, -13.36530271656463320 ) ) ;
#15357=CARTESIAN_POINT ( 'NONE',  ( 29.30807694892355286, -8.357723062633453992, -13.20244061823602522 ) ) ;
#15378=CARTESIAN_POINT ( 'NONE',  ( 13.15785925275590529, 8.585986940276173485, -15.88461348575242305 ) ) ;
#15379=CARTESIAN_POINT ( 'NONE',  ( 33.61574637963836665, -12.50126044309498496, -18.73137083807847958 ) ) ;
#15382=CARTESIAN_POINT ( 'NONE',  ( 9.105507159292685060, 16.21358177345661389, -17.05825009255364932 ) ) ;
#15385=CARTESIAN_POINT ( 'NONE',  ( 26.48263329513011755, -12.06126822337667903, -13.95730679897583038 ) ) ;
#15386=CARTESIAN_POINT ( 'NONE',  ( 10.35864918915110877, 16.97212501191939538, -23.00000000000000711 ) ) ;
#15391=CARTESIAN_POINT ( 'NONE',  ( 11.47079713067724782, 9.278817116560638567, -15.86177209170659275 ) ) ;
#15395=CARTESIAN_POINT ( 'NONE',  ( 13.13063628947021755, 8.573956625762026107, -15.90631066800904669 ) ) ;
#15397=CARTESIAN_POINT ( 'NONE',  ( 13.40325769311605164, 6.909072298322937122, -18.40730773563142719 ) ) ;
#15398=CARTESIAN_POINT ( 'NONE',  ( 22.08592964957147586, 4.518037853963432049, -19.67680751601638889 ) ) ;
#15404=CARTESIAN_POINT ( 'NONE',  ( 25.21413058671614849, -1.115224416820481457, -18.44856734933592080 ) ) ;
#15413=CARTESIAN_POINT ( 'NONE',  ( 35.07504771885155037, -20.05712364337910714, -20.21480690768607857 ) ) ;
#15419=CARTESIAN_POINT ( 'NONE',  ( 15.36220012886423447, 10.89358938796158149, -12.84895098869522201 ) ) ;
#15420=CARTESIAN_POINT ( 'NONE',  ( 35.54859390953724585, -23.18451583373416014, -17.64281456791166391 ) ) ;
#15427=CARTESIAN_POINT ( 'NONE',  ( 10.71071464234916348, 8.878904022500222482, -16.39175934796422851 ) ) ;
#15433=CARTESIAN_POINT ( 'NONE',  ( 13.30397322184224329, 9.708587077508630259, -15.76815807330931030 ) ) ;
#15434=CARTESIAN_POINT ( 'NONE',  ( 36.32827445255054499, -20.19473721995742821, -19.46526261299151983 ) ) ;
#15435=CARTESIAN_POINT ( 'NONE',  ( 25.45462155318426767, -0.2439708902934435431, -15.99927030562601438 ) ) ;
#15443=CARTESIAN_POINT ( 'NONE',  ( 23.87675077653036126, -6.787291307973906562, -13.16608595595566733 ) ) ;
#15444=CARTESIAN_POINT ( 'NONE',  ( 19.75347561433959953, 2.650395817966514578, -13.58229691592852184 ) ) ;
#15456=CARTESIAN_POINT ( 'NONE',  ( 11.23377902493292879, 9.047655202846097922, -17.23738383348171865 ) ) ;
#15457=CARTESIAN_POINT ( 'NONE',  ( 12.49664108868010182, 8.569232744350554043, -15.13285098609708790 ) ) ;
#15465=CARTESIAN_POINT ( 'NONE',  ( 24.79644250101478065, -1.608028467720058918, -19.02763285027648976 ) ) ;
#15469=CARTESIAN_POINT ( 'NONE',  ( 11.05541531668977662, 17.68942339022145305, -17.95086732675816776 ) ) ;
#15474=CARTESIAN_POINT ( 'NONE',  ( 24.43075134246613800, -6.859861339260811874, -14.00379227226492951 ) ) ;
#15476=CARTESIAN_POINT ( 'NONE',  ( 21.70429774405079115, -3.429840324723197664, -17.59459576866303365 ) ) ;
#15478=CARTESIAN_POINT ( 'NONE',  ( 35.54859390953724585, -22.18451583373416014, -17.78191007148576475 ) ) ;
#15482=CARTESIAN_POINT ( 'NONE',  ( 27.18523481531828168, -13.05407500640787077, -12.66260957699712186 ) ) ;
#15483=CARTESIAN_POINT ( 'NONE',  ( 21.21264933382939333, -0.1440395243212932441, -13.28659446924270959 ) ) ;
#15485=CARTESIAN_POINT ( 'NONE',  ( 31.22280883588763700, -10.09333740185288875, -13.86128061636125786 ) ) ;
#15494=CARTESIAN_POINT ( 'NONE',  ( 27.00779440489029071, -4.779404007149373079, -14.88408750732950914 ) ) ;
#15495=CARTESIAN_POINT ( 'NONE',  ( 16.22940209442605308, 10.22534693890197133, -14.12725775589269084 ) ) ;
#15496=CARTESIAN_POINT ( 'NONE',  ( 35.76309413546784555, -19.65568143964299352, -21.39484760613106573 ) ) ;
#15498=CARTESIAN_POINT ( 'NONE',  ( 11.55687758731922798, 9.016417257711555777, -15.81607864292198329 ) ) ;
#15500=CARTESIAN_POINT ( 'NONE',  ( 13.15390973649967599, 8.859676595473322536, -14.60899741038990562 ) ) ;
#15501=CARTESIAN_POINT ( 'NONE',  ( 13.23272240178861381, 8.619070305187777947, -15.82494623455082916 ) ) ;
#15504=CARTESIAN_POINT ( 'NONE',  ( 11.47181023233108021, 9.274170903235749108, -15.86135313853478657 ) ) ;
#15510=CARTESIAN_POINT ( 'NONE',  ( 31.88113401528661939, -11.03952345999570994, -14.96145667752709763 ) ) ;
#15512=CARTESIAN_POINT ( 'NONE',  ( 8.944585970659694851, 16.95158685720792846, -17.91243444582771005 ) ) ;
#15513=CARTESIAN_POINT ( 'NONE',  ( 36.06101586692013683, -20.99408596552883566, -21.31372499146719690 ) ) ;
#15517=CARTESIAN_POINT ( 'NONE',  ( 21.96101381878726500, 3.467707295883769802, -19.37612211972275844 ) ) ;
#15519=CARTESIAN_POINT ( 'NONE',  ( 30.07542022419311678, -8.155067017681195907, -14.09159111155252120 ) ) ;
#15525=CARTESIAN_POINT ( 'NONE',  ( 22.41093758190154972, 3.143874582428516806, -16.84310506638757943 ) ) ;
#15533=CARTESIAN_POINT ( 'NONE',  ( 12.35422140817580683, 8.720385185214494683, -16.48779044034850116 ) ) ;
#15534=CARTESIAN_POINT ( 'NONE',  ( 35.52138705868412671, -21.06228986472472897, -18.81697501280657647 ) ) ;
#15537=CARTESIAN_POINT ( 'NONE',  ( 9.111161770198492604, 16.18764900704733378, -17.05531488649033633 ) ) ;
#15539=CARTESIAN_POINT ( 'NONE',  ( 24.62590367393082502, -9.567571807129121808, -15.85044010117769098 ) ) ;
#15540=CARTESIAN_POINT ( 'NONE',  ( 10.35864918915110877, 16.97212501191939538, -17.93331994345748370 ) ) ;
#15550=CARTESIAN_POINT ( 'NONE',  ( 9.661883061612440926, 16.25482663361732705, -17.92454625180715411 ) ) ;
#15551=CARTESIAN_POINT ( 'NONE',  ( 16.54285080251403173, 3.669380853427548939, -13.47387114519368012 ) ) ;
#15552=CARTESIAN_POINT ( 'NONE',  ( 18.76724195421386554, 7.045283186750163296, -20.62625128596355495 ) ) ;
#15558=CARTESIAN_POINT ( 'NONE',  ( 21.79935899731381710, -1.430375723040585356, -13.25318265510616733 ) ) ;
#15565=CARTESIAN_POINT ( 'NONE',  ( 33.40713826534622655, -12.56408340279653757, -19.71064172033093698 ) ) ;
#15570=CARTESIAN_POINT ( 'NONE',  ( 12.24552273913795730, 9.516269270964150095, -15.33299823368393078 ) ) ;
#15571=CARTESIAN_POINT ( 'NONE',  ( 33.29928106196997817, -12.14339677642331772, -19.64090527578606427 ) ) ;
#15573=( BOUNDED_SURFACE ( )  B_SPLINE_SURFACE ( 3, 3, ( 
 ( #1564, #29381, #20152, #20301, #29690, #4142, #4591, #5035, #18926, #6734, #14326, #2321, #25955, #20750, #9303, #7035, #18473, #14180, #321, #25804, #9449, #23356, #21207, #30139, #4444, #11890, #6893, #18773, #7185, #13739, #28280, #28126, #23066, #9145, #9607, #4885, #7337, #23507, #27827, #2617, #15, #16478, #16636, #23661, #16026, #2165, #18628, #16327, #16183, #27976, #2765, #12049, #29987, #25643, #8997, #18315, #11439, #25502, #13880, #169, #20904, #27673, #23203, #2472, #11591, #4735, #25351, #14028, #11746, #21064, #21656, #10785, #27150, #1340, #3774, #10629, #20093, #29470, #7776, #22391, #28572, #23820, #16931, #6213, #16783, #2917, #8488, #12199, #7625, #26262, #27000, #22229, #5344, #21514, #469, #9756, #19076, #6061, #17791, #15347, #19939, #28428, #17643, #620, #26412, #757, #15504, #12344, #9905, #21362, #24835, #19214, #29307, #5491, #10053, #8341, #17087, #14631, #3926, #24684, #7480, #14774, #13068, #23978, #3070, #19368, #28730, #24116, #1496, #26111, #3214, #12914, #5186, #14483, #13671, #11082, #11232, #22848, #27602, #18402, #6662, #2098, #15804, #4075, #8636, #17938, #1949, #25429, #30064, #9075, #27754, #6814, #27908, #24993, #22996, #22693, #29773, #8929, #15954, #16108, #13369, #20383, #11375, #8783, #1794, #22548, #1646, #10925, #4519, #20831, #13807, #20679, #20233, #23135, #18098, #18247, #20535, #18551, #4221, #27462, #13226, #30214, #6514, #2244, #25281, #13518 ),
 ( #4370, #11517, #25131, #29922, #9223, #15660, #6966, #16254, #25567, #29622, #27312, #6366, #23441, #5116, #2553, #2689, #14257, #19008, #9843, #28366, #23749, #7264, #25732, #95, #9380, #23589, #16863, #21447, #558, #19155, #28512, #19300, #16409, #14409, #14108, #21140, #399, #7421, #7561, #4814, #11824, #14561, #26195, #23909, #5274, #251, #3004, #4967, #12132, #12282, #21601, #20988, #28053, #11970, #21289, #9527, #9683, #698, #9985, #2846, #16721, #28659, #7712, #18706, #7107, #18850, #17021, #25889, #4660, #28211, #26041, #16566, #13955, #23287, #2398, #11672, #24200, #26651, #15310, #1459, #5881, #8303, #15162, #24643, #3738, #12732, #26966, #3302, #28821, #21897, #10749, #21746, #7859, #13036, #17168, #12577, #1011, #1303, #10290, #26497, #5578, #19903, #22353, #19598, #14860, #5426, #28967, #26809, #8003, #24343, #5730, #10435, #10593, #19744, #24498, #17311, #15013, #848, #10138, #3439, #17610, #12879, #22193, #29269, #6027, #20057, #22054, #3589, #1156, #29113, #8154, #17460, #29431, #8450, #26345, #14712, #24055, #3155, #12428, #19452, #20644, #18062, #25244, #9038, #16069, #3890, #10888, #27425, #25093, #6328, #15769, #11340, #30030, #27568, #4183, #13777, #20797, #22512, #20199, #1612, #18211, #8745, #18361, #15624, #11192, #29582, #8599, #30182, #13477, #25395, #24958, #6480, #6776, #23105, #6623, #27718, #15915, #4486, #2208, #22808, #11482, #4038, #17898, #13332, #17758, #13189 ),
 ( #4333, #22656, #27279, #27114, #6175, #15469, #22959, #24800, #2061, #13629, #1756, #11046, #20347, #1914, #20501, #29738, #29887, #8896, #9191, #16823, #61, #9651, #14223, #213, #18971, #25853, #4783, #23867, #7385, #2966, #23554, #23708, #9345, #14073, #2656, #18815, #14524, #9491, #18672, #18516, #26157, #28017, #28328, #11932, #28173, #16680, #4932, #23402, #12244, #26003, #21562, #21254, #2810, #7076, #2519, #11787, #11637, #20950, #12093, #5231, #21107, #16371, #27876, #25692, #5079, #7230, #16530, #365, #14370, #21410, #514, #9805, #19117, #28473, #4630, #13922, #7521, #6931, #16224, #25538, #23253, #2365, #15274, #12390, #1123, #10097, #17131, #26609, #14971, #15123, #807, #7823, #10552, #5839, #19862, #24456, #19411, #3551, #967, #8115, #22155, #29225, #16979, #24018, #10248, #7966, #28781, #28930, #12843, #1265, #10401, #17275, #26925, #3697, #5388, #3118, #14674, #19708, #21855, #8262, #26458, #24306, #21702, #5539, #12999, #5692, #17571, #14824, #19563, #5985, #24606, #29072, #661, #17420, #9946, #19259, #3401, #28615, #24159, #3263, #12538, #7672, #26305, #12694, #22015, #26768, #29542, #8560, #27536, #22773, #17862, #13149, #1419, #10709, #20018, #6590, #29999, #15879, #1879, #29388, #18178, #22473, #4301, #27078, #11308, #8412, #25210, #20611, #27681, #27391, #13600, #17719, #27237, #11159, #15734, #9003, #6135, #18323, #16033, #6287, #20465, #15433, #22928, #24763, #2028, #6741 ),
 ( #29697, #10850, #20308, #25359, #4452, #29854, #8710, #22311, #3851, #1571, #20159, #15584, #8860, #13299, #24918, #4000, #25061, #22618, #1717, #11003, #18026, #6445, #4148, #13442, #2773, #19083, #23515, #25962, #2625, #12056, #21369, #179, #14334, #20912, #16191, #9312, #28435, #9153, #25509, #476, #4599, #25, #18638, #18934, #14188, #27984, #13887, #23074, #2173, #11449, #28289, #9766, #7344, #11900, #20757, #9614, #23214, #18782, #23364, #7487, #4745, #2330, #13746, #16791, #11599, #21216, #28135, #14036, #330, #9458, #7044, #26118, #16643, #30146, #7193, #5042, #16335, #25652, #2481, #11754, #21072, #23669, #18480, #16488, #25812, #27837, #4894, #6900, #3082, #3221, #14784, #19527, #10366, #28898, #24272, #7784, #26270, #627, #23828, #14490, #19671, #12811, #29036, #14936, #2924, #1089, #5351, #10214, #24124, #10512, #26419, #14638, #5196, #22125, #23985, #5654, #7929, #5498, #3370, #21822, #765, #19825, #12657, #29189, #17240, #8075, #12351, #10061, #19375, #7633, #16940, #17384, #1228, #28739, #21664, #12206, #17094, #21976, #12499, #923, #26571, #26729, #5802, #15084, #24423, #3518, #8226, #9912, #19223, #17535, #21525, #28579, #22737, #13411, #1848, #11274, #8380, #27356, #6101, #13111, #22586, #10967, #11128, #27046, #3817, #6554, #20429, #15845, #29820, #15395, #8828, #27203, #4116, #18142, #25175, #12959, #19983, #6255, #3970, #24729, #24884, #27503, #4266, #6413, #13269, #22892 ),
 ( #13567, #22436, #20277, #1384, #10675, #8970, #1686, #1994, #1538, #15550, #20578, #29964, #15702, #26891, #25031, #5956, #15244, #29663, #24576, #10821, #29355, #20130, #3664, #22274, #17687, #29510, #8531, #17832, #8678, #17984, #18744, #25469, #9115, #27643, #18597, #25773, #9571, #16606, #4419, #11415, #27948, #25605, #6863, #16293, #11865, #21177, #28090, #4703, #14299, #21330, #23038, #20720, #2140, #7151, #9268, #289, #16151, #11714, #30107, #18447, #437, #13995, #25928, #4560, #7005, #7302, #23633, #16451, #18893, #4852, #5009, #2731, #23324, #28252, #13848, #27797, #23175, #12015, #13713, #2287, #18286, #11557, #20874, #30256, #23480, #14153, #2438, #21033, #6709, #15999, #25328, #2589, #139, #9419, #19493, #7456, #5617, #9878, #14752, #19338, #15052, #728, #19190, #9724, #17349, #593, #10181, #24090, #10024, #28863, #26387, #5314, #24385, #7899, #3484, #3190, #24239, #28545, #14598, #23950, #12169, #21488, #3339, #26695, #3043, #7597, #19047, #16903, #17208, #26233, #7750, #28702, #12467, #14897, #21789, #26537, #12315, #21631, #5162, #14452, #17059, #21939, #12620, #1052, #10330, #19637, #12775, #5464, #29003, #889, #8042, #5770, #22092, #28402, #16758, #26081, #23790, #2886, #20390, #15667, #19947, #4083, #13376, #10637, #6068, #22700, #1807, #11089, #10476, #29314, #29781, #25000, #8498, #13235, #8789, #15354, #6522, #18106, #8192, #15812, #3780, #27468, #22238, #10793, #17797, #8348 ),
 ( #1349, #5923, #25137, #17650, #10932, #8642, #15209, #4228, #20243, #24541, #27012, #24693, #13529, #3629, #6219, #12922, #1196, #13077, #19787, #17503, #29152, #26854, #22400, #15512, #6376, #1503, #20100, #29630, #24846, #29478, #27159, #3932, #22556, #1654, #17945, #27320, #2816, #8938, #12099, #14376, #23713, #2973, #21416, #28336, #18254, #19123, #27760, #13678, #6672, #14530, #2253, #20838, #23873, #22854, #26009, #522, #25436, #1956, #9810, #370, #9085, #15961, #30073, #11238, #18410, #4527, #7390, #6827, #23004, #9657, #16115, #28480, #5238, #20687, #13815, #7526, #11383, #18978, #25291, #20542, #23143, #29931, #11526, #16686, #27609, #4380, #5088, #16832, #26162, #2106, #12838, #3394, #21849, #959, #10241, #17714, #20154, #27072, #10395, #22150, #1565, #17858, #22305, #24759, #1411, #10845, #29536, #29218, #13138, #19703, #14965, #8106, #27231, #7959, #24299, #8554, #12687, #29067, #6281, #3691, #22467, #1258, #22009, #19556, #28924, #17268, #6130, #15577, #15427, #10704, #26598, #8407, #1116, #17565, #10545, #24909, #3544, #17414, #12531, #5685, #26761, #12993, #26918, #19853, #20013, #8255, #5831, #15117, #29383, #24450, #5980, #3845, #15269, #24600, #8854, #6437, #15728, #27829, #20906, #27530, #22767, #13293, #1874, #4445, #11154, #2021, #13595, #18317, #9146, #27675, #23068, #6584, #25057, #29691, #8704, #22921, #16184, #20752, #30140, #18474, #6894, #18630, #4143, #13740, #13437, #20457 ),
 ( #18169, #2167, #10996, #25503, #18018, #4593, #13881, #23206, #16329, #2323, #11441, #27384, #11593, #15873, #29848, #25204, #27978, #29990, #6735, #7038, #3994, #18, #9306, #4295, #22612, #1710, #8998, #11302, #20605, #16028, #20303, #25352, #28283, #7482, #7339, #16933, #3075, #23509, #25957, #622, #4888, #9759, #171, #759, #9609, #10056, #14182, #11893, #14633, #7778, #16638, #16786, #19078, #9452, #12346, #2475, #9907, #2619, #21209, #12051, #2919, #25646, #28574, #324, #18928, #26265, #5346, #23980, #4738, #5037, #21659, #19217, #2768, #26113, #7628, #14329, #19370, #28732, #11748, #14030, #23663, #23358, #16481, #21364, #471, #28430, #21066, #18775, #21518, #5189, #14485, #28129, #25806, #7187, #23822, #12201, #26886, #24571, #917, #6096, #5950, #21817, #17235, #24267, #15391, #19522, #22120, #28893, #29350, #10206, #24725, #3216, #1377, #3812, #22431, #1222, #22268, #14778, #3365, #15236, #10506, #13105, #7924, #1534, #10816, #21970, #3659, #24119, #10670, #26565, #19977, #12954, #8374, #29506, #17682, #17529, #5649, #20126, #29031, #14931, #12651, #17089, #12806, #19819, #26414, #5493, #27039, #12494, #17379, #1084, #10361, #29184, #19665, #8069, #26724, #5797, #15078, #24418, #8221, #3512, #10963, #22886, #1989, #13709, #11269, #27638, #11123, #29659, #3966, #13263, #18134, #20715, #25321, #4414, #23034, #2136, #23171, #20271, #8965, #17979, #25026, #4260, #20572, #11410, #8674, #15696 ) ),
 .UNSPECIFIED., .T., .F., .F. ) 
 B_SPLINE_SURFACE_WITH_KNOTS ( ( 4, 3, 4 ),
 ( 4, 2, 2, 2, 2, 2, 2, 2, 2, 2, 2, 2, 2, 2, 2, 2, 2, 2, 2, 2, 2, 2, 2, 2, 2, 2, 2, 2, 2, 2, 2, 2, 2, 2, 2, 2, 2, 2, 2, 2, 2, 2, 2, 2, 2, 2, 2, 2, 2, 2, 2, 2, 2, 2, 2, 2, 2, 2, 2, 2, 2, 2, 2, 2, 2, 2, 2, 2, 2, 2, 2, 2, 2, 2, 2, 2, 2, 2, 2, 2, 2, 2, 2, 2, 2, 2, 2, 2, 2, 2, 2, 2, 4 ),
 ( 0.000000000000000000, 0.5000000000000000000, 1.000000000000000000 ),
 ( 0.000000000000000000, 0.2329478137359916323, 0.2349098735327962983, 0.2358909034311986175, 0.2363814183803997770, 0.2366266758550003568, 0.2367493045923006467, 0.2368106189609507917, 0.2368719333296009644, 0.2369056680493116240, 0.2369394027690223115, 0.2370068722084436863, 0.2371418110872863805, 0.2374116888449718243, 0.2379514443603427121, 0.2390309553910844875, 0.2411899774525679829, 0.2455080215755349737, 0.2541441098214689553, 0.2714162863133369186, 0.2886884628052048818, 0.2973245510511388634, 0.3016425951741058542, 0.3038016172355893496, 0.3048811282663310696, 0.3054208837817019573, 0.3056907615393874011, 0.3058257004182300953, 0.3058931698576514702, 0.3059269045773621576, 0.3059606392970728450, 0.3060023410584322145, 0.3060440428197915841, 0.3061274463425103787, 0.3062942533879479123, 0.3066278674788229797, 0.3072950956605731143, 0.3086295520240733836, 0.3112984647510739222, 0.3166362902050750550, 0.3273119411130772649, 0.3486632429290816293, 0.3913658465610904136, 0.4767710538251080377, 0.5621762610891256617, 0.6048788647211345015, 0.6262301665371388104, 0.6369058174451409648, 0.6422436428991420421, 0.6449125556261425807, 0.6462470119896428500, 0.6469142401713929846, 0.6472478542622681630, 0.6474146613077056411, 0.6474980648304244912, 0.6475397665917839163, 0.6475814683531432303, 0.6476196945210073164, 0.6476579206888715134, 0.6477343730245996856, 0.6478872776960560298, 0.6481930870389687183, 0.6488047057247940952, 0.6500279430964450711, 0.6524744178397468009, 0.6573673673263502604, 0.6671532662995571794, 0.6769391652727642095, 0.6867250642459712395, 0.6965109632191782696, 0.7062968621923852997, 0.7160827611655922187, 0.7209757106521956782, 0.7234221853954974080, 0.7246454227671483839, 0.7252570414529737608, 0.7255628507958864493, 0.7257157554673427935, 0.7257922078030709656, 0.7258304339709351627, 0.7258686601387992487, 0.7259088784260310234, 0.7259490967132626871, 0.7260295332877260144, 0.7261904064366526690, 0.7265121527345062002, 0.7271556453302130407, 0.7284426305216267217, 0.7310166009044543056, 0.7361645416701092515, 0.7464604232014193652, 0.7670521862640395927, 1.000000000000000000 ),
 .UNSPECIFIED. ) 
 GEOMETRIC_REPRESENTATION_ITEM ( )  RATIONAL_B_SPLINE_SURFACE ( (
 ( 1.000000000000000000, 1.000000000000000000, 1.000000000000000000, 1.000000000000000000, 1.000000000000000000, 1.000000000000000000, 1.000000000000000000, 1.000000000000000000, 1.000000000000000000, 1.000000000000000000, 1.000000000000000000, 1.000000000000000000, 1.000000000000000000, 1.000000000000000000, 1.000000000000000000, 1.000000000000000000, 1.000000000000000000, 1.000000000000000000, 1.000000000000000000, 1.000000000000000000, 1.000000000000000000, 1.000000000000000000, 1.000000000000000000, 1.000000000000000000, 1.000000000000000000, 1.000000000000000000, 1.000000000000000000, 1.000000000000000000, 1.000000000000000000, 1.000000000000000000, 1.000000000000000000, 1.000000000000000000, 1.000000000000000000, 1.000000000000000000, 1.000000000000000000, 1.000000000000000000, 1.000000000000000000, 1.000000000000000000, 1.000000000000000000, 1.000000000000000000, 1.000000000000000000, 1.000000000000000000, 1.000000000000000000, 1.000000000000000000, 1.000000000000000000, 1.000000000000000000, 1.000000000000000000, 1.000000000000000000, 1.000000000000000000, 1.000000000000000000, 1.000000000000000000, 1.000000000000000000, 1.000000000000000000, 1.000000000000000000, 1.000000000000000000, 1.000000000000000000, 1.000000000000000000, 1.000000000000000000, 1.000000000000000000, 1.000000000000000000, 1.000000000000000000, 1.000000000000000000, 1.000000000000000000, 1.000000000000000000, 1.000000000000000000, 1.000000000000000000, 1.000000000000000000, 1.000000000000000000, 1.000000000000000000, 1.000000000000000000, 1.000000000000000000, 1.000000000000000000, 1.000000000000000000, 1.000000000000000000, 1.000000000000000000, 1.000000000000000000, 1.000000000000000000, 1.000000000000000000, 1.000000000000000000, 1.000000000000000000, 1.000000000000000000, 1.000000000000000000, 1.000000000000000000, 1.000000000000000000, 1.000000000000000000, 1.000000000000000000, 1.000000000000000000, 1.000000000000000000, 1.000000000000000000, 1.000000000000000000, 1.000000000000000000, 1.000000000000000000, 1.000000000000000000, 1.000000000000000000, 1.000000000000000000, 1.000000000000000000, 1.000000000000000000, 1.000000000000000000, 1.000000000000000000, 1.000000000000000000, 1.000000000000000000, 1.000000000000000000, 1.000000000000000000, 1.000000000000000000, 1.000000000000000000, 1.000000000000000000, 1.000000000000000000, 1.000000000000000000, 1.000000000000000000, 1.000000000000000000, 1.000000000000000000, 1.000000000000000000, 1.000000000000000000, 1.000000000000000000, 1.000000000000000000, 1.000000000000000000, 1.000000000000000000, 1.000000000000000000, 1.000000000000000000, 1.000000000000000000, 1.000000000000000000, 1.000000000000000000, 1.000000000000000000, 1.000000000000000000, 1.000000000000000000, 1.000000000000000000, 1.000000000000000000, 1.000000000000000000, 1.000000000000000000, 1.000000000000000000, 1.000000000000000000, 1.000000000000000000, 1.000000000000000000, 1.000000000000000000, 1.000000000000000000, 1.000000000000000000, 1.000000000000000000, 1.000000000000000000, 1.000000000000000000, 1.000000000000000000, 1.000000000000000000, 1.000000000000000000, 1.000000000000000000, 1.000000000000000000, 1.000000000000000000, 1.000000000000000000, 1.000000000000000000, 1.000000000000000000, 1.000000000000000000, 1.000000000000000000, 1.000000000000000000, 1.000000000000000000, 1.000000000000000000, 1.000000000000000000, 1.000000000000000000, 1.000000000000000000, 1.000000000000000000, 1.000000000000000000, 1.000000000000000000, 1.000000000000000000, 1.000000000000000000, 1.000000000000000000, 1.000000000000000000, 1.000000000000000000, 1.000000000000000000, 1.000000000000000000, 1.000000000000000000, 1.000000000000000000, 1.000000000000000000, 1.000000000000000000, 1.000000000000000000, 1.000000000000000000, 1.000000000000000000, 1.000000000000000000, 1.000000000000000000, 1.000000000000000000, 1.000000000000000000, 1.000000000000000000, 1.000000000000000000, 1.000000000000000000, 1.000000000000000000, 1.000000000000000000, 1.000000000000000000, 1.000000000000000000, 1.000000000000000000, 1.000000000000000000),
 ( 0.3333333333333333703, 0.3333333333333333703, 0.3333333333333333703, 0.3333333333333333703, 0.3333333333333333703, 0.3333333333333333703, 0.3333333333333333703, 0.3333333333333333703, 0.3333333333333333703, 0.3333333333333333703, 0.3333333333333333703, 0.3333333333333333703, 0.3333333333333333703, 0.3333333333333333703, 0.3333333333333333703, 0.3333333333333333703, 0.3333333333333333703, 0.3333333333333333703, 0.3333333333333333703, 0.3333333333333333703, 0.3333333333333333703, 0.3333333333333333703, 0.3333333333333333703, 0.3333333333333333703, 0.3333333333333333703, 0.3333333333333333703, 0.3333333333333333703, 0.3333333333333333703, 0.3333333333333333703, 0.3333333333333333703, 0.3333333333333333703, 0.3333333333333333703, 0.3333333333333333703, 0.3333333333333333703, 0.3333333333333333703, 0.3333333333333333703, 0.3333333333333333703, 0.3333333333333333703, 0.3333333333333333703, 0.3333333333333333703, 0.3333333333333333703, 0.3333333333333333703, 0.3333333333333333703, 0.3333333333333333703, 0.3333333333333333703, 0.3333333333333333703, 0.3333333333333333703, 0.3333333333333333703, 0.3333333333333333703, 0.3333333333333333703, 0.3333333333333333703, 0.3333333333333333703, 0.3333333333333333703, 0.3333333333333333703, 0.3333333333333333703, 0.3333333333333333703, 0.3333333333333333703, 0.3333333333333333703, 0.3333333333333333703, 0.3333333333333333703, 0.3333333333333333703, 0.3333333333333333703, 0.3333333333333333703, 0.3333333333333333703, 0.3333333333333333703, 0.3333333333333333703, 0.3333333333333333703, 0.3333333333333333703, 0.3333333333333333703, 0.3333333333333333703, 0.3333333333333333703, 0.3333333333333333703, 0.3333333333333333703, 0.3333333333333333703, 0.3333333333333333703, 0.3333333333333333703, 0.3333333333333333703, 0.3333333333333333703, 0.3333333333333333703, 0.3333333333333333703, 0.3333333333333333703, 0.3333333333333333703, 0.3333333333333333703, 0.3333333333333333703, 0.3333333333333333703, 0.3333333333333333703, 0.3333333333333333703, 0.3333333333333333703, 0.3333333333333333703, 0.3333333333333333703, 0.3333333333333333703, 0.3333333333333333703, 0.3333333333333333703, 0.3333333333333333703, 0.3333333333333333703, 0.3333333333333333703, 0.3333333333333333703, 0.3333333333333333703, 0.3333333333333333703, 0.3333333333333333703, 0.3333333333333333703, 0.3333333333333333703, 0.3333333333333333703, 0.3333333333333333703, 0.3333333333333333703, 0.3333333333333333703, 0.3333333333333333703, 0.3333333333333333703, 0.3333333333333333703, 0.3333333333333333703, 0.3333333333333333703, 0.3333333333333333703, 0.3333333333333333703, 0.3333333333333333703, 0.3333333333333333703, 0.3333333333333333703, 0.3333333333333333703, 0.3333333333333333703, 0.3333333333333333703, 0.3333333333333333703, 0.3333333333333333703, 0.3333333333333333703, 0.3333333333333333703, 0.3333333333333333703, 0.3333333333333333703, 0.3333333333333333703, 0.3333333333333333703, 0.3333333333333333703, 0.3333333333333333703, 0.3333333333333333703, 0.3333333333333333703, 0.3333333333333333703, 0.3333333333333333703, 0.3333333333333333703, 0.3333333333333333703, 0.3333333333333333703, 0.3333333333333333703, 0.3333333333333333703, 0.3333333333333333703, 0.3333333333333333703, 0.3333333333333333703, 0.3333333333333333703, 0.3333333333333333703, 0.3333333333333333703, 0.3333333333333333703, 0.3333333333333333703, 0.3333333333333333703, 0.3333333333333333703, 0.3333333333333333703, 0.3333333333333333703, 0.3333333333333333703, 0.3333333333333333703, 0.3333333333333333703, 0.3333333333333333703, 0.3333333333333333703, 0.3333333333333333703, 0.3333333333333333703, 0.3333333333333333703, 0.3333333333333333703, 0.3333333333333333703, 0.3333333333333333703, 0.3333333333333333703, 0.3333333333333333703, 0.3333333333333333703, 0.3333333333333333703, 0.3333333333333333703, 0.3333333333333333703, 0.3333333333333333703, 0.3333333333333333703, 0.3333333333333333703, 0.3333333333333333703, 0.3333333333333333703, 0.3333333333333333703, 0.3333333333333333703, 0.3333333333333333703, 0.3333333333333333703, 0.3333333333333333703, 0.3333333333333333703, 0.3333333333333333703, 0.3333333333333333703, 0.3333333333333333703, 0.3333333333333333703, 0.3333333333333333703, 0.3333333333333333703, 0.3333333333333333703, 0.3333333333333333703),
 ( 0.3333333333333333703, 0.3333333333333333703, 0.3333333333333333703, 0.3333333333333333703, 0.3333333333333333703, 0.3333333333333333703, 0.3333333333333333703, 0.3333333333333333703, 0.3333333333333333703, 0.3333333333333333703, 0.3333333333333333703, 0.3333333333333333703, 0.3333333333333333703, 0.3333333333333333703, 0.3333333333333333703, 0.3333333333333333703, 0.3333333333333333703, 0.3333333333333333703, 0.3333333333333333703, 0.3333333333333333703, 0.3333333333333333703, 0.3333333333333333703, 0.3333333333333333703, 0.3333333333333333703, 0.3333333333333333703, 0.3333333333333333703, 0.3333333333333333703, 0.3333333333333333703, 0.3333333333333333703, 0.3333333333333333703, 0.3333333333333333703, 0.3333333333333333703, 0.3333333333333333703, 0.3333333333333333703, 0.3333333333333333703, 0.3333333333333333703, 0.3333333333333333703, 0.3333333333333333703, 0.3333333333333333703, 0.3333333333333333703, 0.3333333333333333703, 0.3333333333333333703, 0.3333333333333333703, 0.3333333333333333703, 0.3333333333333333703, 0.3333333333333333703, 0.3333333333333333703, 0.3333333333333333703, 0.3333333333333333703, 0.3333333333333333703, 0.3333333333333333703, 0.3333333333333333703, 0.3333333333333333703, 0.3333333333333333703, 0.3333333333333333703, 0.3333333333333333703, 0.3333333333333333703, 0.3333333333333333703, 0.3333333333333333703, 0.3333333333333333703, 0.3333333333333333703, 0.3333333333333333703, 0.3333333333333333703, 0.3333333333333333703, 0.3333333333333333703, 0.3333333333333333703, 0.3333333333333333703, 0.3333333333333333703, 0.3333333333333333703, 0.3333333333333333703, 0.3333333333333333703, 0.3333333333333333703, 0.3333333333333333703, 0.3333333333333333703, 0.3333333333333333703, 0.3333333333333333703, 0.3333333333333333703, 0.3333333333333333703, 0.3333333333333333703, 0.3333333333333333703, 0.3333333333333333703, 0.3333333333333333703, 0.3333333333333333703, 0.3333333333333333703, 0.3333333333333333703, 0.3333333333333333703, 0.3333333333333333703, 0.3333333333333333703, 0.3333333333333333703, 0.3333333333333333703, 0.3333333333333333703, 0.3333333333333333703, 0.3333333333333333703, 0.3333333333333333703, 0.3333333333333333703, 0.3333333333333333703, 0.3333333333333333703, 0.3333333333333333703, 0.3333333333333333703, 0.3333333333333333703, 0.3333333333333333703, 0.3333333333333333703, 0.3333333333333333703, 0.3333333333333333703, 0.3333333333333333703, 0.3333333333333333703, 0.3333333333333333703, 0.3333333333333333703, 0.3333333333333333703, 0.3333333333333333703, 0.3333333333333333703, 0.3333333333333333703, 0.3333333333333333703, 0.3333333333333333703, 0.3333333333333333703, 0.3333333333333333703, 0.3333333333333333703, 0.3333333333333333703, 0.3333333333333333703, 0.3333333333333333703, 0.3333333333333333703, 0.3333333333333333703, 0.3333333333333333703, 0.3333333333333333703, 0.3333333333333333703, 0.3333333333333333703, 0.3333333333333333703, 0.3333333333333333703, 0.3333333333333333703, 0.3333333333333333703, 0.3333333333333333703, 0.3333333333333333703, 0.3333333333333333703, 0.3333333333333333703, 0.3333333333333333703, 0.3333333333333333703, 0.3333333333333333703, 0.3333333333333333703, 0.3333333333333333703, 0.3333333333333333703, 0.3333333333333333703, 0.3333333333333333703, 0.3333333333333333703, 0.3333333333333333703, 0.3333333333333333703, 0.3333333333333333703, 0.3333333333333333703, 0.3333333333333333703, 0.3333333333333333703, 0.3333333333333333703, 0.3333333333333333703, 0.3333333333333333703, 0.3333333333333333703, 0.3333333333333333703, 0.3333333333333333703, 0.3333333333333333703, 0.3333333333333333703, 0.3333333333333333703, 0.3333333333333333703, 0.3333333333333333703, 0.3333333333333333703, 0.3333333333333333703, 0.3333333333333333703, 0.3333333333333333703, 0.3333333333333333703, 0.3333333333333333703, 0.3333333333333333703, 0.3333333333333333703, 0.3333333333333333703, 0.3333333333333333703, 0.3333333333333333703, 0.3333333333333333703, 0.3333333333333333703, 0.3333333333333333703, 0.3333333333333333703, 0.3333333333333333703, 0.3333333333333333703, 0.3333333333333333703, 0.3333333333333333703, 0.3333333333333333703, 0.3333333333333333703, 0.3333333333333333703, 0.3333333333333333703, 0.3333333333333333703, 0.3333333333333333703, 0.3333333333333333703),
 ( 1.000000000000000000, 1.000000000000000000, 1.000000000000000000, 1.000000000000000000, 1.000000000000000000, 1.000000000000000000, 1.000000000000000000, 1.000000000000000000, 1.000000000000000000, 1.000000000000000000, 1.000000000000000000, 1.000000000000000000, 1.000000000000000000, 1.000000000000000000, 1.000000000000000000, 1.000000000000000000, 1.000000000000000000, 1.000000000000000000, 1.000000000000000000, 1.000000000000000000, 1.000000000000000000, 1.000000000000000000, 1.000000000000000000, 1.000000000000000000, 1.000000000000000000, 1.000000000000000000, 1.000000000000000000, 1.000000000000000000, 1.000000000000000000, 1.000000000000000000, 1.000000000000000000, 1.000000000000000000, 1.000000000000000000, 1.000000000000000000, 1.000000000000000000, 1.000000000000000000, 1.000000000000000000, 1.000000000000000000, 1.000000000000000000, 1.000000000000000000, 1.000000000000000000, 1.000000000000000000, 1.000000000000000000, 1.000000000000000000, 1.000000000000000000, 1.000000000000000000, 1.000000000000000000, 1.000000000000000000, 1.000000000000000000, 1.000000000000000000, 1.000000000000000000, 1.000000000000000000, 1.000000000000000000, 1.000000000000000000, 1.000000000000000000, 1.000000000000000000, 1.000000000000000000, 1.000000000000000000, 1.000000000000000000, 1.000000000000000000, 1.000000000000000000, 1.000000000000000000, 1.000000000000000000, 1.000000000000000000, 1.000000000000000000, 1.000000000000000000, 1.000000000000000000, 1.000000000000000000, 1.000000000000000000, 1.000000000000000000, 1.000000000000000000, 1.000000000000000000, 1.000000000000000000, 1.000000000000000000, 1.000000000000000000, 1.000000000000000000, 1.000000000000000000, 1.000000000000000000, 1.000000000000000000, 1.000000000000000000, 1.000000000000000000, 1.000000000000000000, 1.000000000000000000, 1.000000000000000000, 1.000000000000000000, 1.000000000000000000, 1.000000000000000000, 1.000000000000000000, 1.000000000000000000, 1.000000000000000000, 1.000000000000000000, 1.000000000000000000, 1.000000000000000000, 1.000000000000000000, 1.000000000000000000, 1.000000000000000000, 1.000000000000000000, 1.000000000000000000, 1.000000000000000000, 1.000000000000000000, 1.000000000000000000, 1.000000000000000000, 1.000000000000000000, 1.000000000000000000, 1.000000000000000000, 1.000000000000000000, 1.000000000000000000, 1.000000000000000000, 1.000000000000000000, 1.000000000000000000, 1.000000000000000000, 1.000000000000000000, 1.000000000000000000, 1.000000000000000000, 1.000000000000000000, 1.000000000000000000, 1.000000000000000000, 1.000000000000000000, 1.000000000000000000, 1.000000000000000000, 1.000000000000000000, 1.000000000000000000, 1.000000000000000000, 1.000000000000000000, 1.000000000000000000, 1.000000000000000000, 1.000000000000000000, 1.000000000000000000, 1.000000000000000000, 1.000000000000000000, 1.000000000000000000, 1.000000000000000000, 1.000000000000000000, 1.000000000000000000, 1.000000000000000000, 1.000000000000000000, 1.000000000000000000, 1.000000000000000000, 1.000000000000000000, 1.000000000000000000, 1.000000000000000000, 1.000000000000000000, 1.000000000000000000, 1.000000000000000000, 1.000000000000000000, 1.000000000000000000, 1.000000000000000000, 1.000000000000000000, 1.000000000000000000, 1.000000000000000000, 1.000000000000000000, 1.000000000000000000, 1.000000000000000000, 1.000000000000000000, 1.000000000000000000, 1.000000000000000000, 1.000000000000000000, 1.000000000000000000, 1.000000000000000000, 1.000000000000000000, 1.000000000000000000, 1.000000000000000000, 1.000000000000000000, 1.000000000000000000, 1.000000000000000000, 1.000000000000000000, 1.000000000000000000, 1.000000000000000000, 1.000000000000000000, 1.000000000000000000, 1.000000000000000000, 1.000000000000000000, 1.000000000000000000, 1.000000000000000000, 1.000000000000000000, 1.000000000000000000, 1.000000000000000000, 1.000000000000000000, 1.000000000000000000, 1.000000000000000000, 1.000000000000000000, 1.000000000000000000, 1.000000000000000000, 1.000000000000000000, 1.000000000000000000, 1.000000000000000000),
 ( 0.3333333333333333703, 0.3333333333333333703, 0.3333333333333333703, 0.3333333333333333703, 0.3333333333333333703, 0.3333333333333333703, 0.3333333333333333703, 0.3333333333333333703, 0.3333333333333333703, 0.3333333333333333703, 0.3333333333333333703, 0.3333333333333333703, 0.3333333333333333703, 0.3333333333333333703, 0.3333333333333333703, 0.3333333333333333703, 0.3333333333333333703, 0.3333333333333333703, 0.3333333333333333703, 0.3333333333333333703, 0.3333333333333333703, 0.3333333333333333703, 0.3333333333333333703, 0.3333333333333333703, 0.3333333333333333703, 0.3333333333333333703, 0.3333333333333333703, 0.3333333333333333703, 0.3333333333333333703, 0.3333333333333333703, 0.3333333333333333703, 0.3333333333333333703, 0.3333333333333333703, 0.3333333333333333703, 0.3333333333333333703, 0.3333333333333333703, 0.3333333333333333703, 0.3333333333333333703, 0.3333333333333333703, 0.3333333333333333703, 0.3333333333333333703, 0.3333333333333333703, 0.3333333333333333703, 0.3333333333333333703, 0.3333333333333333703, 0.3333333333333333703, 0.3333333333333333703, 0.3333333333333333703, 0.3333333333333333703, 0.3333333333333333703, 0.3333333333333333703, 0.3333333333333333703, 0.3333333333333333703, 0.3333333333333333703, 0.3333333333333333703, 0.3333333333333333703, 0.3333333333333333703, 0.3333333333333333703, 0.3333333333333333703, 0.3333333333333333703, 0.3333333333333333703, 0.3333333333333333703, 0.3333333333333333703, 0.3333333333333333703, 0.3333333333333333703, 0.3333333333333333703, 0.3333333333333333703, 0.3333333333333333703, 0.3333333333333333703, 0.3333333333333333703, 0.3333333333333333703, 0.3333333333333333703, 0.3333333333333333703, 0.3333333333333333703, 0.3333333333333333703, 0.3333333333333333703, 0.3333333333333333703, 0.3333333333333333703, 0.3333333333333333703, 0.3333333333333333703, 0.3333333333333333703, 0.3333333333333333703, 0.3333333333333333703, 0.3333333333333333703, 0.3333333333333333703, 0.3333333333333333703, 0.3333333333333333703, 0.3333333333333333703, 0.3333333333333333703, 0.3333333333333333703, 0.3333333333333333703, 0.3333333333333333703, 0.3333333333333333703, 0.3333333333333333703, 0.3333333333333333703, 0.3333333333333333703, 0.3333333333333333703, 0.3333333333333333703, 0.3333333333333333703, 0.3333333333333333703, 0.3333333333333333703, 0.3333333333333333703, 0.3333333333333333703, 0.3333333333333333703, 0.3333333333333333703, 0.3333333333333333703, 0.3333333333333333703, 0.3333333333333333703, 0.3333333333333333703, 0.3333333333333333703, 0.3333333333333333703, 0.3333333333333333703, 0.3333333333333333703, 0.3333333333333333703, 0.3333333333333333703, 0.3333333333333333703, 0.3333333333333333703, 0.3333333333333333703, 0.3333333333333333703, 0.3333333333333333703, 0.3333333333333333703, 0.3333333333333333703, 0.3333333333333333703, 0.3333333333333333703, 0.3333333333333333703, 0.3333333333333333703, 0.3333333333333333703, 0.3333333333333333703, 0.3333333333333333703, 0.3333333333333333703, 0.3333333333333333703, 0.3333333333333333703, 0.3333333333333333703, 0.3333333333333333703, 0.3333333333333333703, 0.3333333333333333703, 0.3333333333333333703, 0.3333333333333333703, 0.3333333333333333703, 0.3333333333333333703, 0.3333333333333333703, 0.3333333333333333703, 0.3333333333333333703, 0.3333333333333333703, 0.3333333333333333703, 0.3333333333333333703, 0.3333333333333333703, 0.3333333333333333703, 0.3333333333333333703, 0.3333333333333333703, 0.3333333333333333703, 0.3333333333333333703, 0.3333333333333333703, 0.3333333333333333703, 0.3333333333333333703, 0.3333333333333333703, 0.3333333333333333703, 0.3333333333333333703, 0.3333333333333333703, 0.3333333333333333703, 0.3333333333333333703, 0.3333333333333333703, 0.3333333333333333703, 0.3333333333333333703, 0.3333333333333333703, 0.3333333333333333703, 0.3333333333333333703, 0.3333333333333333703, 0.3333333333333333703, 0.3333333333333333703, 0.3333333333333333703, 0.3333333333333333703, 0.3333333333333333703, 0.3333333333333333703, 0.3333333333333333703, 0.3333333333333333703, 0.3333333333333333703, 0.3333333333333333703, 0.3333333333333333703, 0.3333333333333333703, 0.3333333333333333703, 0.3333333333333333703, 0.3333333333333333703, 0.3333333333333333703, 0.3333333333333333703, 0.3333333333333333703),
 ( 0.3333333333333333703, 0.3333333333333333703, 0.3333333333333333703, 0.3333333333333333703, 0.3333333333333333703, 0.3333333333333333703, 0.3333333333333333703, 0.3333333333333333703, 0.3333333333333333703, 0.3333333333333333703, 0.3333333333333333703, 0.3333333333333333703, 0.3333333333333333703, 0.3333333333333333703, 0.3333333333333333703, 0.3333333333333333703, 0.3333333333333333703, 0.3333333333333333703, 0.3333333333333333703, 0.3333333333333333703, 0.3333333333333333703, 0.3333333333333333703, 0.3333333333333333703, 0.3333333333333333703, 0.3333333333333333703, 0.3333333333333333703, 0.3333333333333333703, 0.3333333333333333703, 0.3333333333333333703, 0.3333333333333333703, 0.3333333333333333703, 0.3333333333333333703, 0.3333333333333333703, 0.3333333333333333703, 0.3333333333333333703, 0.3333333333333333703, 0.3333333333333333703, 0.3333333333333333703, 0.3333333333333333703, 0.3333333333333333703, 0.3333333333333333703, 0.3333333333333333703, 0.3333333333333333703, 0.3333333333333333703, 0.3333333333333333703, 0.3333333333333333703, 0.3333333333333333703, 0.3333333333333333703, 0.3333333333333333703, 0.3333333333333333703, 0.3333333333333333703, 0.3333333333333333703, 0.3333333333333333703, 0.3333333333333333703, 0.3333333333333333703, 0.3333333333333333703, 0.3333333333333333703, 0.3333333333333333703, 0.3333333333333333703, 0.3333333333333333703, 0.3333333333333333703, 0.3333333333333333703, 0.3333333333333333703, 0.3333333333333333703, 0.3333333333333333703, 0.3333333333333333703, 0.3333333333333333703, 0.3333333333333333703, 0.3333333333333333703, 0.3333333333333333703, 0.3333333333333333703, 0.3333333333333333703, 0.3333333333333333703, 0.3333333333333333703, 0.3333333333333333703, 0.3333333333333333703, 0.3333333333333333703, 0.3333333333333333703, 0.3333333333333333703, 0.3333333333333333703, 0.3333333333333333703, 0.3333333333333333703, 0.3333333333333333703, 0.3333333333333333703, 0.3333333333333333703, 0.3333333333333333703, 0.3333333333333333703, 0.3333333333333333703, 0.3333333333333333703, 0.3333333333333333703, 0.3333333333333333703, 0.3333333333333333703, 0.3333333333333333703, 0.3333333333333333703, 0.3333333333333333703, 0.3333333333333333703, 0.3333333333333333703, 0.3333333333333333703, 0.3333333333333333703, 0.3333333333333333703, 0.3333333333333333703, 0.3333333333333333703, 0.3333333333333333703, 0.3333333333333333703, 0.3333333333333333703, 0.3333333333333333703, 0.3333333333333333703, 0.3333333333333333703, 0.3333333333333333703, 0.3333333333333333703, 0.3333333333333333703, 0.3333333333333333703, 0.3333333333333333703, 0.3333333333333333703, 0.3333333333333333703, 0.3333333333333333703, 0.3333333333333333703, 0.3333333333333333703, 0.3333333333333333703, 0.3333333333333333703, 0.3333333333333333703, 0.3333333333333333703, 0.3333333333333333703, 0.3333333333333333703, 0.3333333333333333703, 0.3333333333333333703, 0.3333333333333333703, 0.3333333333333333703, 0.3333333333333333703, 0.3333333333333333703, 0.3333333333333333703, 0.3333333333333333703, 0.3333333333333333703, 0.3333333333333333703, 0.3333333333333333703, 0.3333333333333333703, 0.3333333333333333703, 0.3333333333333333703, 0.3333333333333333703, 0.3333333333333333703, 0.3333333333333333703, 0.3333333333333333703, 0.3333333333333333703, 0.3333333333333333703, 0.3333333333333333703, 0.3333333333333333703, 0.3333333333333333703, 0.3333333333333333703, 0.3333333333333333703, 0.3333333333333333703, 0.3333333333333333703, 0.3333333333333333703, 0.3333333333333333703, 0.3333333333333333703, 0.3333333333333333703, 0.3333333333333333703, 0.3333333333333333703, 0.3333333333333333703, 0.3333333333333333703, 0.3333333333333333703, 0.3333333333333333703, 0.3333333333333333703, 0.3333333333333333703, 0.3333333333333333703, 0.3333333333333333703, 0.3333333333333333703, 0.3333333333333333703, 0.3333333333333333703, 0.3333333333333333703, 0.3333333333333333703, 0.3333333333333333703, 0.3333333333333333703, 0.3333333333333333703, 0.3333333333333333703, 0.3333333333333333703, 0.3333333333333333703, 0.3333333333333333703, 0.3333333333333333703, 0.3333333333333333703, 0.3333333333333333703, 0.3333333333333333703, 0.3333333333333333703, 0.3333333333333333703, 0.3333333333333333703, 0.3333333333333333703, 0.3333333333333333703),
 ( 1.000000000000000000, 1.000000000000000000, 1.000000000000000000, 1.000000000000000000, 1.000000000000000000, 1.000000000000000000, 1.000000000000000000, 1.000000000000000000, 1.000000000000000000, 1.000000000000000000, 1.000000000000000000, 1.000000000000000000, 1.000000000000000000, 1.000000000000000000, 1.000000000000000000, 1.000000000000000000, 1.000000000000000000, 1.000000000000000000, 1.000000000000000000, 1.000000000000000000, 1.000000000000000000, 1.000000000000000000, 1.000000000000000000, 1.000000000000000000, 1.000000000000000000, 1.000000000000000000, 1.000000000000000000, 1.000000000000000000, 1.000000000000000000, 1.000000000000000000, 1.000000000000000000, 1.000000000000000000, 1.000000000000000000, 1.000000000000000000, 1.000000000000000000, 1.000000000000000000, 1.000000000000000000, 1.000000000000000000, 1.000000000000000000, 1.000000000000000000, 1.000000000000000000, 1.000000000000000000, 1.000000000000000000, 1.000000000000000000, 1.000000000000000000, 1.000000000000000000, 1.000000000000000000, 1.000000000000000000, 1.000000000000000000, 1.000000000000000000, 1.000000000000000000, 1.000000000000000000, 1.000000000000000000, 1.000000000000000000, 1.000000000000000000, 1.000000000000000000, 1.000000000000000000, 1.000000000000000000, 1.000000000000000000, 1.000000000000000000, 1.000000000000000000, 1.000000000000000000, 1.000000000000000000, 1.000000000000000000, 1.000000000000000000, 1.000000000000000000, 1.000000000000000000, 1.000000000000000000, 1.000000000000000000, 1.000000000000000000, 1.000000000000000000, 1.000000000000000000, 1.000000000000000000, 1.000000000000000000, 1.000000000000000000, 1.000000000000000000, 1.000000000000000000, 1.000000000000000000, 1.000000000000000000, 1.000000000000000000, 1.000000000000000000, 1.000000000000000000, 1.000000000000000000, 1.000000000000000000, 1.000000000000000000, 1.000000000000000000, 1.000000000000000000, 1.000000000000000000, 1.000000000000000000, 1.000000000000000000, 1.000000000000000000, 1.000000000000000000, 1.000000000000000000, 1.000000000000000000, 1.000000000000000000, 1.000000000000000000, 1.000000000000000000, 1.000000000000000000, 1.000000000000000000, 1.000000000000000000, 1.000000000000000000, 1.000000000000000000, 1.000000000000000000, 1.000000000000000000, 1.000000000000000000, 1.000000000000000000, 1.000000000000000000, 1.000000000000000000, 1.000000000000000000, 1.000000000000000000, 1.000000000000000000, 1.000000000000000000, 1.000000000000000000, 1.000000000000000000, 1.000000000000000000, 1.000000000000000000, 1.000000000000000000, 1.000000000000000000, 1.000000000000000000, 1.000000000000000000, 1.000000000000000000, 1.000000000000000000, 1.000000000000000000, 1.000000000000000000, 1.000000000000000000, 1.000000000000000000, 1.000000000000000000, 1.000000000000000000, 1.000000000000000000, 1.000000000000000000, 1.000000000000000000, 1.000000000000000000, 1.000000000000000000, 1.000000000000000000, 1.000000000000000000, 1.000000000000000000, 1.000000000000000000, 1.000000000000000000, 1.000000000000000000, 1.000000000000000000, 1.000000000000000000, 1.000000000000000000, 1.000000000000000000, 1.000000000000000000, 1.000000000000000000, 1.000000000000000000, 1.000000000000000000, 1.000000000000000000, 1.000000000000000000, 1.000000000000000000, 1.000000000000000000, 1.000000000000000000, 1.000000000000000000, 1.000000000000000000, 1.000000000000000000, 1.000000000000000000, 1.000000000000000000, 1.000000000000000000, 1.000000000000000000, 1.000000000000000000, 1.000000000000000000, 1.000000000000000000, 1.000000000000000000, 1.000000000000000000, 1.000000000000000000, 1.000000000000000000, 1.000000000000000000, 1.000000000000000000, 1.000000000000000000, 1.000000000000000000, 1.000000000000000000, 1.000000000000000000, 1.000000000000000000, 1.000000000000000000, 1.000000000000000000, 1.000000000000000000, 1.000000000000000000, 1.000000000000000000, 1.000000000000000000, 1.000000000000000000, 1.000000000000000000, 1.000000000000000000, 1.000000000000000000, 1.000000000000000000, 1.000000000000000000, 1.000000000000000000) ) ) 
 REPRESENTATION_ITEM ( '' )  SURFACE ( )  );
#15575=CARTESIAN_POINT ( 'NONE',  ( 12.77278825050581013, 8.691252192278360766, -14.91275796197543890 ) ) ;
#15577=CARTESIAN_POINT ( 'NONE',  ( 10.70135522441200671, 8.911701773272509897, -16.39640207298747754 ) ) ;
#15584=CARTESIAN_POINT ( 'NONE',  ( 10.35864918915110877, 16.97212501191939538, -17.92015940598198753 ) ) ;
#15585=CARTESIAN_POINT ( 'NONE',  ( 33.19592593216645326, -10.35933293216661610, -17.69446280125821147 ) ) ;
#15586=CARTESIAN_POINT ( 'NONE',  ( 24.92864811393110358, -0.2441600445015326137, -14.78813717129899885 ) ) ;
#15595=CARTESIAN_POINT ( 'NONE',  ( 24.16496757332932788, -10.42823604606268617, -16.34834267607407909 ) ) ;
#15596=CARTESIAN_POINT ( 'NONE',  ( 24.71165717419137309, -6.805198111665588634, -19.34662478563667065 ) ) ;
#15607=CARTESIAN_POINT ( 'NONE',  ( 11.21589157578718421, 9.127945497600544300, -17.24491392235805876 ) ) ;
#15608=CARTESIAN_POINT ( 'NONE',  ( 10.33811693838771717, 18.38618951776012267, -23.00000000000000711 ) ) ;
#15616=CARTESIAN_POINT ( 'NONE',  ( 9.641384570184822422, 17.66873631484086715, -17.89388817125738385 ) ) ;
#15620=CARTESIAN_POINT ( 'NONE',  ( 21.94319337455657859, -4.318501116253552041, -18.82930321547734920 ) ) ;
#15624=CARTESIAN_POINT ( 'NONE',  ( 12.24596961785936777, 9.516471373605908113, -15.33264171117454744 ) ) ;
#15625=CARTESIAN_POINT ( 'NONE',  ( 33.09970432537804896, -11.76965169494800989, -17.65272085910585886 ) ) ;
#15627=CARTESIAN_POINT ( 'NONE',  ( 23.63863231746517712, -2.790269051896475450, -19.68844555248840678 ) ) ;
#15629=CARTESIAN_POINT ( 'NONE',  ( 21.15397186503396654, -1.756306506132798706, -15.01670888948634364 ) ) ;
#15635=CARTESIAN_POINT ( 'NONE',  ( 16.36264732604271899, 7.873549196589271659, -20.78255227469630739 ) ) ;
#15636=CARTESIAN_POINT ( 'NONE',  ( 26.70980024742295456, -9.230482666323300833, -19.13350686062700134 ) ) ;
#15639=CARTESIAN_POINT ( 'NONE',  ( 29.22485947447185595, -8.910266539455653501, -18.36689805200119707 ) ) ;
#15643=MECHANICAL_DESIGN_GEOMETRIC_PRESENTATION_REPRESENTATION('',(#14170),#20518);
#15647=CARTESIAN_POINT ( 'NONE',  ( 9.641350810849047548, 17.66889113945805789, -17.94384837343789485 ) ) ;
#15648=CARTESIAN_POINT ( 'NONE',  ( 24.01829950071418907, -5.359185124211399476, -18.14381017295562160 ) ) ;
#15649=CARTESIAN_POINT ( 'NONE',  ( 17.46151185945609186, 6.859213057953727599, -13.86392132274949418 ) ) ;
#15651=CARTESIAN_POINT ( 'NONE',  ( 32.82219004228267778, -9.671386367997632405, -18.62901690529166743 ) ) ;
#15654=CARTESIAN_POINT ( 'NONE',  ( 11.47652547240386944, 9.253065934422213701, -15.85936358228339316 ) ) ;
#15657=CARTESIAN_POINT ( 'NONE',  ( 9.661883061612440926, 16.25482663361732705, -17.92981046679734547 ) ) ;
#15660=CARTESIAN_POINT ( 'NONE',  ( 10.33811693838771717, 18.38618951776012267, -17.95086732675816776 ) ) ;
#15664=FACE_OUTER_BOUND ( 'NONE', #25279, .T. ) ;
#15667=CARTESIAN_POINT ( 'NONE',  ( 13.37841584274036855, 7.625425322794393779, -15.70882597216490240 ) ) ;
#15668=CARTESIAN_POINT ( 'NONE',  ( 31.92618181579182135, -10.29178896789921893, -18.33933693937521880 ) ) ;
#15669=CARTESIAN_POINT ( 'NONE',  ( 18.04051923446642292, -0.4597542321540471488, -16.60176153622942508 ) ) ;
#15670=CARTESIAN_POINT ( 'NONE',  ( 26.95082352492110189, -12.40836276091286194, -17.97502949936508898 ) ) ;
#15673=CARTESIAN_POINT ( 'NONE',  ( 19.28943675834911531, -1.002762487816046155, -14.40755329178536037 ) ) ;
#15681=ADVANCED_BREP_SHAPE_REPRESENTATION ( '', ( #1479, #13190 ), #21465 ) ;
#15685=CARTESIAN_POINT ( 'NONE',  ( 35.50545599541538877, -20.99072003637593653, -18.92103158260024642 ) ) ;
#15687=CARTESIAN_POINT ( 'NONE',  ( 10.64844024921564092, 9.137493944846720950, -16.41957189434499753 ) ) ;
#15690=CARTESIAN_POINT ( 'NONE',  ( 29.62588713853392264, -10.65184931322849060, -12.76488833982454629 ) ) ;
#15692=CARTESIAN_POINT ( 'NONE',  ( 10.35864924400752862, 16.97212476034085782, -17.91519562840587199 ) ) ;
#15696=CARTESIAN_POINT ( 'NONE',  ( 16.84948243412402036, 10.49281628697410262, -11.66356073909478575 ) ) ;
#15702=CARTESIAN_POINT ( 'NONE',  ( 9.661883061612440926, 16.25482663361732705, -17.91928203681695564 ) ) ;
#15703=CARTESIAN_POINT ( 'NONE',  ( 18.26079443319284934, -0.1287745640203900310, -14.06839115638798354 ) ) ;
#15704=CARTESIAN_POINT ( 'NONE',  ( 19.20998527735078198, 1.665648160765265784, -20.80323043525838855 ) ) ;
#15708=CARTESIAN_POINT ( 'NONE',  ( 20.72626264887238534, -1.914771856900582714, -13.62749948506543518 ) ) ;
#15714=CARTESIAN_POINT ( 'NONE',  ( 10.46817501828509123, 16.46982559821503145, -17.33665662920367723 ) ) ;
#15723=CARTESIAN_POINT ( 'NONE',  ( 19.05868480923028940, 8.129737193291200370, -16.02886444249750042 ) ) ;
#15724=CARTESIAN_POINT ( 'NONE',  ( 12.24513942169458858, 9.516104476910269838, -15.33330339355663519 ) ) ;
#15725=CARTESIAN_POINT ( 'NONE',  ( 35.54287943964028784, -22.15884374752674546, -18.65915260879160797 ) ) ;
#15728=CARTESIAN_POINT ( 'NONE',  ( 12.75280283744833376, 7.624395256242640251, -14.92868632776139037 ) ) ;
#15734=CARTESIAN_POINT ( 'NONE',  ( 12.90243451339205194, 9.531139938431367753, -16.08819151157827321 ) ) ;
#15735=CARTESIAN_POINT ( 'NONE',  ( 33.07549275714919901, -10.34104163876563831, -17.35407900654646340 ) ) ;
#15736=CARTESIAN_POINT ( 'NONE',  ( 19.83745040964868522, -2.306422872736943575, -14.39351019504378293 ) ) ;
#15742=CARTESIAN_POINT ( 'NONE',  ( 30.78125299044525320, -8.317598597646391312, -16.28273480984023891 ) ) ;
#15743=CARTESIAN_POINT ( 'NONE',  ( 24.28190956353967422, -4.127413435877471670, -12.52835809790152766 ) ) ;
#15750=AXIS2_PLACEMENT_3D ( 'NONE', #14838, #828, #9822 ) ;
#15751=CARTESIAN_POINT ( 'NONE',  ( 11.09431937732777129, 9.685491096586417825, -17.29518830297554643 ) ) ;
#15754=CARTESIAN_POINT ( 'NONE',  ( 12.50035968906703765, 8.570861208087439564, -15.12988832871674560 ) ) ;
#15756=CARTESIAN_POINT ( 'NONE',  ( 27.62103240953636174, -12.62788667074165794, -13.46147607715242245 ) ) ;
#15762=CARTESIAN_POINT ( 'NONE',  ( 18.98827506421364575, 7.203492520304279445, -17.17051369180543929 ) ) ;
#15765=CARTESIAN_POINT ( 'NONE',  ( 23.11440248821028831, -7.346120041196752659, -16.32852059634029018 ) ) ;
#15769=CARTESIAN_POINT ( 'NONE',  ( 12.24552273913795730, 9.516269270964150095, -15.33299823368393078 ) ) ;
#15770=CARTESIAN_POINT ( 'NONE',  ( 34.82539348385352440, -18.93555941106099993, -20.13934242161363741 ) ) ;
#15772=CARTESIAN_POINT ( 'NONE',  ( 25.97256211245905533, -8.171536508395311316, -18.54953510021574559 ) ) ;
#15774=CARTESIAN_POINT ( 'NONE',  ( 25.36902537161520499, -2.228419832982303728, -15.31576610616191481 ) ) ;
#15776=CARTESIAN_POINT ( 'NONE',  ( 10.35864918915111055, 16.97212501191939182, -23.00000000000000711 ) ) ;
#15777=SHAPE_REPRESENTATION_RELATIONSHIP ( 'NONE' , 'NONE' ,  #22819, #15681 ) ;
#15778=CARTESIAN_POINT ( 'NONE',  ( 29.60951380729897764, -9.700310021160106544, -19.83312561509874783 ) ) ;
#15779=CARTESIAN_POINT ( 'NONE',  ( 29.51995068812739476, -6.211492405346085377, -16.93985997890334261 ) ) ;
#15792=CARTESIAN_POINT ( 'NONE',  ( 24.01770293978927384, -9.123702295727731837, -14.45939194930751448 ) ) ;
#15793=CARTESIAN_POINT ( 'NONE',  ( 20.51209521231993094, 3.083376493849706801, -19.38174501956431683 ) ) ;
#15794=CARTESIAN_POINT ( 'NONE',  ( 33.89278150306358128, -11.43586942258664507, -20.72336631513872973 ) ) ;
#15796=CARTESIAN_POINT ( 'NONE',  ( 12.50035968906703765, 8.570861208087439564, -15.12988832871674560 ) ) ;
#15800=CARTESIAN_POINT ( 'NONE',  ( 9.797549260427590667, 15.63264415243319938, -17.83144836289601898 ) ) ;
#15804=CARTESIAN_POINT ( 'NONE',  ( 12.29195110325218288, 8.516770644378290456, -15.29309475950548958 ) ) ;
#15812=CARTESIAN_POINT ( 'NONE',  ( 13.59703899429919005, 7.722038565090276308, -15.53457947969411634 ) ) ;
#15813=CARTESIAN_POINT ( 'NONE',  ( 35.41344336761681433, -22.57735604011907071, -20.16400759377322061 ) ) ;
#15814=CARTESIAN_POINT ( 'NONE',  ( 18.41232452102509143, -0.3525767977158695277, -15.58598945151665305 ) ) ;
#15815=CARTESIAN_POINT ( 'NONE',  ( 17.64917075666736679, 6.165203978315560995, -14.56523922633501655 ) ) ;
#15817=CARTESIAN_POINT ( 'NONE',  ( 21.04533358917985808, -3.575919577149618167, -19.74844908412899969 ) ) ;
#15818=EDGE_CURVE ( 'NONE', #8937, #3493, #937, .T. ) ;
#15827=CARTESIAN_POINT ( 'NONE',  ( 35.15837367389831769, -19.43146302041509443, -19.19767279675701488 ) ) ;
#15829=CARTESIAN_POINT ( 'NONE',  ( 10.66059746906157635, 9.081739384948186000, -16.41454445628326297 ) ) ;
#15833=CARTESIAN_POINT ( 'NONE',  ( 11.76876341733043141, 10.50516141373230106, -16.79855566342228101 ) ) ;
#15844=ORIENTED_EDGE ( 'NONE', *, *, #2983, .F. ) ;
#15845=CARTESIAN_POINT ( 'NONE',  ( 13.12723341905928898, 8.572452836447732594, -15.90902281579132449 ) ) ;
#15847=CARTESIAN_POINT ( 'NONE',  ( 24.59799960276797393, -1.134526835705675918, -15.12159415400816975 ) ) ;
#15848=CARTESIAN_POINT ( 'NONE',  ( 22.87580194831562252, -0.07614860672512525908, -19.74465839296685132 ) ) ;
#15849=CARTESIAN_POINT ( 'NONE',  ( 21.92441584138004984, 2.204866226087792924, -14.79409581392398110 ) ) ;
#15855=CARTESIAN_POINT ( 'NONE',  ( 21.42923412144385509, -1.598955984811285536, -13.33006947543598741 ) ) ;
#15862=CARTESIAN_POINT ( 'NONE',  ( 35.54859390953724585, -22.18451583373416014, -17.22552805718784441 ) ) ;
#15867=CARTESIAN_POINT ( 'NONE',  ( 19.25048709941964376, 7.441878894999256921, -18.84525011105569803 ) ) ;
#15868=CARTESIAN_POINT ( 'NONE',  ( 12.24619727527933222, 9.516571979449480523, -15.33246026419563890 ) ) ;
#15869=CARTESIAN_POINT ( 'NONE',  ( 35.53434814243864537, -22.12051714835155281, -18.84852710552948096 ) ) ;
#15873=CARTESIAN_POINT ( 'NONE',  ( 9.641350810849047548, 17.66889113945805789, -17.91796598306941135 ) ) ;
#15879=CARTESIAN_POINT ( 'NONE',  ( 12.86837137031974621, 9.516086858917468305, -16.11534043535873906 ) ) ;
#15881=CARTESIAN_POINT ( 'NONE',  ( 33.16581763841239194, -10.35476010881584052, -17.60936685258081624 ) ) ;
#15882=CARTESIAN_POINT ( 'NONE',  ( 24.78692427941192733, -9.284778175067517125, -17.23615439686343720 ) ) ;
#15890=CARTESIAN_POINT ( 'NONE',  ( 30.02037170576755187, -9.505783518442527225, -18.49971606337314967 ) ) ;
#15892=CARTESIAN_POINT ( 'NONE',  ( 27.68339325353806046, -3.782361434017075474, -17.87574284786517964 ) ) ;
#15903=CARTESIAN_POINT ( 'NONE',  ( 12.49860086554322436, 8.570087612320898884, -15.13128986298120537 ) ) ;
#15908=CARTESIAN_POINT ( 'NONE',  ( 18.11961939296043056, 8.971021047410516758, -18.23824686698257125 ) ) ;
#15911=CARTESIAN_POINT ( 'NONE',  ( 25.45462155318426767, -0.2439708902934435431, -15.99927030562601438 ) ) ;
#15915=CARTESIAN_POINT ( 'NONE',  ( 12.31319128649213646, 9.546177831575306527, -15.27906485473354792 ) ) ;
#15918=CARTESIAN_POINT ( 'NONE',  ( 34.11209566957792561, -15.73109017586260272, -19.92372960426217787 ) ) ;
#15920=CARTESIAN_POINT ( 'NONE',  ( 28.12266609392075267, -5.599633216697744942, -16.00068813756295327 ) ) ;
#15922=CARTESIAN_POINT ( 'NONE',  ( 25.85951265464835203, -2.375871015539448461, -16.96122936427994787 ) ) ;
#15925=CARTESIAN_POINT ( 'NONE',  ( 30.28288205714520132, -11.65814127372701670, -12.00898047443557459 ) ) ;
#15927=CARTESIAN_POINT ( 'NONE',  ( 27.75006011364712322, -11.91879133414019698, -17.49150313904273801 ) ) ;
#15943=CARTESIAN_POINT ( 'NONE',  ( 24.94059380785660451, 0.5691772567322460619, -14.01379559947946518 ) ) ;
#15944=CARTESIAN_POINT ( 'NONE',  ( 16.54288150113237066, 3.399532473721276649, -19.15960874834559746 ) ) ;
#15945=CARTESIAN_POINT ( 'NONE',  ( 31.73602415849877900, -9.487789691486469223, -15.56998832973926916 ) ) ;
#15947=CARTESIAN_POINT ( 'NONE',  ( 12.07641845611955489, 8.540206757827041528, -15.45582622123028216 ) ) ;
#15950=CARTESIAN_POINT ( 'NONE',  ( 9.688134281814004822, 16.13443519152062677, -17.87669530545171881 ) ) ;
#15954=CARTESIAN_POINT ( 'NONE',  ( 12.49977518293622758, 8.570603418560722275, -15.13035415120363325 ) ) ;
#15961=CARTESIAN_POINT ( 'NONE',  ( 9.112637166705713554, 16.18088265059586561, -17.05468042929993189 ) ) ;
#15962=CARTESIAN_POINT ( 'NONE',  ( 35.54750751241274287, -23.17963522693337453, -18.53372063443203999 ) ) ;
#15964=CARTESIAN_POINT ( 'NONE',  ( 20.66677465483945397, 4.408179161683285052, -13.64328152160912033 ) ) ;
#15966=CARTESIAN_POINT ( 'NONE',  ( 15.71409287621466788, 5.292507472020409942, -15.15310296786427635 ) ) ;
#15972=CARTESIAN_POINT ( 'NONE',  ( 22.17025134254096130, -8.444422103036636429, -16.38876926059057126 ) ) ;
#15981=CARTESIAN_POINT ( 'NONE',  ( 34.62340031318386480, -17.02811109401968181, -19.03596318374462726 ) ) ;
#15982=CARTESIAN_POINT ( 'NONE',  ( 12.65299103417153681, 7.585129394224154886, -15.00786874580416530 ) ) ;
#15985=CARTESIAN_POINT ( 'NONE',  ( 26.72610680620850232, -7.491537437428757329, -18.63066883040512067 ) ) ;
#15987=CARTESIAN_POINT ( 'NONE',  ( 10.47151541139924547, 16.45450612959241354, -17.33501744001014444 ) ) ;
#15999=CARTESIAN_POINT ( 'NONE',  ( 10.89980385979276356, 10.57756405496316710, -17.37562731196375410 ) ) ;
#16000=CARTESIAN_POINT ( 'NONE',  ( 20.06573045921589227, -2.681363122285017386, -18.07621394912722934 ) ) ;
#16001=CARTESIAN_POINT ( 'NONE',  ( 24.51656338950621361, -2.114370418465405521, -18.20187689272319176 ) ) ;
#16002=CARTESIAN_POINT ( 'NONE',  ( 19.23896461120675383, 4.098237937441782996, -14.15247350351863886 ) ) ;
#16008=CARTESIAN_POINT ( 'NONE',  ( 21.48529164538665981, 5.106035544247377267, -18.65531623833433628 ) ) ;
#16014=CARTESIAN_POINT ( 'NONE',  ( 10.35864918915110877, 16.97212501191939538, -19.66666666666842644 ) ) ;
#16020=CARTESIAN_POINT ( 'NONE',  ( 19.11618317516819587, 7.271703427217982352, -19.10559232466456692 ) ) ;
#16021=CARTESIAN_POINT ( 'NONE',  ( 11.28421916535349112, 16.64009977454265865, -16.78120545242191142 ) ) ;
#16026=CARTESIAN_POINT ( 'NONE',  ( 9.879812780108833792, 16.57527415160161510, -16.52987074417163527 ) ) ;
#16028=CARTESIAN_POINT ( 'NONE',  ( 9.641485839925177714, 17.66827187890266160, -17.87200850766020110 ) ) ;
#16033=CARTESIAN_POINT ( 'NONE',  ( 13.00452062571394229, 9.576253617860157163, -16.00682707811506233 ) ) ;
#16035=CARTESIAN_POINT ( 'NONE',  ( 35.34711162051457478, -16.78689235204268115, -20.22678452305727603 ) ) ;
#16036=CARTESIAN_POINT ( 'NONE',  ( 24.18219217278060995, -6.970120066757704791, -14.18070892486464629 ) ) ;
#16042=CARTESIAN_POINT ( 'NONE',  ( 14.93998017692337221, 5.301442995092576105, -18.84457556472494488 ) ) ;
#16043=CARTESIAN_POINT ( 'NONE',  ( 21.03482577225312156, -5.582666113748667058, -14.36824825895596014 ) ) ;
#16051=CARTESIAN_POINT ( 'NONE',  ( 10.33931768503335924, 18.38068274058360885, -17.76381606660089929 ) ) ;
#16053=CARTESIAN_POINT ( 'NONE',  ( 31.88113401528661939, -11.03952345999570994, -14.96145667752709763 ) ) ;
#16059=CARTESIAN_POINT ( 'NONE',  ( 9.826288910175632552, 16.82074144182198694, -16.60662094963572244 ) ) ;
#16061=CARTESIAN_POINT ( 'NONE',  ( 28.05683000375443825, -12.20169833507544865, -14.26034257730772126 ) ) ;
#16069=CARTESIAN_POINT ( 'NONE',  ( 12.24830724310059082, 9.517209185634078139, -15.33080109912759070 ) ) ;
#16070=CARTESIAN_POINT ( 'NONE',  ( 35.54787733059053778, -22.18129662410796854, -18.46719521006932396 ) ) ;
#16073=CARTESIAN_POINT ( 'NONE',  ( 20.31058213454123162, -2.053861134507735109, -16.68646832148754200 ) ) ;
#16079=CARTESIAN_POINT ( 'NONE',  ( 18.68520274485960542, 10.62608585526774441, -17.78552708330943588 ) ) ;
#16080=CARTESIAN_POINT ( 'NONE',  ( 28.61400761516875590, -9.413816014945153299, -13.42719155385534080 ) ) ;
#16092=CARTESIAN_POINT ( 'NONE',  ( 25.07632161252335123, -1.101686516974712315, -19.85338880782979132 ) ) ;
#16093=CARTESIAN_POINT ( 'NONE',  ( 19.23896461120675383, 4.098237937441782996, -14.15247350351863886 ) ) ;
#16095=CARTESIAN_POINT ( 'NONE',  ( 31.38423252821215570, -10.20947814759437655, -16.80760986317607930 ) ) ;
#16098=CARTESIAN_POINT ( 'NONE',  ( 11.51951884677450266, 9.108496074915260365, -15.83757232928968683 ) ) ;
#16108=CARTESIAN_POINT ( 'NONE',  ( 12.50016782010997751, 8.570776461014483871, -15.13004124836345632 ) ) ;
#16115=CARTESIAN_POINT ( 'NONE',  ( 9.115110896146415342, 16.16953781205366170, -17.05365751988364309 ) ) ;
#16116=CARTESIAN_POINT ( 'NONE',  ( 33.08402606333302742, -12.15068820457383403, -20.63309441556253176 ) ) ;
#16118=CARTESIAN_POINT ( 'NONE',  ( 14.32916401545863039, 6.225515681311286187, -14.04012878508491369 ) ) ;
#16120=CARTESIAN_POINT ( 'NONE',  ( 19.26077778332419044, 5.765437233969479713, -18.81236659294151892 ) ) ;
#16122=CARTESIAN_POINT ( 'NONE',  ( 18.61935276534875783, -1.259532457306228315, -15.72749031817820331 ) ) ;
#16132=CARTESIAN_POINT ( 'NONE',  ( 34.49426285277334614, -12.00696374527110066, -18.89673795385250799 ) ) ;
#16134=CARTESIAN_POINT ( 'NONE',  ( 11.57911078346310774, 7.697743364462890980, -15.81898674067912225 ) ) ;
#16141=CARTESIAN_POINT ( 'NONE',  ( 10.38089682401341385, 16.87009452252716102, -17.57504515238516873 ) ) ;
#16151=CARTESIAN_POINT ( 'NONE',  ( 9.667859621686535121, 16.22741736728331929, -17.88507964468380251 ) ) ;
#16152=CARTESIAN_POINT ( 'NONE',  ( 17.03934835405440751, -0.5873649402599611102, -16.44458879923593742 ) ) ;
#16153=CARTESIAN_POINT ( 'NONE',  ( 22.62754675296084983, -4.373583220233932423, -15.05708262856468060 ) ) ;
#16154=CARTESIAN_POINT ( 'NONE',  ( 16.12927480167980576, 2.990883400875756326, -18.25071113400840517 ) ) ;
#16159=CARTESIAN_POINT ( 'NONE',  ( 23.56138260001205964, -6.829566487537672259, -18.05074380722902916 ) ) ;
#16168=CARTESIAN_POINT ( 'NONE',  ( 10.36430886937160167, 16.94616899698690204, -17.73806594831300032 ) ) ;
#16173=ADVANCED_FACE ( 'NONE', ( #7163 ), #28257, .T. ) ;
#16176=CARTESIAN_POINT ( 'NONE',  ( 17.63704213852533442, 9.806822523219006271, -18.50018230520716145 ) ) ;
#16177=CARTESIAN_POINT ( 'NONE',  ( 11.05558847800967648, 17.68862925033535660, -17.87192865789842955 ) ) ;
#16178=CARTESIAN_POINT ( 'NONE',  ( 35.54859390953724585, -22.18451583373416014, -17.78191007148576475 ) ) ;
#16183=CARTESIAN_POINT ( 'NONE',  ( 9.907423389235603395, 16.44864837861227969, -16.50891839478055090 ) ) ;
#16184=CARTESIAN_POINT ( 'NONE',  ( 12.82404076521984670, 7.655871835264917102, -14.87190880308183871 ) ) ;
#16191=CARTESIAN_POINT ( 'NONE',  ( 10.36007019289729847, 16.96560810760319882, -17.82599398985513872 ) ) ;
#16192=CARTESIAN_POINT ( 'NONE',  ( 31.87116100697361887, -10.15812870475309815, -13.95024105943860171 ) ) ;
#16193=CARTESIAN_POINT ( 'NONE',  ( 25.04068920418659161, -5.475481712173364990, -18.92835678451453774 ) ) ;
#16199=CARTESIAN_POINT ( 'NONE',  ( 18.45234147263269620, 6.489596213788811241, -14.85506563039705519 ) ) ;
#16200=CARTESIAN_POINT ( 'NONE',  ( 21.56333733550986409, -5.354713294276967517, -13.65854400988971484 ) ) ;
#16210=CARTESIAN_POINT ( 'NONE',  ( 10.71436926824426550, 16.66064837202128501, -15.95707641581892133 ) ) ;
#16215=CARTESIAN_POINT ( 'NONE',  ( 9.926830210242822972, 16.35964622367879784, -16.50025672554925293 ) ) ;
#16217=CARTESIAN_POINT ( 'NONE',  ( 18.67591552545227174, 7.243412299697878254, -16.30691131850022657 ) ) ;
#16220=CARTESIAN_POINT ( 'NONE',  ( 31.22280883588763700, -10.09333740185288875, -13.86128061636125786 ) ) ;
#16224=CARTESIAN_POINT ( 'NONE',  ( 11.31663841827600692, 16.49142094814642334, -16.76779895092377615 ) ) ;
#16226=CARTESIAN_POINT ( 'NONE',  ( 35.52583876341286384, -22.08228901593173177, -18.97221062538168113 ) ) ;
#16230=CARTESIAN_POINT ( 'NONE',  ( 23.96437976099892708, -9.208260125601851698, -18.67152130837153123 ) ) ;
#16233=CARTESIAN_POINT ( 'NONE',  ( 20.13607245741800611, 4.456688099076253629, -14.49627829575511129 ) ) ;
#16234=CARTESIAN_POINT ( 'NONE',  ( 25.85465836959373220, -10.01954208144345770, -18.53069695322523103 ) ) ;
#16243=CARTESIAN_POINT ( 'NONE',  ( 9.644802874473198173, 17.65305953564175567, -17.69767226479352118 ) ) ;
#16244=CARTESIAN_POINT ( 'NONE',  ( 20.36141319467227362, -5.793038086071195636, -16.11598603859005507 ) ) ;
#16245=CARTESIAN_POINT ( 'NONE',  ( 21.81760893248375766, -3.923850722439390815, -13.93537712798182682 ) ) ;
#16246=CARTESIAN_POINT ( 'NONE',  ( 32.41494245136814811, -10.61148775487728813, -19.57799680467864789 ) ) ;
#16251=CARTESIAN_POINT ( 'NONE',  ( 13.77718166750865869, 8.859676595473324312, -15.39100258941132182 ) ) ;
#16254=CARTESIAN_POINT ( 'NONE',  ( 10.33811693838771717, 18.38618951776012267, -17.93331994345748726 ) ) ;
#16258=CARTESIAN_POINT ( 'NONE',  ( 15.94478687392618355, 4.193953704849600506, -19.05305658475056063 ) ) ;
#16261=CARTESIAN_POINT ( 'NONE',  ( 34.31408884023914396, -17.63853849290766362, -21.02710884213126263 ) ) ;
#16263=CARTESIAN_POINT ( 'NONE',  ( 22.68669718693540105, -3.283095500849226411, -14.44170700164887933 ) ) ;
#16264=CARTESIAN_POINT ( 'NONE',  ( 16.70639138691818459, 6.939553047386250562, -20.38695695975560085 ) ) ;
#16266=CARTESIAN_POINT ( 'NONE',  ( 19.83814782303322133, -0.7621604502531613701, -13.87429439740111370 ) ) ;
#16278=CARTESIAN_POINT ( 'NONE',  ( 33.01527616964045109, -10.33189599206409959, -17.18388710919138873 ) ) ;
#16279=CARTESIAN_POINT ( 'NONE',  ( 9.641350829061996919, 17.66889105593114806, -17.91548090047172437 ) ) ;
#16284=CARTESIAN_POINT ( 'NONE',  ( 10.35953768210033665, 16.96805026999784616, -17.84385765891457254 ) ) ;
#16293=CARTESIAN_POINT ( 'NONE',  ( 9.666872068725954392, 16.23194641104447911, -17.88584179299332533 ) ) ;
#16295=CARTESIAN_POINT ( 'NONE',  ( 16.98604603105943767, -0.4850832133139416080, -17.48051239862526884 ) ) ;
#16296=CARTESIAN_POINT ( 'NONE',  ( 21.05341046998850629, -2.558799731849103587, -14.42238450910079806 ) ) ;
#16298=CARTESIAN_POINT ( 'NONE',  ( 20.38603433104324480, 7.363110203939331022, -17.91596102798271062 ) ) ;
#16303=CARTESIAN_POINT ( 'NONE',  ( 22.97938783112199701, -3.359759438970757017, -19.62490732200095067 ) ) ;
#16313=CARTESIAN_POINT ( 'NONE',  ( 10.35864918915110877, 16.97212501191939538, -17.92015940598198753 ) ) ;
#16315=CARTESIAN_POINT ( 'NONE',  ( 33.41663030065195272, -12.60673267154789201, -19.71350710734569134 ) ) ;
#16317=CARTESIAN_POINT ( 'NONE',  ( 11.96143972814086531, 7.837808674300617007, -16.77422427047595477 ) ) ;
#16321=CARTESIAN_POINT ( 'NONE',  ( 20.50636976340433293, -0.9757509181830721356, -19.91080244439677571 ) ) ;
#16322=CARTESIAN_POINT ( 'NONE',  ( 11.16343636398553052, 17.19402509784177369, -16.95964061678045454 ) ) ;
#16327=CARTESIAN_POINT ( 'NONE',  ( 9.905109554012803130, 16.45925992188944420, -16.51025697316969953 ) ) ;
#16329=CARTESIAN_POINT ( 'NONE',  ( 9.641350810849047548, 17.66889113945805789, -17.92981046679734547 ) ) ;
#16335=CARTESIAN_POINT ( 'NONE',  ( 10.49225533350670858, 16.35939020308235925, -17.32643665990597981 ) ) ;
#16337=CARTESIAN_POINT ( 'NONE',  ( 36.54859590101256828, -22.18452478037840336, -18.26685560724362034 ) ) ;
#16338=CARTESIAN_POINT ( 'NONE',  ( 25.67262840375075328, -3.322766148301121714, -14.04542551033457798 ) ) ;
#16340=CARTESIAN_POINT ( 'NONE',  ( 34.43765690731135720, -12.70119407716533111, -19.95187818093482335 ) ) ;
#16342=CARTESIAN_POINT ( 'NONE',  ( 14.82995595102070752, 5.192148136363496036, -18.54057990209784634 ) ) ;
#16343=CARTESIAN_POINT ( 'NONE',  ( 26.72351632055398696, -11.69804524575189397, -15.34103589027250791 ) ) ;
#16346=B_SPLINE_CURVE_WITH_KNOTS ( 'NONE', 3,
 ( #1328, #17191, #6202, #19472, #8332, #17331, #15495, #17635, #13057, #22077, #24224, #12446, #28845, #26518, #26990, #3176, #6048, #15337, #14878, #3324, #12603, #26677, #5754, #15036, #24368, #19765, #29134, #6650, #27744, #29763, #30205, #13798, #1636, #9214, #27449, #20821, #15649, #4210, #1939, #13358, #9064, #8772, #27302, #6356, #18389, #11505, #18087, #22683, #3914, #1784, #25271, #11069, #22834, #15944, #4357, #23124, #13660, #22984, #6502, #24982, #20224, #6804, #29610, #2233, #10915, #16093, #18541, #27895, #29911, #30054, #22538, #20373, #2087, #18234, #6957, #8626, #24826, #25420, #15793, #11221, #17926, #25120, #4509, #13507, #11363, #13214, #4065, #20524, #8918, #27592, #20667, #4804, #14248, #9829, #19145, #26032, #7256, #687, #16854, #25879, #18697, #9974, #28502, #21277, #11813, #9366, #2543, #21588, #21128, #18839, #28355, #23430, #28042, #389, #28200, #7550, #23579, #240, #7098, #2675, #13944, #23738, #7411, #16398, #9517, #19289, #11662, #25721, #14550, #14097, #16555, #4958, #2835, #5262, #11961, #9675, #18997, #26181, #20976, #23897, #2389, #12121, #21436, #28645, #16711, #5106, #14396, #547, #2994, #12269, #16245, #25557, #4652, #23274, #85, #12868, #22181, #26485, #10580, #7991, #15150, #20047, #1291, #8140, #21732, #26954, #19586, #17156, #835, #22340, #3427, #22040, #17299, #7696, #10424, #1144, #26638, #1443, #19887, #12718, #3289, #19733, #12416, #10126, #17009, #15000, #15298, #5565, #5720, #6011, #13024, #24334, #29101, #14700, #7847, #24630, #14845, #24481, #17448, #19436, #12564, #24188, #21883, #3727, #26332, #28955, #26797, #5868, #28809, #10736, #24042, #29258, #994, #10277, #3579, #8290, #5415, #17599, #3141, #4025, #20634, #9025, #8440, #27264, #18349, #22948, #6463, #11180, #2048, #13320, #4474, #27705, #6164, #13764, #1742, #25380, #20186, #8731, #15756, #17884, #13617, #22644, #1599, #10876, #11327, #16053 ),
 .UNSPECIFIED., .F., .F.,
 ( 4, 2, 2, 2, 2, 2, 2, 2, 2, 2, 2, 2, 2, 2, 2, 2, 2, 2, 2, 2, 2, 2, 2, 2, 2, 2, 2, 2, 2, 2, 2, 2, 2, 2, 2, 2, 2, 2, 2, 2, 2, 2, 2, 2, 2, 2, 2, 2, 2, 2, 2, 2, 2, 2, 2, 2, 2, 2, 2, 2, 2, 2, 2, 2, 2, 2, 2, 2, 2, 2, 2, 2, 2, 2, 2, 2, 2, 2, 2, 2, 2, 2, 2, 2, 2, 2, 2, 2, 2, 2, 2, 2, 2, 2, 2, 2, 2, 2, 2, 2, 2, 2, 2, 2, 2, 2, 2, 2, 2, 2, 2, 2, 2, 2, 2, 2, 2, 2, 2, 2, 2, 2, 4 ),
 ( 0.000000000000000000, 0.007812500000000000000, 0.01464843750000000000, 0.02148437500000000000, 0.02832031250000000000, 0.03515625000000000000, 0.04882812500000000000, 0.05566406250000000000, 0.06250000000000000000, 0.06933593750000000000, 0.07617187500000000000, 0.08984375000000000000, 0.09667968750000000000, 0.1035156250000000000, 0.1103515625000000000, 0.1171875000000000000, 0.1240234375000000000, 0.1308593750000000000, 0.1376953125000000000, 0.1445312500000000000, 0.1513671875000000000, 0.1582031250000000000, 0.1718750000000000000, 0.1787109375000000000, 0.1855468750000000000, 0.1992187500000000000, 0.2060546875000000000, 0.2128906250000000000, 0.2197265625000000000, 0.2265625000000000000, 0.2402343750000000000, 0.2470703125000000000, 0.2539062500000000000, 0.2607421875000000000, 0.2675781250000000000, 0.2812500000000000000, 0.2880859375000000000, 0.2949218750000000000, 0.3017578125000000000, 0.3085937500000000000, 0.3154296875000000000, 0.3222656250000000000, 0.3291015625000000000, 0.3359375000000000000, 0.3496093750000000000, 0.3564453125000000000, 0.3632812500000000000, 0.3701171875000000000, 0.3769531250000000000, 0.3906250000000000000, 0.3974609375000000000, 0.4042968750000000000, 0.4179687500000000000, 0.4316406250000000000, 0.4384765625000000000, 0.4453125000000000000, 0.4521484375000000000, 0.4589843750000000000, 0.4658203125000000000, 0.4726562500000000000, 0.4794921875000000000, 0.4863281250000000000, 0.4931640625000000000, 0.5000000000000000000, 0.5078125000000000000, 0.5156250000000000000, 0.5234375000000000000, 0.5312500000000000000, 0.5390625000000000000, 0.5468750000000000000, 0.5625000000000000000, 0.5693359375000000000, 0.5761718750000000000, 0.5898437500000000000, 0.5966796875000000000, 0.6035156250000000000, 0.6103515625000000000, 0.6171875000000000000, 0.6308593750000000000, 0.6376953125000000000, 0.6445312500000000000, 0.6513671875000000000, 0.6582031250000000000, 0.6718750000000000000, 0.6787109375000000000, 0.6855468750000000000, 0.6992187500000000000, 0.7128906250000000000, 0.7197265625000000000, 0.7265625000000000000, 0.7333984375000000000, 0.7402343750000000000, 0.7470703125000000000, 0.7539062500000000000, 0.7607421875000000000, 0.7675781250000000000, 0.7744140625000000000, 0.7812500000000000000, 0.7890625000000000000, 0.7968750000000000000, 0.8046875000000000000, 0.8125000000000000000, 0.8203125000000000000, 0.8281250000000000000, 0.8437500000000000000, 0.8505859375000000000, 0.8574218750000000000, 0.8710937500000000000, 0.8779296875000000000, 0.8847656250000000000, 0.8916015625000000000, 0.8984375000000000000, 0.9121093750000000000, 0.9189453125000000000, 0.9257812500000000000, 0.9326171875000000000, 0.9394531250000000000, 0.9531250000000000000, 0.9589843750000000000, 0.9648437500000000000, 0.9765625000000000000, 0.9882812500000000000, 1.000000000000000000 ),
 .UNSPECIFIED. ) ;
#16356=CARTESIAN_POINT ( 'NONE',  ( 10.72091424521701519, 16.63063227333373462, -15.95414859203816782 ) ) ;
#16362=CARTESIAN_POINT ( 'NONE',  ( 11.47276097331165623, 9.269810413962238371, -15.86095999428340697 ) ) ;
#16365=CARTESIAN_POINT ( 'NONE',  ( 15.96855819401819865, 6.783166013289068985, -19.29613786212107840 ) ) ;
#16368=CARTESIAN_POINT ( 'NONE',  ( 27.11191462667604313, -11.78482644060662743, -13.28705938033944989 ) ) ;
#16371=CARTESIAN_POINT ( 'NONE',  ( 11.27618196228310232, 16.67695941232857137, -16.78452903358395076 ) ) ;
#16374=CARTESIAN_POINT ( 'NONE',  ( 35.54859390953724585, -21.18451583373416014, -18.19919658220850422 ) ) ;
#16375=CARTESIAN_POINT ( 'NONE',  ( 16.77165338796101324, 10.12286561294300569, -15.51291369241808304 ) ) ;
#16377=CARTESIAN_POINT ( 'NONE',  ( 23.86193934616450818, -4.638293873783104537, -19.03466029786466152 ) ) ;
#16381=CARTESIAN_POINT ( 'NONE',  ( 22.90957683611224738, 2.308586283387667581, -16.61139769879808625 ) ) ;
#16382=CARTESIAN_POINT ( 'NONE',  ( 15.60254075764268755, 8.625145012302763092, -14.61600764054077395 ) ) ;
#16396=CARTESIAN_POINT ( 'NONE',  ( 9.913797604922770290, 16.41941541294738727, -16.50570979788118464 ) ) ;
#16397=CARTESIAN_POINT ( 'NONE',  ( 26.04927874075684713, 0.2391533594452614209, -17.67486400872287788 ) ) ;
#16398=CARTESIAN_POINT ( 'NONE',  ( 21.30888034401541731, -0.8953576338359930942, -14.03585182699830369 ) ) ;
#16399=CARTESIAN_POINT ( 'NONE',  ( 31.92618181579182135, -10.29178896789921893, -18.33933693937521880 ) ) ;
#16401=CARTESIAN_POINT ( 'NONE',  ( 12.51757296969303290, 8.578467993704791184, -15.11616904564172792 ) ) ;
#16409=CARTESIAN_POINT ( 'NONE',  ( 10.33931768503335924, 18.38068274058360885, -17.76381606660089929 ) ) ;
#16417=CARTESIAN_POINT ( 'NONE',  ( 17.95327243003904982, 7.812726124483462264, -14.88485059575767266 ) ) ;
#16418=CARTESIAN_POINT ( 'NONE',  ( 15.41555982967951444, 8.269517134526982005, -21.14450021912286104 ) ) ;
#16420=CARTESIAN_POINT ( 'NONE',  ( 35.21546461977369091, -21.68794239832507742, -20.90642333977985956 ) ) ;
#16422=CARTESIAN_POINT ( 'NONE',  ( 20.47999367081501632, -2.041782396245861442, -15.93780510180117638 ) ) ;
#16423=CARTESIAN_POINT ( 'NONE',  ( 21.74214448781610542, 1.960522507982400020, -19.23370281053773923 ) ) ;
#16425=CARTESIAN_POINT ( 'NONE',  ( 27.29378187812181267, -6.326311925282933402, -12.73600023524891967 ) ) ;
#16433=CARTESIAN_POINT ( 'NONE',  ( 34.64580997985590471, -12.63631557036062247, -18.97247631304233195 ) ) ;
#16434=CARTESIAN_POINT ( 'NONE',  ( 17.10490717348788081, 9.547663288818908356, -11.45998271326893381 ) ) ;
#16438=CARTESIAN_POINT ( 'NONE',  ( 10.47224519147693478, 16.45115926513079074, -17.33471155705291977 ) ) ;
#16451=CARTESIAN_POINT ( 'NONE',  ( 9.668885350391278166, 16.22271324469333109, -17.88465541571617834 ) ) ;
#16453=CARTESIAN_POINT ( 'NONE',  ( 23.59197141788265384, -6.183129490800155281, -14.78464116683282015 ) ) ;
#16454=CARTESIAN_POINT ( 'NONE',  ( 20.29352232415978463, 1.537418251635638944, -14.27211978419980021 ) ) ;
#16458=CARTESIAN_POINT ( 'NONE',  ( 23.21730923944814506, -4.364887171357101359, -13.63095412955673247 ) ) ;
#16464=CARTESIAN_POINT ( 'NONE',  ( 10.47452605456472696, 16.44069893626776491, -17.33376834041267145 ) ) ;
#16465=CARTESIAN_POINT ( 'NONE',  ( 35.54287943964028784, -22.15884374752674546, -18.65915260879160797 ) ) ;
#16466=CARTESIAN_POINT ( 'NONE',  ( 32.62126879184269512, -11.04717877266006987, -18.30218954475424908 ) ) ;
#16469=CARTESIAN_POINT ( 'NONE',  ( 8.944584683310379702, 16.95159276115599667, -17.93331994345748726 ) ) ;
#16472=CARTESIAN_POINT ( 'NONE',  ( 19.23836061553175369, 5.151828676608854352, -13.99136221198299168 ) ) ;
#16473=CARTESIAN_POINT ( 'NONE',  ( 11.05545861061968083, 17.68922483874021978, -17.89384690447096560 ) ) ;
#16478=CARTESIAN_POINT ( 'NONE',  ( 9.826288910175632552, 16.82074144182198694, -16.60662094963572244 ) ) ;
#16481=CARTESIAN_POINT ( 'NONE',  ( 10.07879545831710999, 15.66271422494645904, -16.43741374977755143 ) ) ;
#16488=CARTESIAN_POINT ( 'NONE',  ( 10.73134732381016576, 15.26288385841099249, -17.22756371135774245 ) ) ;
#16489=CARTESIAN_POINT ( 'NONE',  ( 33.89278150306358128, -11.43586942258664507, -20.72336631513872973 ) ) ;
#16490=CARTESIAN_POINT ( 'NONE',  ( 29.90031526554274777, -7.862644070287768905, -16.42500436498598049 ) ) ;
#16491=CARTESIAN_POINT ( 'NONE',  ( 29.30346499805017757, -7.722527705200430859, -14.56292402596598556 ) ) ;
#16497=CARTESIAN_POINT ( 'NONE',  ( 29.95311431238071975, -11.57681909846818691, -12.96816900313696230 ) ) ;
#16499=CARTESIAN_POINT ( 'NONE',  ( 28.32023557703361405, -7.180604414193060059, -17.61256657898508138 ) ) ;
#16509=CARTESIAN_POINT ( 'NONE',  ( 10.72487265201256434, 16.61247851518984575, -15.95251179903439542 ) ) ;
#16515=CARTESIAN_POINT ( 'NONE',  ( 11.47181023233108021, 9.274170903235749108, -15.86135313853478657 ) ) ;
#16519=CARTESIAN_POINT ( 'NONE',  ( 10.31625730718771017, 13.25378293009361563, -17.61694433892753153 ) ) ;
#16520=CARTESIAN_POINT ( 'NONE',  ( 20.64663396976543552, 5.620433075351431995, -17.27584747705915902 ) ) ;
#16525=CARTESIAN_POINT ( 'NONE',  ( 29.82081855766934453, -7.722587238354316597, -15.76009366473342332 ) ) ;
#16530=CARTESIAN_POINT ( 'NONE',  ( 11.27674754065650653, 16.67436559781366157, -16.78429523206404994 ) ) ;
#16532=CARTESIAN_POINT ( 'NONE',  ( 33.47764622482974062, -12.08535443106849883, -18.57070694247861553 ) ) ;
#16535=CARTESIAN_POINT ( 'NONE',  ( 27.46460276834485370, -5.912627539431687396, -19.42860466253708296 ) ) ;
#16539=CARTESIAN_POINT ( 'NONE',  ( 16.12927480167980576, 2.990883400875756326, -18.25071113400840517 ) ) ;
#16540=CARTESIAN_POINT ( 'NONE',  ( 17.51631511252498186, 5.448942031446791567, -19.07752241466814880 ) ) ;
#16553=CARTESIAN_POINT ( 'NONE',  ( 9.915973561396301150, 16.40943619918981256, -16.50475030878699556 ) ) ;
#16554=CARTESIAN_POINT ( 'NONE',  ( 24.12676367385581244, 0.3224161365626431741, -13.25522683364457777 ) ) ;
#16555=CARTESIAN_POINT ( 'NONE',  ( 24.14852421541024441, 0.2028892341458684023, -15.23052705399570428 ) ) ;
#16556=CARTESIAN_POINT ( 'NONE',  ( 33.21739345078569272, -12.71166704379270129, -20.69560413545502797 ) ) ;
#16561=CARTESIAN_POINT ( 'NONE',  ( 16.53304876882650731, 8.555045913257369961, -19.77053526944897754 ) ) ;
#16566=CARTESIAN_POINT ( 'NONE',  ( 10.72487265201256434, 16.61247851518984575, -15.95251179903439542 ) ) ;
#16572=CARTESIAN_POINT ( 'NONE',  ( 15.44629794785920218, 3.545610805586186132, -16.71614555938632307 ) ) ;
#16573=CARTESIAN_POINT ( 'NONE',  ( 16.69609108537820674, 9.478167028156011753, -20.90851310094495474 ) ) ;
#16575=CARTESIAN_POINT ( 'NONE',  ( 32.68951927270060764, -11.07419627511998605, -18.48540492261787449 ) ) ;
#16576=CARTESIAN_POINT ( 'NONE',  ( 24.04487210496366245, -0.6674514567044148583, -16.01806975046538284 ) ) ;
#16577=CARTESIAN_POINT ( 'NONE',  ( 20.63695664501197413, 4.642632487595073520, -17.05591670970450124 ) ) ;
#16579=CARTESIAN_POINT ( 'NONE',  ( 29.92318863513849436, -9.020257460645494163, -14.67793329163371574 ) ) ;
#16589=CARTESIAN_POINT ( 'NONE',  ( 35.71575670127456448, -17.44301942315582110, -19.29589553906783905 ) ) ;
#16590=CARTESIAN_POINT ( 'NONE',  ( 12.75568354342045119, 7.625663700289499580, -14.92639070443840588 ) ) ;
#16594=CARTESIAN_POINT ( 'NONE',  ( 12.03623766312057519, 9.280706639558555793, -16.68777662621714342 ) ) ;
#16606=CARTESIAN_POINT ( 'NONE',  ( 9.662623034719734605, 16.25143302262299372, -17.90105808085208849 ) ) ;
#16608=CARTESIAN_POINT ( 'NONE',  ( 27.58270427615865472, -5.135490454175970498, -17.42064064436273085 ) ) ;
#16609=CARTESIAN_POINT ( 'NONE',  ( 23.39789874936200320, -0.01207823811560896493, -14.43595595811700782 ) ) ;
#16613=CARTESIAN_POINT ( 'NONE',  ( 28.16462234717350199, -5.661059359726887230, -16.30864077692347536 ) ) ;
#16622=CARTESIAN_POINT ( 'NONE',  ( 10.47195275365909595, 16.45250042224058618, -17.33483252618548676 ) ) ;
#16624=CARTESIAN_POINT ( 'NONE',  ( 33.75544676243647757, -14.12885555826641593, -19.81592319558764004 ) ) ;
#16626=CARTESIAN_POINT ( 'NONE',  ( 8.944584683310379702, 16.95159276115599667, -17.91928203681695564 ) ) ;
#16629=CARTESIAN_POINT ( 'NONE',  ( 18.50902107916489570, 2.085137940960992697, -20.06823964296112450 ) ) ;
#16630=CARTESIAN_POINT ( 'NONE',  ( 11.28016675873817576, 16.65868462784220227, -16.78288126510920719 ) ) ;
#16636=CARTESIAN_POINT ( 'NONE',  ( 9.843778300897430000, 16.74053286659246709, -16.57516421589427225 ) ) ;
#16638=CARTESIAN_POINT ( 'NONE',  ( 9.912057827679275235, 16.42739425315605928, -16.50652470164456531 ) ) ;
#16643=CARTESIAN_POINT ( 'NONE',  ( 10.47705880869930084, 16.42908340295556258, -17.33272095748315422 ) ) ;
#16646=CARTESIAN_POINT ( 'NONE',  ( 36.54859390953724585, -22.18451583373416014, -16.11276402859391865 ) ) ;
#16648=CARTESIAN_POINT ( 'NONE',  ( 27.01132674553606350, -11.00696853675122711, -18.49859303458091730 ) ) ;
#16649=CARTESIAN_POINT ( 'NONE',  ( 15.95367323521391256, 9.281262803959288377, -20.14168370736028280 ) ) ;
#16653=CARTESIAN_POINT ( 'NONE',  ( 32.33411138940433460, -10.22844123512284575, -15.25869122620317953 ) ) ;
#16654=CARTESIAN_POINT ( 'NONE',  ( 15.11341857612343809, 8.679638894638937785, -13.66094189273949056 ) ) ;
#16655=CARTESIAN_POINT ( 'NONE',  ( 16.77165338796101324, 10.12286561294300569, -15.51291369241808304 ) ) ;
#16666=CARTESIAN_POINT ( 'NONE',  ( 10.33819201225523621, 18.38584521943398187, -17.87775236254758227 ) ) ;
#16671=CARTESIAN_POINT ( 'NONE',  ( 9.997747326010761881, 16.03441129093729245, -16.47093000352221637 ) ) ;
#16673=CARTESIAN_POINT ( 'NONE',  ( 9.667859086210386366, 16.22741982304516739, -17.88507982571460531 ) ) ;
#16674=CARTESIAN_POINT ( 'NONE',  ( 20.19814137509539975, 5.716210941879356078, -15.87681946797394517 ) ) ;
#16677=CARTESIAN_POINT ( 'NONE',  ( 29.88803641097454999, -7.968445601786871002, -16.75847372370488131 ) ) ;
#16680=CARTESIAN_POINT ( 'NONE',  ( 11.25757798850943381, 16.76227960750979307, -16.79548539596511247 ) ) ;
#16682=CARTESIAN_POINT ( 'NONE',  ( 33.51257387524950815, -12.16639167148776224, -18.62538556556795655 ) ) ;
#16683=CARTESIAN_POINT ( 'NONE',  ( 14.03850921439652311, 8.975161913830900673, -15.18271992443145635 ) ) ;
#16686=CARTESIAN_POINT ( 'NONE',  ( 9.371932165391852365, 14.99172273419688750, -16.94745289082924344 ) ) ;
#16687=CARTESIAN_POINT ( 'NONE',  ( 31.26470888135608206, -7.466309307788507432, -16.51192723299172727 ) ) ;
#16692=CARTESIAN_POINT ( 'NONE',  ( 16.54288150113237066, 3.399532473721276649, -19.15960874834559746 ) ) ;
#16693=CARTESIAN_POINT ( 'NONE',  ( 17.31141255128542511, 8.026854538702009378, -19.31233526832781777 ) ) ;
#16709=CARTESIAN_POINT ( 'NONE',  ( 9.641354186875979337, 17.66887565656821124, -17.90893343548146177 ) ) ;
#16710=CARTESIAN_POINT ( 'NONE',  ( 27.81650010061016332, -6.490163795910067535, -14.16582606047713178 ) ) ;
#16711=CARTESIAN_POINT ( 'NONE',  ( 20.86695504291294156, -3.984745147917406971, -17.88565525751875995 ) ) ;
#16712=CARTESIAN_POINT ( 'NONE',  ( 33.13932541451587355, -12.36573032794433047, -20.66922553108291538 ) ) ;
#16718=CARTESIAN_POINT ( 'NONE',  ( 14.57776618122778700, 6.338444840345393239, -15.85465340776532095 ) ) ;
#16721=CARTESIAN_POINT ( 'NONE',  ( 10.72074420406304895, 16.63141210374104872, -15.95421917676928025 ) ) ;
#16724=CARTESIAN_POINT ( 'NONE',  ( 15.39489021548154568, 6.697694061803245447, -14.95590323207311734 ) ) ;
#16725=CARTESIAN_POINT ( 'NONE',  ( 13.09464261414706066, 5.717622835290344874, -15.96348941799783816 ) ) ;
#16727=CARTESIAN_POINT ( 'NONE',  ( 33.41663030065195272, -12.60673267154789201, -19.71350710734569134 ) ) ;
#16729=CARTESIAN_POINT ( 'NONE',  ( 21.43024726678804726, -3.720057188146618010, -16.74626013867020902 ) ) ;
#16730=CARTESIAN_POINT ( 'NONE',  ( 20.49785840140504689, 4.750029832917431527, -16.36601636927073145 ) ) ;
#16732=CARTESIAN_POINT ( 'NONE',  ( 28.61400761516875590, -9.413816014945153299, -13.42719155385534080 ) ) ;
#16743=CARTESIAN_POINT ( 'NONE',  ( 36.54859497913844990, -21.18452063888661385, -18.28382709584098720 ) ) ;
#16745=CARTESIAN_POINT ( 'NONE',  ( 14.64119204185053391, 8.458903494591371697, -13.42360716063767967 ) ) ;
#16749=CARTESIAN_POINT ( 'NONE',  ( 12.01190781424926435, 9.390070215761314287, -16.69800690218674788 ) ) ;
#16758=CARTESIAN_POINT ( 'NONE',  ( 13.37268442792299261, 7.622911828202562745, -15.71339253741762221 ) ) ;
#16760=CARTESIAN_POINT ( 'NONE',  ( 27.43603605124483025, -4.716368786860208218, -15.63773258035017300 ) ) ;
#16762=CARTESIAN_POINT ( 'NONE',  ( 22.42023978564754927, -3.655767601918122445, -13.54521809681785172 ) ) ;
#16773=CARTESIAN_POINT ( 'NONE',  ( 11.99569818778800645, 9.464409628959467469, -16.70471015293584216 ) ) ;
#16775=CARTESIAN_POINT ( 'NONE',  ( 35.07504771885155037, -20.05712364337910714, -20.21480690768607857 ) ) ;
#16777=CARTESIAN_POINT ( 'NONE',  ( 8.944584683310379702, 16.95159276115599667, -17.91796598306941135 ) ) ;
#16779=CARTESIAN_POINT ( 'NONE',  ( 17.96884874826282186, 1.586046385177752871, -19.67104016136476119 ) ) ;
#16780=CARTESIAN_POINT ( 'NONE',  ( 12.83225144795546235, 9.540626470039393681, -16.14103964284477399 ) ) ;
#16783=CARTESIAN_POINT ( 'NONE',  ( 10.24089172292967298, 14.91932009296530559, -16.37038124228770997 ) ) ;
#16786=CARTESIAN_POINT ( 'NONE',  ( 9.913797604922770290, 16.41941541294738727, -16.50570979788118464 ) ) ;
#16791=CARTESIAN_POINT ( 'NONE',  ( 10.47224519147693478, 16.45115926513079074, -17.33471155705291977 ) ) ;
#16794=CARTESIAN_POINT ( 'NONE',  ( 32.85377328814971065, -9.687349299063408026, -18.71178847241494481 ) ) ;
#16795=CARTESIAN_POINT ( 'NONE',  ( 28.06689949639850212, -8.111051215268487269, -13.49421662364394514 ) ) ;
#16796=CARTESIAN_POINT ( 'NONE',  ( 26.87449084144840938, -11.88902188497427481, -13.49525739704605343 ) ) ;
#16799=CARTESIAN_POINT ( 'NONE',  ( 32.46393572324419807, -10.24815885013986794, -15.62561752695271622 ) ) ;
#16800=CARTESIAN_POINT ( 'NONE',  ( 18.95088517700565944, -0.6660330538943091128, -18.51770762617101340 ) ) ;
#16801=CARTESIAN_POINT ( 'NONE',  ( 26.64397501440380012, -9.555891369342745634, -14.23407566704858951 ) ) ;
#16809=CARTESIAN_POINT ( 'NONE',  ( 12.27697253541231426, 9.494350595542041304, -15.31066389949581463 ) ) ;
#16814=CARTESIAN_POINT ( 'NONE',  ( 12.50736435846123484, 8.573956625762026107, -15.12430548898761806 ) ) ;
#16816=CARTESIAN_POINT ( 'NONE',  ( 17.05751464226099401, 1.788256342680895949, -18.14502383782993888 ) ) ;
#16823=CARTESIAN_POINT ( 'NONE',  ( 11.05541542350396256, 17.68942290035798237, -17.91468072056456862 ) ) ;
#16827=CARTESIAN_POINT ( 'NONE',  ( 35.54582861202835886, -21.17209281684672817, -18.49356017204852520 ) ) ;
#16828=CARTESIAN_POINT ( 'NONE',  ( 17.18819971663578272, 0.8441372818425427749, -18.45219435416397502 ) ) ;
#16832=CARTESIAN_POINT ( 'NONE',  ( 10.02031722384195156, 12.01814620627372143, -16.67932286086919902 ) ) ;
#16834=CARTESIAN_POINT ( 'NONE',  ( 31.24625831705917278, -7.622123577322120980, -17.00257116200763008 ) ) ;
#16837=CARTESIAN_POINT ( 'NONE',  ( 19.47744964272635926, 1.166342761889149982, -14.46873920536258495 ) ) ;
#16838=CARTESIAN_POINT ( 'NONE',  ( 17.65840769916877662, 9.384080434346836697, -15.74689851229248738 ) ) ;
#16852=CARTESIAN_POINT ( 'NONE',  ( 9.695397291186985456, 17.42102709130404747, -17.08803885907851594 ) ) ;
#16853=CARTESIAN_POINT ( 'NONE',  ( 28.61166709039449785, -6.781025521995295513, -16.93684798036101213 ) ) ;
#16854=CARTESIAN_POINT ( 'NONE',  ( 21.92441584138004984, 2.204866226087792924, -14.79409581392398110 ) ) ;
#16855=CARTESIAN_POINT ( 'NONE',  ( 35.21546461977369091, -21.68794239832507742, -20.90642333977985956 ) ) ;
#16861=CARTESIAN_POINT ( 'NONE',  ( 19.52227536296714305, 7.868296793410291201, -18.00468392081665669 ) ) ;
#16863=CARTESIAN_POINT ( 'NONE',  ( 10.33813570737955700, 18.38610344077106973, -17.89676158639688452 ) ) ;
#16868=CARTESIAN_POINT ( 'NONE',  ( 15.93484470893836935, 6.939319753835953009, -14.67888072223970752 ) ) ;
#16871=CARTESIAN_POINT ( 'NONE',  ( 26.36605488913174611, -12.34709378291890758, -12.75955235896099005 ) ) ;
#16873=CARTESIAN_POINT ( 'NONE',  ( 35.24964364652129234, -20.84149066036063047, -20.16262864730545346 ) ) ;
#16874=CARTESIAN_POINT ( 'NONE',  ( 23.66523006742493251, -0.7244823556979478330, -15.35173719993635011 ) ) ;
#16876=CARTESIAN_POINT ( 'NONE',  ( 19.79871159306781436, 4.571585941193342606, -15.48227718036497080 ) ) ;
#16878=CARTESIAN_POINT ( 'NONE',  ( 29.51995068812739476, -6.211492405346085377, -16.93985997890334261 ) ) ;
#16885=CARTESIAN_POINT ( 'NONE',  ( 33.30032953382602301, -10.37518355935928938, -17.98954529685971337 ) ) ;
#16887=CARTESIAN_POINT ( 'NONE',  ( 12.76959483864652611, 7.631811206235384226, -14.91530316759754982 ) ) ;
#16891=CARTESIAN_POINT ( 'NONE',  ( 13.11714404544056656, 8.568033937426095648, -15.91706119101506545 ) ) ;
#16903=CARTESIAN_POINT ( 'NONE',  ( 11.25771276049011327, 8.953580691464267716, -17.22628983894280807 ) ) ;
#16904=CARTESIAN_POINT ( 'NONE',  ( 27.60672911170952304, -4.775276709060196190, -16.23362067418393195 ) ) ;
#16905=CARTESIAN_POINT ( 'NONE',  ( 24.30592326428028827, -5.273034306582022879, -19.67074064463221106 ) ) ;
#16917=CARTESIAN_POINT ( 'NONE',  ( 10.49225533350670858, 16.35939020308235925, -17.32643665990597981 ) ) ;
#16920=CARTESIAN_POINT ( 'NONE',  ( 32.77977724007769211, -11.13765286058784554, -18.71157503069099448 ) ) ;
#16922=CARTESIAN_POINT ( 'NONE',  ( 13.37720302390605553, 7.624891072754538257, -15.70979247928349132 ) ) ;
#16925=CARTESIAN_POINT ( 'NONE',  ( 21.40051611374530793, -0.1690565882708310874, -20.18282279970310000 ) ) ;
#16926=CARTESIAN_POINT ( 'NONE',  ( 12.86729516143382845, 9.515644835462770956, -16.11619563230584973 ) ) ;
#16931=CARTESIAN_POINT ( 'NONE',  ( 10.07879545831710999, 15.66271422494645904, -16.43741374977755143 ) ) ;
#16933=CARTESIAN_POINT ( 'NONE',  ( 9.649959050778257108, 17.62941265384766254, -17.56860460898032628 ) ) ;
#16940=CARTESIAN_POINT ( 'NONE',  ( 12.07790154976966868, 9.144051220271959934, -16.66639656463015839 ) ) ;
#16943=CARTESIAN_POINT ( 'NONE',  ( 34.08234396701924851, -12.11069646272769162, -20.88346212624082909 ) ) ;
#16944=CARTESIAN_POINT ( 'NONE',  ( 16.19004574127830054, 9.516462436566445859, -20.03842800660303070 ) ) ;
#16945=CARTESIAN_POINT ( 'NONE',  ( 15.30534275580653869, 10.60631812597827839, -15.20037037882373987 ) ) ;
#16949=CARTESIAN_POINT ( 'NONE',  ( 34.18187006836440389, -11.68445768601494628, -19.79758194388510972 ) ) ;
#16951=CARTESIAN_POINT ( 'NONE',  ( 18.98834166481877972, 4.258514017552020192, -15.11364409576566459 ) ) ;
#16952=CARTESIAN_POINT ( 'NONE',  ( 17.21692058948253035, 4.245457944912791604, -14.13226496128363863 ) ) ;
#16965=CARTESIAN_POINT ( 'NONE',  ( 12.14726737398757095, 10.08919500705755645, -15.36430154580878593 ) ) ;
#16970=CARTESIAN_POINT ( 'NONE',  ( 12.43696608443014284, 8.546664718661613591, -15.18012293544581226 ) ) ;
#16973=CARTESIAN_POINT ( 'NONE',  ( 20.29966856415212817, 4.923229158599749411, -18.85509502865480869 ) ) ;
#16979=CARTESIAN_POINT ( 'NONE',  ( 12.82818608578791064, 9.559270667424515366, -16.14272081857926366 ) ) ;
#16982=CARTESIAN_POINT ( 'NONE',  ( 33.26400919001463308, -11.80307911188568148, -18.11217348381727632 ) ) ;
#16983=CARTESIAN_POINT ( 'NONE',  ( 21.64656857049893901, 5.639188926465734220, -17.17864421186117951 ) ) ;
#16985=CARTESIAN_POINT ( 'NONE',  ( 16.38240814442996651, 6.370603895193741373, -13.89573738210111919 ) ) ;
#16990=CARTESIAN_POINT ( 'NONE',  ( 20.86695504291294156, -3.984745147917406971, -17.88565525751875995 ) ) ;
#16991=CARTESIAN_POINT ( 'NONE',  ( 17.86202776125589153, 5.750484210099715554, -19.07881598002096268 ) ) ;
#17006=CARTESIAN_POINT ( 'NONE',  ( 11.48249212886396897, 9.228508165798535501, -15.85668214399537845 ) ) ;
#17008=CARTESIAN_POINT ( 'NONE',  ( 28.49100808714443289, -10.93160309251996765, -13.65156567797833631 ) ) ;
#17009=CARTESIAN_POINT ( 'NONE',  ( 27.20456514074317056, -5.347416052021189081, -13.22196079581408235 ) ) ;
#17010=CARTESIAN_POINT ( 'NONE',  ( 32.54305136433941215, -11.03529315477374517, -18.08112484791816499 ) ) ;
#17018=CARTESIAN_POINT ( 'NONE',  ( 19.38992137333195842, 2.881095379261479739, -20.30776781288435373 ) ) ;
#17021=CARTESIAN_POINT ( 'NONE',  ( 10.72145343393089512, 16.62815948516130504, -15.95392576598924350 ) ) ;
#17024=CARTESIAN_POINT ( 'NONE',  ( 19.83745040964868522, -2.306422872736943575, -14.39351019504378293 ) ) ;
#17025=CARTESIAN_POINT ( 'NONE',  ( 30.21326039400183561, -7.476461571224066738, -17.86537319528562051 ) ) ;
#17027=CARTESIAN_POINT ( 'NONE',  ( 32.67186286342521839, -11.06527230177895227, -18.43913201350460440 ) ) ;
#17029=CARTESIAN_POINT ( 'NONE',  ( 25.72346593501046996, -2.209713236584236018, -16.07608620281017053 ) ) ;
#17030=CARTESIAN_POINT ( 'NONE',  ( 19.42159491456138554, 2.195880709831018684, -14.63272625841335106 ) ) ;
#17043=CARTESIAN_POINT ( 'NONE',  ( 33.28625081342995884, -10.37305140221732991, -17.94975064729133862 ) ) ;
#17045=CARTESIAN_POINT ( 'NONE',  ( 10.07879545831710999, 15.66271422494645904, -16.43741374977755143 ) ) ;
#17049=CARTESIAN_POINT ( 'NONE',  ( 12.06596557120094992, 9.177570865404522493, -16.67295095431955332 ) ) ;
#17059=CARTESIAN_POINT ( 'NONE',  ( 12.60230244812736800, 7.534144488243946114, -16.30820540178382316 ) ) ;
#17061=CARTESIAN_POINT ( 'NONE',  ( 24.24519292511275737, -8.489478586693508078, -18.02380513063773648 ) ) ;
#17062=CARTESIAN_POINT ( 'NONE',  ( 26.86433939054618492, -2.362129714094441724, -16.96571632802953644 ) ) ;
#17077=CARTESIAN_POINT ( 'NONE',  ( 10.47300640208398370, 16.44766825625507778, -17.33439677017039671 ) ) ;
#17078=CARTESIAN_POINT ( 'NONE',  ( 35.54287943964028784, -22.15884374752674546, -18.65915260879160797 ) ) ;
#17081=CARTESIAN_POINT ( 'NONE',  ( 8.944584683310379702, 16.95159276115599667, -17.92015940598198753 ) ) ;
#17083=CARTESIAN_POINT ( 'NONE',  ( 24.00918528248616468, -0.5066965781341161712, -13.81223085940890627 ) ) ;
#17084=CARTESIAN_POINT ( 'NONE',  ( 12.83226850357503501, 9.540548187773516986, -16.14103259455261608 ) ) ;
#17087=CARTESIAN_POINT ( 'NONE',  ( 11.47310491742633687, 9.268236560789974376, -15.86081749295074594 ) ) ;
#17089=CARTESIAN_POINT ( 'NONE',  ( 12.23783994716398560, 8.515526397163364791, -15.33449341356891615 ) ) ;
#17094=CARTESIAN_POINT ( 'NONE',  ( 12.40302661446015264, 8.678734247659738443, -16.45371344743900366 ) ) ;
#17096=CARTESIAN_POINT ( 'NONE',  ( 35.74526169011073762, -19.57556970876266433, -21.38945728569726867 ) ) ;
#17097=CARTESIAN_POINT ( 'NONE',  ( 27.26129135193747999, -10.77754955263135095, -18.64424489656416739 ) ) ;
#17098=CARTESIAN_POINT ( 'NONE',  ( 13.52175692814481067, 9.804829593628518580, -15.59458061523717909 ) ) ;
#17104=CARTESIAN_POINT ( 'NONE',  ( 19.79871159306781436, 4.571585941193342606, -15.48227718036497080 ) ) ;
#17106=CARTESIAN_POINT ( 'NONE',  ( 16.57956996521092918, 4.788269978297743812, -19.71382457362092566 ) ) ;
#17116=CARTESIAN_POINT ( 'NONE',  ( 12.26306961015461461, 9.515005556349402482, -15.31970085818224980 ) ) ;
#17122=CARTESIAN_POINT ( 'NONE',  ( 11.47464782381437587, 9.261287281732329291, -15.86016978468419936 ) ) ;
#17124=CARTESIAN_POINT ( 'NONE',  ( 18.39947282702827991, 3.040288584705510999, -19.58888106367123427 ) ) ;
#17131=CARTESIAN_POINT ( 'NONE',  ( 11.92449941057312124, 13.70369295321711256, -16.51642704783386506 ) ) ;
#17133=CARTESIAN_POINT ( 'NONE',  ( 36.49521523454778560, -20.94471372247522467, -19.05937150832556526 ) ) ;
#17134=CARTESIAN_POINT ( 'NONE',  ( 15.93484470893836935, 6.939319753835953009, -14.67888072223970752 ) ) ;
#17138=CARTESIAN_POINT ( 'NONE',  ( 15.84550288711180777, 10.06862660282224731, -14.00251831694083826 ) ) ;
#17142=CARTESIAN_POINT ( 'NONE',  ( 19.87821071931953298, -1.530402839103173651, -15.12151443550766494 ) ) ;
#17143=CARTESIAN_POINT ( 'NONE',  ( 19.77208840006000656, -0.3814412559078061982, -20.24210485642555568 ) ) ;
#17154=CARTESIAN_POINT ( 'NONE',  ( 11.47327446659168615, 9.267463859335506982, -15.86074700677745852 ) ) ;
#17155=CARTESIAN_POINT ( 'NONE',  ( 29.74223563811278481, -10.39579538818624549, -13.90533736129563813 ) ) ;
#17156=CARTESIAN_POINT ( 'NONE',  ( 24.59824444495380646, -5.013944910511990649, -19.70109713935865514 ) ) ;
#17157=CARTESIAN_POINT ( 'NONE',  ( 32.48283477683061449, -11.02614750807341260, -17.91093295056291979 ) ) ;
#17164=CARTESIAN_POINT ( 'NONE',  ( 17.55424633453837302, 0.6138019359854992585, -14.89346452969079060 ) ) ;
#17168=CARTESIAN_POINT ( 'NONE',  ( 12.21210587983259366, 9.791837354264822935, -15.33748854281299323 ) ) ;
#17172=CARTESIAN_POINT ( 'NONE',  ( 20.24985932600369409, 3.694099309552050237, -20.13309853732883781 ) ) ;
#17173=CARTESIAN_POINT ( 'NONE',  ( 15.23446545079332815, 2.143032791470029341, -16.75203451335420368 ) ) ;
#17175=CARTESIAN_POINT ( 'NONE',  ( 34.11209566957792561, -15.73109017586260272, -19.92372960426217787 ) ) ;
#17178=CARTESIAN_POINT ( 'NONE',  ( 22.80194228990702143, -6.214338098008789224, -14.16187805771452801 ) ) ;
#17181=CARTESIAN_POINT ( 'NONE',  ( 26.10879525372914145, -2.341005984040549937, -13.07697618282131913 ) ) ;
#17183=CARTESIAN_POINT ( 'NONE',  ( 24.14317479683219858, -6.286850201977149055, -18.60698471650063723 ) ) ;
#17191=CARTESIAN_POINT ( 'NONE',  ( 13.51621490077814691, 9.019785729699995258, -14.32023381125561556 ) ) ;
#17192=CARTESIAN_POINT ( 'NONE',  ( 33.24108837279852224, -10.36619216719171632, -17.82210672427467912 ) ) ;
#17193=CARTESIAN_POINT ( 'NONE',  ( 9.917712295358372288, 16.40146214360271770, -16.50402730409559027 ) ) ;
#17197=CARTESIAN_POINT ( 'NONE',  ( 12.02685106364323531, 9.321538569219327997, -16.69182734290254899 ) ) ;
#17208=CARTESIAN_POINT ( 'NONE',  ( 11.26737699260669778, 8.919714795263022467, -17.22149591130980184 ) ) ;
#17210=CARTESIAN_POINT ( 'NONE',  ( 12.86846089198198584, 5.826474397738612865, -17.89591831848172276 ) ) ;
#17212=CARTESIAN_POINT ( 'NONE',  ( 24.38930386813997586, -0.5518329404549096040, -18.38842912410832753 ) ) ;
#17225=CARTESIAN_POINT ( 'NONE',  ( 13.12595734265553205, 8.571888915454989544, -15.91003987120930319 ) ) ;
#17226=CARTESIAN_POINT ( 'NONE',  ( 33.59450136257035524, -12.41883169790769692, -18.71738141962731561 ) ) ;
#17228=CARTESIAN_POINT ( 'NONE',  ( 9.090073284221231731, 16.28436349189565391, -17.07021669716791124 ) ) ;
#17229=CARTESIAN_POINT ( 'NONE',  ( 26.72181814967143509, -3.137724904577397389, -15.69709663067708050 ) ) ;
#17230=CARTESIAN_POINT ( 'NONE',  ( 12.50804596317817463, 11.02747407808666580, -16.27511002087113567 ) ) ;
#17235=CARTESIAN_POINT ( 'NONE',  ( 11.46877092736959014, 9.288109543210406827, -15.86260999805022820 ) ) ;
#17240=CARTESIAN_POINT ( 'NONE',  ( 12.03309083968702886, 9.293808706017943067, -16.68917936036902105 ) ) ;
#17242=CARTESIAN_POINT ( 'NONE',  ( 17.83966564144121136, 6.109271821037239647, -21.09843361817607388 ) ) ;
#17243=CARTESIAN_POINT ( 'NONE',  ( 13.44640266258695327, 6.638963897028184569, -16.15403403936744198 ) ) ;
#17250=CARTESIAN_POINT ( 'NONE',  ( 36.54859195715578579, -22.18450706271777406, -18.40832622446962930 ) ) ;
#17252=CARTESIAN_POINT ( 'NONE',  ( 17.63088349262504551, 4.212901655933308120, -18.95607689789294170 ) ) ;
#17253=CARTESIAN_POINT ( 'NONE',  ( 17.32873655921053313, 10.26331207550778579, -16.20725374984683143 ) ) ;
#17261=CARTESIAN_POINT ( 'NONE',  ( 12.27679999902766284, 9.495116139066881900, -15.31073721177884650 ) ) ;
#17266=CARTESIAN_POINT ( 'NONE',  ( 12.13006862794127017, 8.527244997094612700, -15.41586291625151972 ) ) ;
#17268=CARTESIAN_POINT ( 'NONE',  ( 10.68417091768239047, 8.977850322645869241, -16.40447401652228621 ) ) ;
#17275=CARTESIAN_POINT ( 'NONE',  ( 12.83210864641033844, 9.541281304504437344, -16.14109870176968897 ) ) ;
#17276=CARTESIAN_POINT ( 'NONE',  ( 34.56382110058589774, -12.26799042007339757, -18.94768870749412315 ) ) ;
#17277=CARTESIAN_POINT ( 'NONE',  ( 19.25048709941964376, 7.441878894999256921, -18.84525011105569803 ) ) ;
#17281=CARTESIAN_POINT ( 'NONE',  ( 19.85388831290292799, 7.668379621071204078, -15.62993620635094061 ) ) ;
#17287=CARTESIAN_POINT ( 'NONE',  ( 26.68443370873975340, -2.140902173977853540, -15.79004130932784555 ) ) ;
#17288=CARTESIAN_POINT ( 'NONE',  ( 17.82019932507133930, 1.781282266713458240, -14.47200660618688417 ) ) ;
#17297=CARTESIAN_POINT ( 'NONE',  ( 11.43229926783177497, 9.455373222906182207, -15.87769231223556332 ) ) ;
#17298=CARTESIAN_POINT ( 'NONE',  ( 27.33932411720343936, -8.205422078888220838, -18.29166945089792407 ) ) ;
#17299=CARTESIAN_POINT ( 'NONE',  ( 22.33774198005919587, -7.088069534354142220, -17.87445411435389886 ) ) ;
#17308=CARTESIAN_POINT ( 'NONE',  ( 15.44629794785920218, 3.545610805586186132, -16.71614555938632307 ) ) ;
#17311=CARTESIAN_POINT ( 'NONE',  ( 12.27694278248960558, 9.494486990809335225, -15.31067620760345527 ) ) ;
#17312=CARTESIAN_POINT ( 'NONE',  ( 32.12153525177792091, -10.97127362787143312, -16.88978156643115724 ) ) ;
#17314=CARTESIAN_POINT ( 'NONE',  ( 25.57370974413349884, -0.4222200280313516685, -16.88676729435558599 ) ) ;
#17316=CARTESIAN_POINT ( 'NONE',  ( 21.20591713499851849, 2.664298913801621538, -19.97344039048299891 ) ) ;
#17319=CARTESIAN_POINT ( 'NONE',  ( 35.54859390953724585, -22.18451583373416014, -16.94733705004010460 ) ) ;
#17321=CARTESIAN_POINT ( 'NONE',  ( 25.21061150575720333, -3.342243121390650717, -18.67481654970342930 ) ) ;
#17322=CARTESIAN_POINT ( 'NONE',  ( 25.18022790295009727, 0.7303485828293051485, -17.76052596840512621 ) ) ;
#17323=CARTESIAN_POINT ( 'NONE',  ( 26.38113052396219516, -11.59678093645141672, -17.84452879788985769 ) ) ;
#17331=CARTESIAN_POINT ( 'NONE',  ( 15.84550288711180777, 10.06862660282224731, -14.00251831694083826 ) ) ;
#17333=CARTESIAN_POINT ( 'NONE',  ( 34.63381380623899020, -13.58242311684542081, -20.01117170570581649 ) ) ;
#17334=CARTESIAN_POINT ( 'NONE',  ( 11.39177520167864266, 9.641221755901229429, -15.89445043910815336 ) ) ;
#17338=CARTESIAN_POINT ( 'NONE',  ( 13.14084490070201738, 8.578467993704791184, -15.89817422466314945 ) ) ;
#17349=CARTESIAN_POINT ( 'NONE',  ( 11.22197018571015725, 9.100068217651248403, -17.24240020332717904 ) ) ;
#17352=CARTESIAN_POINT ( 'NONE',  ( 13.03988341252192917, 6.056598437983586436, -18.79510648546616736 ) ) ;
#17353=CARTESIAN_POINT ( 'NONE',  ( 26.46413748225140594, -13.10274310649288942, -15.24000415025259692 ) ) ;
#17364=CARTESIAN_POINT ( 'NONE',  ( 13.12278719711289732, 8.570488965836000617, -15.91256645732111430 ) ) ;
#17367=CARTESIAN_POINT ( 'NONE',  ( 35.16668739017224965, -20.46881214373840763, -20.22602438870426766 ) ) ;
#17369=CARTESIAN_POINT ( 'NONE',  ( 9.113211330545484046, 16.17824946203780456, -17.05444305708079966 ) ) ;
#17373=CARTESIAN_POINT ( 'NONE',  ( 23.29338531092689735, -7.078548041224526521, -17.51562821661096336 ) ) ;
#17374=CARTESIAN_POINT ( 'NONE',  ( 12.83388176712078810, 9.535019011556107316, -16.14022287234750408 ) ) ;
#17379=CARTESIAN_POINT ( 'NONE',  ( 12.47535353872619446, 8.560407331872438519, -15.14977315560688176 ) ) ;
#17384=CARTESIAN_POINT ( 'NONE',  ( 12.11773132146483789, 9.045882004348337446, -16.64348121447567053 ) ) ;
#17387=CARTESIAN_POINT ( 'NONE',  ( 19.44145409300831417, 9.016062086884520710, -15.75081756649476894 ) ) ;
#17388=CARTESIAN_POINT ( 'NONE',  ( 18.58771872311928774, 0.01515834859250781048, -13.77226461354315035 ) ) ;
#17392=CARTESIAN_POINT ( 'NONE',  ( 36.35800453371076202, -21.32829872614925648, -20.07395605779921155 ) ) ;
#17393=CARTESIAN_POINT ( 'NONE',  ( 14.39533340154967433, 6.572929804808670617, -18.54476805420031837 ) ) ;
#17400=CARTESIAN_POINT ( 'NONE',  ( 32.62126879184269512, -11.04717877266006987, -18.30218954475424908 ) ) ;
#17408=CARTESIAN_POINT ( 'NONE',  ( 11.95275185645256322, 10.98126796543430572, -15.44474055479659569 ) ) ;
#17412=CARTESIAN_POINT ( 'NONE',  ( 12.49271550807400999, 8.567542729147559655, -15.13597632865050535 ) ) ;
#17414=CARTESIAN_POINT ( 'NONE',  ( 11.57911078346310774, 7.697743364462890980, -15.81898674067912225 ) ) ;
#17420=CARTESIAN_POINT ( 'NONE',  ( 12.83866652039362855, 9.525916288823983891, -16.13726486007240624 ) ) ;
#17422=CARTESIAN_POINT ( 'NONE',  ( 36.10807049912983757, -19.20547750251314767, -19.41448258861096932 ) ) ;
#17423=CARTESIAN_POINT ( 'NONE',  ( 18.76632379254337835, 6.868107169226369102, -19.55161205380106892 ) ) ;
#17427=CARTESIAN_POINT ( 'NONE',  ( 32.57950401048368150, -10.91418750421072659, -13.94906786461360504 ) ) ;
#17430=CARTESIAN_POINT ( 'NONE',  ( 19.55718041265476970, -1.390565517676688900, -17.79492730709450754 ) ) ;
#17431=CARTESIAN_POINT ( 'NONE',  ( 20.13453040791782911, -1.388291987844697317, -13.01173725324373009 ) ) ;
#17445=CARTESIAN_POINT ( 'NONE',  ( 11.44040408106239326, 9.418203516307107392, -15.87434068686103394 ) ) ;
#17447=CARTESIAN_POINT ( 'NONE',  ( 16.77165338796101324, 10.12286561294300569, -15.51291369241808304 ) ) ;
#17448=CARTESIAN_POINT ( 'NONE',  ( 26.69342817538273138, -7.978421288772274522, -19.59580293194042966 ) ) ;
#17457=CARTESIAN_POINT ( 'NONE',  ( 19.18841159021359033, -2.222386543571284179, -18.22349448661670834 ) ) ;
#17460=CARTESIAN_POINT ( 'NONE',  ( 12.27434273475605409, 9.502313893772186049, -15.31206391052669602 ) ) ;
#17463=CARTESIAN_POINT ( 'NONE',  ( 19.02541433733466647, 1.263421280649871248, -13.57496312174407826 ) ) ;
#17466=CARTESIAN_POINT ( 'NONE',  ( 20.44834407054411685, 8.573499863981592028, -15.78670165415130100 ) ) ;
#17469=CARTESIAN_POINT ( 'NONE',  ( 23.62051642037636157, -5.854316150849339984, -13.42181569741374503 ) ) ;
#17470=CARTESIAN_POINT ( 'NONE',  ( 27.64697528205969590, -2.889103667904926898, -18.32829528246118755 ) ) ;
#17472=CARTESIAN_POINT ( 'NONE',  ( 27.01132674553606350, -11.00696853675122711, -18.49859303458091730 ) ) ;
#17485=CARTESIAN_POINT ( 'NONE',  ( 25.76085037594245719, -3.206535967183471669, -15.98314152415894540 ) ) ;
#17487=CARTESIAN_POINT ( 'NONE',  ( 36.52322468491136220, -22.07054534594105988, -19.04503427665075321 ) ) ;
#17488=CARTESIAN_POINT ( 'NONE',  ( 9.916336358462064737, 16.40777236560037622, -16.50459729666445696 ) ) ;
#17491=CARTESIAN_POINT ( 'NONE',  ( 13.12489394565217005, 8.571418981294288031, -15.91088741739120671 ) ) ;
#17503=CARTESIAN_POINT ( 'NONE',  ( 8.944584764616054784, 16.95159238827779546, -17.91493351301869552 ) ) ;
#17504=CARTESIAN_POINT ( 'NONE',  ( 13.09464261414706066, 5.717622835290344874, -15.96348941799783816 ) ) ;
#17505=CARTESIAN_POINT ( 'NONE',  ( 28.96558774451377971, -5.053040458581501859, -15.93506438242870971 ) ) ;
#17518=CARTESIAN_POINT ( 'NONE',  ( 13.12489394565217005, 8.571418981294288031, -15.91088741739120671 ) ) ;
#17520=CARTESIAN_POINT ( 'NONE',  ( 35.54859390953724585, -22.18451583373416014, -18.19919658220850778 ) ) ;
#17521=CARTESIAN_POINT ( 'NONE',  ( 10.40934825891211979, 10.23400028951819607, -16.51844484289298265 ) ) ;
#17524=CARTESIAN_POINT ( 'NONE',  ( 24.66978787416869068, -0.3063955544261361963, -14.42797892638687784 ) ) ;
#17525=CARTESIAN_POINT ( 'NONE',  ( 10.35864919943752405, 16.97212496474457311, -17.91550491156534974 ) ) ;
#17529=CARTESIAN_POINT ( 'NONE',  ( 11.77869587587188249, 8.711114196793760200, -15.67004689359726299 ) ) ;
#17535=CARTESIAN_POINT ( 'NONE',  ( 13.10707286029108865, 8.563798077496334926, -15.92507172258792281 ) ) ;
#17538=CARTESIAN_POINT ( 'NONE',  ( 18.23272808550097679, 0.7689261898593379163, -20.18852386690180367 ) ) ;
#17539=CARTESIAN_POINT ( 'NONE',  ( 19.58395429099637752, 5.031901065175194532, -13.05446103591450147 ) ) ;
#17544=CARTESIAN_POINT ( 'NONE',  ( 36.54859390953724585, -22.18451583373416014, -17.99055332684694974 ) ) ;
#17548=CARTESIAN_POINT ( 'NONE',  ( 16.09764958744793262, 8.143416238145906760, -19.84970969296679044 ) ) ;
#17556=CARTESIAN_POINT ( 'NONE',  ( 32.74314609665832165, -11.10724048739539782, -18.62249297335446840 ) ) ;
#17560=CARTESIAN_POINT ( 'NONE',  ( 11.05541548581436118, 17.68942261459453036, -17.91440211708152574 ) ) ;
#17565=CARTESIAN_POINT ( 'NONE',  ( 11.03967536873724242, 8.192193740582544237, -16.19303379925286279 ) ) ;
#17571=CARTESIAN_POINT ( 'NONE',  ( 12.83257874964047929, 9.539242390270068483, -16.14089537112711525 ) ) ;
#17573=CARTESIAN_POINT ( 'NONE',  ( 34.64580997985590471, -12.63631557036062247, -18.97247631304233195 ) ) ;
#17574=CARTESIAN_POINT ( 'NONE',  ( 21.94319337455657859, -4.318501116253552041, -18.82930321547734920 ) ) ;
#17578=CARTESIAN_POINT ( 'NONE',  ( 18.68520274485960542, 10.62608585526774441, -17.78552708330943588 ) ) ;
#17584=CARTESIAN_POINT ( 'NONE',  ( 21.55249387529322647, -4.041031698679099726, -14.19001464829599435 ) ) ;
#17586=CARTESIAN_POINT ( 'NONE',  ( 17.18298215709098287, 1.908350159885260799, -18.42911670940388902 ) ) ;
#17597=CARTESIAN_POINT ( 'NONE',  ( 11.22146363488324283, 9.102391324313689580, -17.24260967991309101 ) ) ;
#17598=CARTESIAN_POINT ( 'NONE',  ( 10.17605321708455257, 15.21667774575863419, -16.39719424528293246 ) ) ;
#17599=CARTESIAN_POINT ( 'NONE',  ( 30.58006126958193249, -8.114715823802763239, -15.12008790671442426 ) ) ;
#17607=CARTESIAN_POINT ( 'NONE',  ( 21.69765170278760280, -5.035756590920279940, -14.89200278627170881 ) ) ;
#17610=CARTESIAN_POINT ( 'NONE',  ( 12.27690927615027583, 9.494639109526119114, -15.31069018153633721 ) ) ;
#17613=CARTESIAN_POINT ( 'NONE',  ( 26.85315702054868936, -3.432285194908070380, -17.01323758698984889 ) ) ;
#17615=CARTESIAN_POINT ( 'NONE',  ( 17.78670086218314239, 4.747145650100266678, -21.23922340053293212 ) ) ;
#17619=CARTESIAN_POINT ( 'NONE',  ( 28.48873154519036888, -4.568419848414010609, -17.42663535687301035 ) ) ;
#17620=CARTESIAN_POINT ( 'NONE',  ( 23.77355757633466382, -7.879698323813751237, -13.16654918938113283 ) ) ;
#17634=CARTESIAN_POINT ( 'NONE',  ( 23.80376867147650444, -3.845223433682474212, -14.48388124448521452 ) ) ;
#17635=CARTESIAN_POINT ( 'NONE',  ( 16.94700227795405212, 10.49100606271714931, -14.51747230701220559 ) ) ;
#17636=CARTESIAN_POINT ( 'NONE',  ( 34.83580697690636185, -15.48987143388560384, -21.11455094357481244 ) ) ;
#17638=CARTESIAN_POINT ( 'NONE',  ( 10.43540724046455992, 14.02724713458965233, -16.28994223329847202 ) ) ;
#17640=CARTESIAN_POINT ( 'NONE',  ( 9.661883064511089358, 16.25482662032373327, -17.91571053624716470 ) ) ;
#17643=CARTESIAN_POINT ( 'NONE',  ( 11.46877092736959014, 9.288109543210406827, -15.86260999805022820 ) ) ;
#17650=CARTESIAN_POINT ( 'NONE',  ( 8.944584683310379702, 16.95159276115599667, -17.98596209335946128 ) ) ;
#17651=CARTESIAN_POINT ( 'NONE',  ( 31.38423252821215570, -10.20947814759437655, -16.80760986317607930 ) ) ;
#17653=CARTESIAN_POINT ( 'NONE',  ( 25.97279949409942290, -11.71600155862194015, -18.85018042282848683 ) ) ;
#17655=CARTESIAN_POINT ( 'NONE',  ( 27.85014272824177795, -5.137623357037004013, -13.74226875356335320 ) ) ;
#17670=CARTESIAN_POINT ( 'NONE',  ( 12.02841764901576838, 9.314357472305010432, -16.69117924060192948 ) ) ;
#17671=CARTESIAN_POINT ( 'NONE',  ( 33.23735339574943026, -11.79161913663336314, -18.04114522998021997 ) ) ;
#17673=CARTESIAN_POINT ( 'NONE',  ( 9.132840175088396961, 16.08822907886823472, -17.04632583937691592 ) ) ;
#17676=CARTESIAN_POINT ( 'NONE',  ( 24.14158683625483803, -3.940216521628096658, -13.50644477367014673 ) ) ;
#17677=CARTESIAN_POINT ( 'NONE',  ( 17.21732962576914616, 11.43796928512929867, -12.64914394394206454 ) ) ;
#17682=CARTESIAN_POINT ( 'NONE',  ( 11.69419402147360110, 8.800013620902292999, -15.72776802682527730 ) ) ;
#17687=CARTESIAN_POINT ( 'NONE',  ( 9.661883135045433946, 16.25482629684424296, -17.91562380025844803 ) ) ;
#17689=CARTESIAN_POINT ( 'NONE',  ( 14.60232135752762517, 2.980368010496468933, -17.13315712471359475 ) ) ;
#17690=CARTESIAN_POINT ( 'NONE',  ( 19.51424001318473245, 7.885341048999412017, -19.79681821819610832 ) ) ;
#17693=CARTESIAN_POINT ( 'NONE',  ( 19.07848178107829540, -2.338951347401693859, -17.85627120065723616 ) ) ;
#17699=CARTESIAN_POINT ( 'NONE',  ( 32.58918748260075660, -11.04229556371213583, -18.21152344180378080 ) ) ;
#17705=CARTESIAN_POINT ( 'NONE',  ( 12.51736351114195500, 9.636405190433555035, -15.11633598780129439 ) ) ;
#17706=CARTESIAN_POINT ( 'NONE',  ( 35.09535884372434111, -21.14837076832613860, -21.10414782775458420 ) ) ;
#17711=CARTESIAN_POINT ( 'NONE',  ( 12.93612603019711571, 8.763434079353435990, -14.78257486846209368 ) ) ;
#17714=CARTESIAN_POINT ( 'NONE',  ( 10.62817821613907476, 9.230418211344437296, -16.42795095778131298 ) ) ;
#17719=CARTESIAN_POINT ( 'NONE',  ( 12.88201729092779857, 9.522117202545773651, -16.10446439827067167 ) ) ;
#17720=CARTESIAN_POINT ( 'NONE',  ( 32.96976325559394638, -10.97479806523316448, -15.05356414682637833 ) ) ;
#17721=CARTESIAN_POINT ( 'NONE',  ( 23.16390915794477223, 2.882539813099532555, -14.99485278278146438 ) ) ;
#17727=CARTESIAN_POINT ( 'NONE',  ( 26.00956027078203192, -8.595392566010074731, -19.46287731774799212 ) ) ;
#17728=CARTESIAN_POINT ( 'NONE',  ( 18.10326352236751646, 1.905885860032081158, -14.21403189877281825 ) ) ;
#17739=CARTESIAN_POINT ( 'NONE',  ( 11.32192133241855103, 8.753083428987814330, -17.19257025691282337 ) ) ;
#17741=CARTESIAN_POINT ( 'NONE',  ( 10.33811693838771717, 18.38618951776012267, -17.91664992932185996 ) ) ;
#17754=CARTESIAN_POINT ( 'NONE',  ( 20.39549844898813191, -2.061726703908969505, -13.85117726305786512 ) ) ;
#17758=CARTESIAN_POINT ( 'NONE',  ( 15.36220012886423447, 10.89358938796158149, -12.84895098869522201 ) ) ;
#17761=CARTESIAN_POINT ( 'NONE',  ( 27.78884322698630882, -6.380937659459246625, -17.89340433249687834 ) ) ;
#17764=CARTESIAN_POINT ( 'NONE',  ( 19.88777865313588222, 4.107626486979258473, -13.29018489620430721 ) ) ;
#17768=CARTESIAN_POINT ( 'NONE',  ( 18.16551323082808267, 7.152368624112494189, -14.07085781252208712 ) ) ;
#17769=CARTESIAN_POINT ( 'NONE',  ( 23.88957251509086888, -3.236156964677408876, -12.29669325917074829 ) ) ;
#17778=CARTESIAN_POINT ( 'NONE',  ( 25.68863286643039601, -3.692565893519352827, -17.49701707463368550 ) ) ;
#17780=CARTESIAN_POINT ( 'NONE',  ( 35.69176435403931436, -19.33523451612313693, -21.37328632439622922 ) ) ;
#17782=CARTESIAN_POINT ( 'NONE',  ( 12.49428694376680049, 8.568214790255201052, -15.13472557389765072 ) ) ;
#17788=CARTESIAN_POINT ( 'NONE',  ( 9.661901852922078149, 16.25474045427587200, -17.91339448853296901 ) ) ;
#17791=CARTESIAN_POINT ( 'NONE',  ( 11.45661370752365116, 9.343864103108954211, -15.86763743611193789 ) ) ;
#17795=CARTESIAN_POINT ( 'NONE',  ( 14.03850921439652311, 8.975161913830900673, -15.18271992443145635 ) ) ;
#17797=CARTESIAN_POINT ( 'NONE',  ( 16.49632153860815720, 9.003283391651189405, -13.22380011606493788 ) ) ;
#17798=CARTESIAN_POINT ( 'NONE',  ( 35.88008189734257769, -20.18124548360443882, -21.42481968387543390 ) ) ;
#17799=CARTESIAN_POINT ( 'NONE',  ( 17.49446177548951553, 10.34313653870878547, -20.19723249710358104 ) ) ;
#17800=CARTESIAN_POINT ( 'NONE',  ( 28.12627659338356878, -5.062120396530918498, -14.05642262879015369 ) ) ;
#17805=CARTESIAN_POINT ( 'NONE',  ( 21.97327598498023704, 3.176719406474355800, -15.71098195781089046 ) ) ;
#17812=CARTESIAN_POINT ( 'NONE',  ( 12.03055882466574289, 9.304755949677762317, -16.69027714870545864 ) ) ;
#17813=CARTESIAN_POINT ( 'NONE',  ( 35.19403856461168090, -19.59168648217519504, -19.20845343762490032 ) ) ;
#17816=CARTESIAN_POINT ( 'NONE',  ( 9.114604345319493817, 16.17186091871610287, -17.05386699646955861 ) ) ;
#17820=CARTESIAN_POINT ( 'NONE',  ( 28.16462234717350199, -5.661059359726887230, -16.30864077692347536 ) ) ;
#17822=CARTESIAN_POINT ( 'NONE',  ( 12.86812980024498643, 9.515982172609518841, -16.11553281326163045 ) ) ;
#17832=CARTESIAN_POINT ( 'NONE',  ( 9.661883795922106444, 16.25482326597959926, -17.91529654610192424 ) ) ;
#17833=CARTESIAN_POINT ( 'NONE',  ( 16.15008960989130671, 4.591438144365319829, -20.60273134265763062 ) ) ;
#17834=CARTESIAN_POINT ( 'NONE',  ( 19.44145409300831417, 9.016062086884520710, -15.75081756649476894 ) ) ;
#17839=CARTESIAN_POINT ( 'NONE',  ( 23.66601916330066402, 2.199037240492611733, -18.57254039386976885 ) ) ;
#17845=CARTESIAN_POINT ( 'NONE',  ( 35.18065281855160720, -20.53155141575438591, -20.22037173032050461 ) ) ;
#17851=CARTESIAN_POINT ( 'NONE',  ( 12.25364105430271700, 9.519861518574414205, -15.32652744092241726 ) ) ;
#17852=CARTESIAN_POINT ( 'NONE',  ( 35.54859390953724585, -23.18451583373416014, -16.11276402859391510 ) ) ;
#17858=CARTESIAN_POINT ( 'NONE',  ( 10.66363677402306287, 9.067800744973538940, -16.41328759676781246 ) ) ;
#17862=CARTESIAN_POINT ( 'NONE',  ( 12.86796368952119174, 9.515911916162036022, -16.11566496612908139 ) ) ;
#17863=CARTESIAN_POINT ( 'NONE',  ( 33.25614251967556356, -10.36847857886694868, -17.86465469861353483 ) ) ;
#17864=CARTESIAN_POINT ( 'NONE',  ( 21.40051611374530793, -0.1690565882708310874, -20.18282279970310000 ) ) ;
#17869=CARTESIAN_POINT ( 'NONE',  ( 23.54468722040186890, -6.934586491718037315, -13.40271233150634878 ) ) ;
#17870=CARTESIAN_POINT ( 'NONE',  ( 24.72855373928933531, -1.476844508782828802, -20.15487193605729033 ) ) ;
#17879=( BOUNDED_SURFACE ( )  B_SPLINE_SURFACE ( 3, 3, ( 
 ( #18762, #158, #26249, #7025, #2909, #7175, #23811, #7616, #2751, #23346, #609, #21194, #14470, #16466, #9291, #2460, #5336, #28270, #16920, #11735, #23969, #25793, #2606, #21052, #20894, #28418, #5, #12038, #25632, #9896, #16315, #18616, #9436, #28115, #25943, #26099, #4874, #23496, #16624, #11881, #9594, #5024, #14315, #23650, #21352, #19064, #458, #9744, #7472, #16775, #5178, #26403, #3503, #17367, #22111, #14917, #26874, #905, #12333, #10351, #29021, #7915, #24556, #17078, #5482, #12793, #14765, #8365, #17520, #24106, #8057, #26714, #5939, #3206, #5786, #15069, #22257, #26553 ),
 ( #3354, #10495, #3648, #1365, #19356, #12484, #12641, #19656, #21808, #15223, #19807, #12943, #24407, #24257, #17671, #10655, #21959, #5637, #29337, #10197, #19967, #19509, #1213, #745, #27028, #17226, #10043, #6083, #15379, #1071, #28883, #3058, #29169, #21647, #8208, #28717, #7765, #1672, #13252, #9101, #20116, #15981, #20259, #6692, #2125, #15827, #17813, #25308, #4101, #27626, #29645, #22419, #27186, #18429, #11105, #11396, #6239, #27779, #8662, #15685, #15534, #6844, #11257, #3801, #25156, #8515, #13698, #29496, #24713, #20703, #13091, #8811, #8954, #24866, #17967, #20411, #22572, #3953 ),
 ( #22721, #27340, #30091, #29803, #1523, #10806, #10952, #6394, #20559, #25014, #13394, #22868, #1825, #29944, #18119, #23022, #27484, #6538, #4249, #13544, #1977, #18270, #4398, #4990, #16132, #28233, #12154, #9554, #5141, #30239, #14431, #23157, #14136, #16433, #28386, #9704, #20856, #19030, #11997, #21313, #28533, #422, #16589, #9251, #23774, #28077, #25590, #11699, #18579, #14281, #25755, #4837, #25454, #18875, #272, #7286, #25913, #4544, #2271, #23464, #7133, #7441, #4684, #23614, #2422, #11847, #2710, #16743, #9401, #18730, #2574, #13978, #23308, #21015, #26066, #13834, #2870, #21469 ),
 ( #19176, #11541, #27927, #577, #6989, #16278, #9863, #120, #21158, #17192, #26836, #17043, #16885, #8025, #874, #28846, #22078, #26215, #26678, #7582, #19622, #3614, #1033, #5907, #21618, #15189, #14583, #5601, #7884, #19766, #1180, #12301, #10461, #3464, #12754, #19930, #29136, #17333, #715, #24521, #19473, #26371, #3177, #10008, #5755, #26519, #14880, #5299, #10314, #21920, #28988, #15037, #23933, #3025, #24225, #3325, #8175, #5450, #24369, #24074, #12604, #17487, #12906, #10162, #22220, #1329, #10621, #19322, #28682, #12448, #7731, #14731, #21773, #13509, #27140, #15338, #24827, #25272 ),
 ( #24675, #27303, #15945, #1940, #27451, #13215, #10776, #4211, #17927, #25121, #1637, #6357, #26992, #22382, #13661, #15651, #6651, #1486, #22985, #22539, #20225, #20085, #2088, #15794, #8333, #20374, #13058, #18235, #3765, #11365, #4359, #29296, #13359, #22836, #29461, #3916, #24983, #10916, #11222, #6203, #17636, #4066, #22684, #29611, #20525, #8479, #17780, #29764, #15496, #6049, #29912, #8627, #1785, #11071, #8921, #8773, #18088, #6503, #27593, #13946, #4959, #9215, #23580, #20977, #28201, #11962, #18999, #6805, #13799, #87, #28043, #18542, #14249, #7258, #390, #14098, #11663, #5107 ),
 ( #2544, #4805, #2836, #16095, #9368, #18698, #2677, #30206, #21130, #6958, #16399, #11815, #21279, #23275, #2390, #7099, #25723, #23431, #241, #16246, #9676, #4510, #30055, #28356, #27897, #25421, #25558, #16712, #7412, #9518, #18840, #23125, #16556, #26033, #14398, #25880, #4653, #2236, #23739, #20670, #9065, #18390, #27745, #11506, #20822, #26333, #10842, #12122, #29377, #19146, #21437, #9975, #7551, #8401, #5567, #28503, #17706, #16855, #27067, #14846, #23898, #19438, #22464, #13132, #28810, #688, #6122, #1562, #26183, #29532, #24905, #19290, #15420, #10127, #5416, #17852, #7848, #8549 ),
 ( #5263, #12565, #26486, #997, #24044, #24754, #28647, #549, #17157, #24189, #17010, #3840, #14551, #2995, #21884, #12271, #27228, #20150, #21589, #3290, #10278, #6278, #7698, #20009, #15571, #9830, #14701, #3142, #12417, #21733, #836, #11436, #25499, #2317, #20298, #27381, #4289, #11297, #22759, #27822, #20746, #13878, #27668, #25199, #18624, #4588, #13591, #27526, #12, #18012, #11587, #1871, #13736, #1707, #30135, #2018, #20901, #11150, #20452, #8850, #6731, #10990, #15869, #15725, #9299, #18165, #29686, #23200, #27972, #6581, #6433, #16178, #29845, #6889, #20601, #22915, #23063, #29984 ) ),
 .UNSPECIFIED., .T., .F., .F. ) 
 B_SPLINE_SURFACE_WITH_KNOTS ( ( 4, 3, 4 ),
 ( 4, 2, 2, 2, 2, 2, 2, 2, 2, 2, 2, 2, 2, 2, 2, 2, 2, 2, 2, 2, 2, 2, 2, 2, 2, 2, 2, 2, 2, 2, 2, 2, 2, 2, 2, 2, 2, 2, 4 ),
 ( 0.000000000000000000, 0.5000000000000000000, 1.000000000000000000 ),
 ( 0.000000000000000000, 0.1003381136405422785, 0.1505071704608134109, 0.1755916988709489979, 0.1881339630760167636, 0.1944050951785506465, 0.2006762272810845571, 0.2086934065084689038, 0.2167105857358532783, 0.2327449441906219718, 0.2648136611001593588, 0.2968823780096967457, 0.3129167364644654947, 0.3209339156918498137, 0.3289510949192341882, 0.3346579968240730452, 0.3403648987289118466, 0.3517787025385894495, 0.3746063101579446553, 0.4202615253966550668, 0.5115719558740758899, 0.6028823863514967130, 0.6485376015902071245, 0.6713652092095623303, 0.6827790130192399332, 0.6941928168289175360, 0.7036545619149295883, 0.7131163070009416405, 0.7320397971729657449, 0.7698867775170139538, 0.8077337578610621627, 0.8266572480330862671, 0.8361189931190984304, 0.8455807382051104826, 0.8552319420672911399, 0.8648831459294716861, 0.8841855536538327787, 0.9227903691025551858, 1.000000000000000000 ),
 .UNSPECIFIED. ) 
 GEOMETRIC_REPRESENTATION_ITEM ( )  RATIONAL_B_SPLINE_SURFACE ( (
 ( 1.000000000000000000, 1.000000000000000000, 1.000000000000000000, 1.000000000000000000, 1.000000000000000000, 1.000000000000000000, 1.000000000000000000, 1.000000000000000000, 1.000000000000000000, 1.000000000000000000, 1.000000000000000000, 1.000000000000000000, 1.000000000000000000, 1.000000000000000000, 1.000000000000000000, 1.000000000000000000, 1.000000000000000000, 1.000000000000000000, 1.000000000000000000, 1.000000000000000000, 1.000000000000000000, 1.000000000000000000, 1.000000000000000000, 1.000000000000000000, 1.000000000000000000, 1.000000000000000000, 1.000000000000000000, 1.000000000000000000, 1.000000000000000000, 1.000000000000000000, 1.000000000000000000, 1.000000000000000000, 1.000000000000000000, 1.000000000000000000, 1.000000000000000000, 1.000000000000000000, 1.000000000000000000, 1.000000000000000000, 1.000000000000000000, 1.000000000000000000, 1.000000000000000000, 1.000000000000000000, 1.000000000000000000, 1.000000000000000000, 1.000000000000000000, 1.000000000000000000, 1.000000000000000000, 1.000000000000000000, 1.000000000000000000, 1.000000000000000000, 1.000000000000000000, 1.000000000000000000, 1.000000000000000000, 1.000000000000000000, 1.000000000000000000, 1.000000000000000000, 1.000000000000000000, 1.000000000000000000, 1.000000000000000000, 1.000000000000000000, 1.000000000000000000, 1.000000000000000000, 1.000000000000000000, 1.000000000000000000, 1.000000000000000000, 1.000000000000000000, 1.000000000000000000, 1.000000000000000000, 1.000000000000000000, 1.000000000000000000, 1.000000000000000000, 1.000000000000000000, 1.000000000000000000, 1.000000000000000000, 1.000000000000000000, 1.000000000000000000, 1.000000000000000000, 1.000000000000000000),
 ( 0.3333333333333333703, 0.3333333333333333703, 0.3333333333333333703, 0.3333333333333333703, 0.3333333333333333703, 0.3333333333333333703, 0.3333333333333333703, 0.3333333333333333703, 0.3333333333333333703, 0.3333333333333333703, 0.3333333333333333703, 0.3333333333333333703, 0.3333333333333333703, 0.3333333333333333703, 0.3333333333333333703, 0.3333333333333333703, 0.3333333333333333703, 0.3333333333333333703, 0.3333333333333333703, 0.3333333333333333703, 0.3333333333333333703, 0.3333333333333333703, 0.3333333333333333703, 0.3333333333333333703, 0.3333333333333333703, 0.3333333333333333703, 0.3333333333333333703, 0.3333333333333333703, 0.3333333333333333703, 0.3333333333333333703, 0.3333333333333333703, 0.3333333333333333703, 0.3333333333333333703, 0.3333333333333333703, 0.3333333333333333703, 0.3333333333333333703, 0.3333333333333333703, 0.3333333333333333703, 0.3333333333333333703, 0.3333333333333333703, 0.3333333333333333703, 0.3333333333333333703, 0.3333333333333333703, 0.3333333333333333703, 0.3333333333333333703, 0.3333333333333333703, 0.3333333333333333703, 0.3333333333333333703, 0.3333333333333333703, 0.3333333333333333703, 0.3333333333333333703, 0.3333333333333333703, 0.3333333333333333703, 0.3333333333333333703, 0.3333333333333333703, 0.3333333333333333703, 0.3333333333333333703, 0.3333333333333333703, 0.3333333333333333703, 0.3333333333333333703, 0.3333333333333333703, 0.3333333333333333703, 0.3333333333333333703, 0.3333333333333333703, 0.3333333333333333703, 0.3333333333333333703, 0.3333333333333333703, 0.3333333333333333703, 0.3333333333333333703, 0.3333333333333333703, 0.3333333333333333703, 0.3333333333333333703, 0.3333333333333333703, 0.3333333333333333703, 0.3333333333333333703, 0.3333333333333333703, 0.3333333333333333703, 0.3333333333333333703),
 ( 0.3333333333333333703, 0.3333333333333333703, 0.3333333333333333703, 0.3333333333333333703, 0.3333333333333333703, 0.3333333333333333703, 0.3333333333333333703, 0.3333333333333333703, 0.3333333333333333703, 0.3333333333333333703, 0.3333333333333333703, 0.3333333333333333703, 0.3333333333333333703, 0.3333333333333333703, 0.3333333333333333703, 0.3333333333333333703, 0.3333333333333333703, 0.3333333333333333703, 0.3333333333333333703, 0.3333333333333333703, 0.3333333333333333703, 0.3333333333333333703, 0.3333333333333333703, 0.3333333333333333703, 0.3333333333333333703, 0.3333333333333333703, 0.3333333333333333703, 0.3333333333333333703, 0.3333333333333333703, 0.3333333333333333703, 0.3333333333333333703, 0.3333333333333333703, 0.3333333333333333703, 0.3333333333333333703, 0.3333333333333333703, 0.3333333333333333703, 0.3333333333333333703, 0.3333333333333333703, 0.3333333333333333703, 0.3333333333333333703, 0.3333333333333333703, 0.3333333333333333703, 0.3333333333333333703, 0.3333333333333333703, 0.3333333333333333703, 0.3333333333333333703, 0.3333333333333333703, 0.3333333333333333703, 0.3333333333333333703, 0.3333333333333333703, 0.3333333333333333703, 0.3333333333333333703, 0.3333333333333333703, 0.3333333333333333703, 0.3333333333333333703, 0.3333333333333333703, 0.3333333333333333703, 0.3333333333333333703, 0.3333333333333333703, 0.3333333333333333703, 0.3333333333333333703, 0.3333333333333333703, 0.3333333333333333703, 0.3333333333333333703, 0.3333333333333333703, 0.3333333333333333703, 0.3333333333333333703, 0.3333333333333333703, 0.3333333333333333703, 0.3333333333333333703, 0.3333333333333333703, 0.3333333333333333703, 0.3333333333333333703, 0.3333333333333333703, 0.3333333333333333703, 0.3333333333333333703, 0.3333333333333333703, 0.3333333333333333703),
 ( 1.000000000000000000, 1.000000000000000000, 1.000000000000000000, 1.000000000000000000, 1.000000000000000000, 1.000000000000000000, 1.000000000000000000, 1.000000000000000000, 1.000000000000000000, 1.000000000000000000, 1.000000000000000000, 1.000000000000000000, 1.000000000000000000, 1.000000000000000000, 1.000000000000000000, 1.000000000000000000, 1.000000000000000000, 1.000000000000000000, 1.000000000000000000, 1.000000000000000000, 1.000000000000000000, 1.000000000000000000, 1.000000000000000000, 1.000000000000000000, 1.000000000000000000, 1.000000000000000000, 1.000000000000000000, 1.000000000000000000, 1.000000000000000000, 1.000000000000000000, 1.000000000000000000, 1.000000000000000000, 1.000000000000000000, 1.000000000000000000, 1.000000000000000000, 1.000000000000000000, 1.000000000000000000, 1.000000000000000000, 1.000000000000000000, 1.000000000000000000, 1.000000000000000000, 1.000000000000000000, 1.000000000000000000, 1.000000000000000000, 1.000000000000000000, 1.000000000000000000, 1.000000000000000000, 1.000000000000000000, 1.000000000000000000, 1.000000000000000000, 1.000000000000000000, 1.000000000000000000, 1.000000000000000000, 1.000000000000000000, 1.000000000000000000, 1.000000000000000000, 1.000000000000000000, 1.000000000000000000, 1.000000000000000000, 1.000000000000000000, 1.000000000000000000, 1.000000000000000000, 1.000000000000000000, 1.000000000000000000, 1.000000000000000000, 1.000000000000000000, 1.000000000000000000, 1.000000000000000000, 1.000000000000000000, 1.000000000000000000, 1.000000000000000000, 1.000000000000000000, 1.000000000000000000, 1.000000000000000000, 1.000000000000000000, 1.000000000000000000, 1.000000000000000000, 1.000000000000000000),
 ( 0.3333333333333333703, 0.3333333333333333703, 0.3333333333333333703, 0.3333333333333333703, 0.3333333333333333703, 0.3333333333333333703, 0.3333333333333333703, 0.3333333333333333703, 0.3333333333333333703, 0.3333333333333333703, 0.3333333333333333703, 0.3333333333333333703, 0.3333333333333333703, 0.3333333333333333703, 0.3333333333333333703, 0.3333333333333333703, 0.3333333333333333703, 0.3333333333333333703, 0.3333333333333333703, 0.3333333333333333703, 0.3333333333333333703, 0.3333333333333333703, 0.3333333333333333703, 0.3333333333333333703, 0.3333333333333333703, 0.3333333333333333703, 0.3333333333333333703, 0.3333333333333333703, 0.3333333333333333703, 0.3333333333333333703, 0.3333333333333333703, 0.3333333333333333703, 0.3333333333333333703, 0.3333333333333333703, 0.3333333333333333703, 0.3333333333333333703, 0.3333333333333333703, 0.3333333333333333703, 0.3333333333333333703, 0.3333333333333333703, 0.3333333333333333703, 0.3333333333333333703, 0.3333333333333333703, 0.3333333333333333703, 0.3333333333333333703, 0.3333333333333333703, 0.3333333333333333703, 0.3333333333333333703, 0.3333333333333333703, 0.3333333333333333703, 0.3333333333333333703, 0.3333333333333333703, 0.3333333333333333703, 0.3333333333333333703, 0.3333333333333333703, 0.3333333333333333703, 0.3333333333333333703, 0.3333333333333333703, 0.3333333333333333703, 0.3333333333333333703, 0.3333333333333333703, 0.3333333333333333703, 0.3333333333333333703, 0.3333333333333333703, 0.3333333333333333703, 0.3333333333333333703, 0.3333333333333333703, 0.3333333333333333703, 0.3333333333333333703, 0.3333333333333333703, 0.3333333333333333703, 0.3333333333333333703, 0.3333333333333333703, 0.3333333333333333703, 0.3333333333333333703, 0.3333333333333333703, 0.3333333333333333703, 0.3333333333333333703),
 ( 0.3333333333333333703, 0.3333333333333333703, 0.3333333333333333703, 0.3333333333333333703, 0.3333333333333333703, 0.3333333333333333703, 0.3333333333333333703, 0.3333333333333333703, 0.3333333333333333703, 0.3333333333333333703, 0.3333333333333333703, 0.3333333333333333703, 0.3333333333333333703, 0.3333333333333333703, 0.3333333333333333703, 0.3333333333333333703, 0.3333333333333333703, 0.3333333333333333703, 0.3333333333333333703, 0.3333333333333333703, 0.3333333333333333703, 0.3333333333333333703, 0.3333333333333333703, 0.3333333333333333703, 0.3333333333333333703, 0.3333333333333333703, 0.3333333333333333703, 0.3333333333333333703, 0.3333333333333333703, 0.3333333333333333703, 0.3333333333333333703, 0.3333333333333333703, 0.3333333333333333703, 0.3333333333333333703, 0.3333333333333333703, 0.3333333333333333703, 0.3333333333333333703, 0.3333333333333333703, 0.3333333333333333703, 0.3333333333333333703, 0.3333333333333333703, 0.3333333333333333703, 0.3333333333333333703, 0.3333333333333333703, 0.3333333333333333703, 0.3333333333333333703, 0.3333333333333333703, 0.3333333333333333703, 0.3333333333333333703, 0.3333333333333333703, 0.3333333333333333703, 0.3333333333333333703, 0.3333333333333333703, 0.3333333333333333703, 0.3333333333333333703, 0.3333333333333333703, 0.3333333333333333703, 0.3333333333333333703, 0.3333333333333333703, 0.3333333333333333703, 0.3333333333333333703, 0.3333333333333333703, 0.3333333333333333703, 0.3333333333333333703, 0.3333333333333333703, 0.3333333333333333703, 0.3333333333333333703, 0.3333333333333333703, 0.3333333333333333703, 0.3333333333333333703, 0.3333333333333333703, 0.3333333333333333703, 0.3333333333333333703, 0.3333333333333333703, 0.3333333333333333703, 0.3333333333333333703, 0.3333333333333333703, 0.3333333333333333703),
 ( 1.000000000000000000, 1.000000000000000000, 1.000000000000000000, 1.000000000000000000, 1.000000000000000000, 1.000000000000000000, 1.000000000000000000, 1.000000000000000000, 1.000000000000000000, 1.000000000000000000, 1.000000000000000000, 1.000000000000000000, 1.000000000000000000, 1.000000000000000000, 1.000000000000000000, 1.000000000000000000, 1.000000000000000000, 1.000000000000000000, 1.000000000000000000, 1.000000000000000000, 1.000000000000000000, 1.000000000000000000, 1.000000000000000000, 1.000000000000000000, 1.000000000000000000, 1.000000000000000000, 1.000000000000000000, 1.000000000000000000, 1.000000000000000000, 1.000000000000000000, 1.000000000000000000, 1.000000000000000000, 1.000000000000000000, 1.000000000000000000, 1.000000000000000000, 1.000000000000000000, 1.000000000000000000, 1.000000000000000000, 1.000000000000000000, 1.000000000000000000, 1.000000000000000000, 1.000000000000000000, 1.000000000000000000, 1.000000000000000000, 1.000000000000000000, 1.000000000000000000, 1.000000000000000000, 1.000000000000000000, 1.000000000000000000, 1.000000000000000000, 1.000000000000000000, 1.000000000000000000, 1.000000000000000000, 1.000000000000000000, 1.000000000000000000, 1.000000000000000000, 1.000000000000000000, 1.000000000000000000, 1.000000000000000000, 1.000000000000000000, 1.000000000000000000, 1.000000000000000000, 1.000000000000000000, 1.000000000000000000, 1.000000000000000000, 1.000000000000000000, 1.000000000000000000, 1.000000000000000000, 1.000000000000000000, 1.000000000000000000, 1.000000000000000000, 1.000000000000000000, 1.000000000000000000, 1.000000000000000000, 1.000000000000000000, 1.000000000000000000, 1.000000000000000000, 1.000000000000000000) ) ) 
 REPRESENTATION_ITEM ( '' )  SURFACE ( )  );
#17882=CARTESIAN_POINT ( 'NONE',  ( 12.94178543664954972, 7.512178771719595360, -16.05074886939826939 ) ) ;
#17883=CARTESIAN_POINT ( 'NONE',  ( 12.49957999542663600, 8.570517509188613658, -15.13050969259218981 ) ) ;
#17884=CARTESIAN_POINT ( 'NONE',  ( 28.35369828010231785, -12.30166555976806464, -13.00196782638265169 ) ) ;
#17889=CARTESIAN_POINT ( 'NONE',  ( 9.641566850259106758, 17.66790035518494051, -17.86107206016944460 ) ) ;
#17894=CARTESIAN_POINT ( 'NONE',  ( 24.66978787416869068, -0.3063955544261361963, -14.42797892638687784 ) ) ;
#17898=CARTESIAN_POINT ( 'NONE',  ( 12.78959314398258940, 9.756708335562493062, -14.89936416525698526 ) ) ;
#17903=CARTESIAN_POINT ( 'NONE',  ( 26.87257363757477435, -3.324124212371978082, -16.68573618535388547 ) ) ;
#17905=CARTESIAN_POINT ( 'NONE',  ( 24.18628427323349328, -0.8779346998738073449, -17.06787597161793357 ) ) ;
#17909=CARTESIAN_POINT ( 'NONE',  ( 25.74126694659371495, -13.30326880535473322, -17.45270501867052104 ) ) ;
#17910=CARTESIAN_POINT ( 'NONE',  ( 29.62334656761623819, -11.49549692320935890, -13.92735753183835712 ) ) ;
#17915=CARTESIAN_POINT ( 'NONE',  ( 29.66490191837812773, -8.365349891895018430, -17.62461620872172574 ) ) ;
#17925=CARTESIAN_POINT ( 'NONE',  ( 25.85400256215867643, -3.413040292952954413, -16.90843739280879277 ) ) ;
#17926=CARTESIAN_POINT ( 'NONE',  ( 19.82332968365342296, 2.432204761014481242, -19.52120720162773537 ) ) ;
#17927=CARTESIAN_POINT ( 'NONE',  ( 32.57905638361870615, -9.615828745292011703, -17.95267489271534700 ) ) ;
#17931=CARTESIAN_POINT ( 'NONE',  ( 11.47155695691762212, 9.275332456566969697, -15.86145787682774078 ) ) ;
#17934=CARTESIAN_POINT ( 'NONE',  ( 13.66828981435543078, 8.811555337407297017, -15.47779131845255307 ) ) ;
#17938=CARTESIAN_POINT ( 'NONE',  ( 12.43696608443014284, 8.546664718661613591, -15.18012293544581226 ) ) ;
#17945=CARTESIAN_POINT ( 'NONE',  ( 8.946690830082905777, 16.94193370358561879, -17.78270686867927708 ) ) ;
#17946=CARTESIAN_POINT ( 'NONE',  ( 31.95629010954621663, -10.29636179124881679, -18.42443288805318247 ) ) ;
#17948=CARTESIAN_POINT ( 'NONE',  ( 19.77504133826384347, 1.335633644655777053, -20.04176789066487530 ) ) ;
#17949=CARTESIAN_POINT ( 'NONE',  ( 26.09074415779471323, -5.786596670875995940, -12.76770422508296932 ) ) ;
#17953=CARTESIAN_POINT ( 'NONE',  ( 25.20506945179333513, 0.8918220058822420304, -17.26233558910082166 ) ) ;
#17967=CARTESIAN_POINT ( 'NONE',  ( 35.54859390953724585, -21.18451583373416014, -16.94733705004010105 ) ) ;
#17970=CARTESIAN_POINT ( 'NONE',  ( 12.75399582221978889, 7.624919616107145970, -14.92773571455457216 ) ) ;
#17972=CARTESIAN_POINT ( 'NONE',  ( 25.97256211245905533, -8.171536508395311316, -18.54953510021574559 ) ) ;
#17974=CARTESIAN_POINT ( 'NONE',  ( 10.35864917552468611, 16.97212507441191320, -17.91611982430173455 ) ) ;
#17979=CARTESIAN_POINT ( 'NONE',  ( 12.71834232392635045, 8.667191563245470576, -14.95615232649864090 ) ) ;
#17984=CARTESIAN_POINT ( 'NONE',  ( 9.661885998671275289, 16.25481316389105402, -17.91482063482849441 ) ) ;
#17986=CARTESIAN_POINT ( 'NONE',  ( 25.05533511103952904, -1.369129923259265524, -16.98221401193426416 ) ) ;
#17987=CARTESIAN_POINT ( 'NONE',  ( 22.35254782987788147, 5.884919045556002537, -15.62344653218675283 ) ) ;
#17993=CARTESIAN_POINT ( 'NONE',  ( 19.18841159021359033, -2.222386543571284179, -18.22349448661670834 ) ) ;
#18000=EDGE_CURVE ( 'NONE', #14962, #2433, #186, .T. ) ;
#18005=CARTESIAN_POINT ( 'NONE',  ( 33.47012763672258728, -12.84706786418751534, -19.72967806864707541 ) ) ;
#18010=CARTESIAN_POINT ( 'NONE',  ( 30.43753979984721525, -10.17066761781405937, -14.50402091508011537 ) ) ;
#18011=CARTESIAN_POINT ( 'NONE',  ( 12.24557421509628519, 9.516296637964343219, -15.33295685416265286 ) ) ;
#18012=CARTESIAN_POINT ( 'NONE',  ( 35.07504771885155037, -20.05712364337910714, -20.21480690768607857 ) ) ;
#18018=CARTESIAN_POINT ( 'NONE',  ( 9.641350810849047548, 17.66889113945805789, -17.97192418671891190 ) ) ;
#18026=CARTESIAN_POINT ( 'NONE',  ( 10.35864927600819740, 16.97212461358170188, -17.91506874352199574 ) ) ;
#18027=CARTESIAN_POINT ( 'NONE',  ( 32.35289370704636980, -10.23129387835982129, -15.31177623828282108 ) ) ;
#18028=CARTESIAN_POINT ( 'NONE',  ( 21.63873165585565417, 2.424707942738766331, -13.54651715722292060 ) ) ;
#18032=CARTESIAN_POINT ( 'NONE',  ( 27.03959252790357581, -7.665547941290169476, -19.57376043866218041 ) ) ;
#18034=CARTESIAN_POINT ( 'NONE',  ( 24.43881766525553090, -7.056818123010307531, -19.17719463634885102 ) ) ;
#18044=CARTESIAN_POINT ( 'NONE',  ( 11.22879857168519813, 9.069188343361037852, -17.23954317433854300 ) ) ;
#18045=CARTESIAN_POINT ( 'NONE',  ( 12.77278825050581013, 8.691252192278360766, -14.91275796197543890 ) ) ;
#18053=CARTESIAN_POINT ( 'NONE',  ( 9.641364314812712166, 17.66882920855936590, -17.90209449470656722 ) ) ;
#18055=CARTESIAN_POINT ( 'NONE',  ( 17.06308625499319831, 6.674173717519480853, -15.25088821959635865 ) ) ;
#18058=CARTESIAN_POINT ( 'NONE',  ( 24.14158683625483803, -3.940216521628096658, -13.50644477367014673 ) ) ;
#18062=CARTESIAN_POINT ( 'NONE',  ( 12.25326555804286421, 9.517817489571868350, -15.32696995758615621 ) ) ;
#18065=CARTESIAN_POINT ( 'NONE',  ( 35.54502023521215648, -22.16846120802060938, -18.59538644662325524 ) ) ;
#18067=CARTESIAN_POINT ( 'NONE',  ( 21.69765170278760280, -5.035756590920279940, -14.89200278627170881 ) ) ;
#18069=CARTESIAN_POINT ( 'NONE',  ( 21.26848706961299129, -1.060808783303755387, -18.71231287479539063 ) ) ;
#18073=CARTESIAN_POINT ( 'NONE',  ( 32.57950401048368150, -10.91418750421072659, -13.94906786461360504 ) ) ;
#18074=CARTESIAN_POINT ( 'NONE',  ( 30.18376337559066158, -9.479172175342087669, -16.86143889264288021 ) ) ;
#18086=CARTESIAN_POINT ( 'NONE',  ( 24.46642504186807088, -8.279991823955473507, -18.31266784446766493 ) ) ;
#18087=CARTESIAN_POINT ( 'NONE',  ( 19.92565466131104301, 6.686648131885553958, -19.16379146452587179 ) ) ;
#18088=CARTESIAN_POINT ( 'NONE',  ( 36.06101586692013683, -20.99408596552883566, -21.31372499146719690 ) ) ;
#18090=CARTESIAN_POINT ( 'NONE',  ( 12.49977518293622758, 8.570603418560722275, -15.13035415120363325 ) ) ;
#18093=CARTESIAN_POINT ( 'NONE',  ( 9.700291501659986437, 16.07868063162199945, -17.87166786738998780 ) ) ;
#18098=CARTESIAN_POINT ( 'NONE',  ( 12.53458732174692258, 8.585986940276173485, -15.10260830673100330 ) ) ;
#18106=CARTESIAN_POINT ( 'NONE',  ( 13.48814714115247249, 7.673917307032582791, -15.62136820872497545 ) ) ;
#18107=CARTESIAN_POINT ( 'NONE',  ( 35.94849409650817762, -20.48858525550898335, -21.40790205994406747 ) ) ;
#18108=CARTESIAN_POINT ( 'NONE',  ( 18.99162967131814028, 0.6168208955672017657, -19.54819510397825510 ) ) ;
#18109=CARTESIAN_POINT ( 'NONE',  ( 14.93998017692337221, 5.301442995092576105, -18.84457556472494488 ) ) ;
#18111=CARTESIAN_POINT ( 'NONE',  ( 24.97326132480219485, 0.3353791038140019887, -18.64228740943764961 ) ) ;
#18119=CARTESIAN_POINT ( 'NONE',  ( 33.96051107771264554, -11.12695408846492739, -17.85276550113785277 ) ) ;
#18121=CARTESIAN_POINT ( 'NONE',  ( 10.66927416475804158, 9.041953549878499530, -16.41095583421565962 ) ) ;
#18124=CARTESIAN_POINT ( 'NONE',  ( 29.66490191837812773, -8.365349891895018430, -17.62461620872172574 ) ) ;
#18126=CARTESIAN_POINT ( 'NONE',  ( 12.87691298531170148, 9.519861518574414205, -16.10853261994384411 ) ) ;
#18134=CARTESIAN_POINT ( 'NONE',  ( 12.50906579366657390, 8.574708520419219937, -15.12294941509656354 ) ) ;
#18142=CARTESIAN_POINT ( 'NONE',  ( 13.15105351193492744, 8.582979361647906202, -15.89003778131599098 ) ) ;
#18143=CARTESIAN_POINT ( 'NONE',  ( 17.73099166324444553, -0.3602181158183791476, -14.74723639357852178 ) ) ;
#18144=CARTESIAN_POINT ( 'NONE',  ( 22.18718699900398761, -4.329393945612883599, -17.49580572735151307 ) ) ;
#18146=CARTESIAN_POINT ( 'NONE',  ( 19.36978511310259421, 2.022953856625822944, -19.43459320487130171 ) ) ;
#18149=CARTESIAN_POINT ( 'NONE',  ( 19.68115760211910725, 3.144890361740488860, -20.29587546762095940 ) ) ;
#18158=CARTESIAN_POINT ( 'NONE',  ( 35.45944968151609800, -21.78403803824750185, -19.54251958818673174 ) ) ;
#18163=CARTESIAN_POINT ( 'NONE',  ( 18.55171814111300321, 6.637122934506423988, -19.73184648383247364 ) ) ;
#18164=CARTESIAN_POINT ( 'NONE',  ( 11.05541531668977662, 17.68942339022145305, -23.00000000000000711 ) ) ;
#18165=CARTESIAN_POINT ( 'NONE',  ( 35.54787733059053778, -22.18129662410796854, -18.46719521006932396 ) ) ;
#18169=CARTESIAN_POINT ( 'NONE',  ( 9.641350810849047548, 17.66889113945805789, -23.00000000000000711 ) ) ;
#18178=CARTESIAN_POINT ( 'NONE',  ( 12.86830129319110405, 9.516055860257337073, -16.11539629037995169 ) ) ;
#18179=CARTESIAN_POINT ( 'NONE',  ( 36.54816482920796972, -21.18258820310476409, -18.41547799146826847 ) ) ;
#18180=CARTESIAN_POINT ( 'NONE',  ( 17.36512755686010934, 0.5347363583120325892, -15.24149349723765390 ) ) ;
#18186=CARTESIAN_POINT ( 'NONE',  ( 28.96558774451377971, -5.053040458581501859, -15.93506438242870971 ) ) ;
#18187=CARTESIAN_POINT ( 'NONE',  ( 27.68278592340041655, -3.068913841971319112, -15.41105173719521915 ) ) ;
#18195=CARTESIAN_POINT ( 'NONE',  ( 12.29195110325218288, 8.516770644378290456, -15.29309475950548958 ) ) ;
#18200=CARTESIAN_POINT ( 'NONE',  ( 9.642214727206800617, 17.66492910891761525, -17.80644250212319690 ) ) ;
#18202=CARTESIAN_POINT ( 'NONE',  ( 14.32261721435726542, 8.042684561749755545, -14.95628083625202542 ) ) ;
#18206=CARTESIAN_POINT ( 'NONE',  ( 26.47492910780048447, -3.130564378024159211, -15.09640780237150892 ) ) ;
#18211=CARTESIAN_POINT ( 'NONE',  ( 12.24503583471362234, 9.516058715885376884, -15.33338595299508889 ) ) ;
#18213=CARTESIAN_POINT ( 'NONE',  ( 35.45944968151609800, -21.78403803824750185, -19.54251958818673174 ) ) ;
#18216=CARTESIAN_POINT ( 'NONE',  ( 23.77086030874127687, -7.150112426529108944, -14.59934731766091431 ) ) ;
#18218=CARTESIAN_POINT ( 'NONE',  ( 22.08459858401872467, -3.550466661657427636, -14.88928395763347723 ) ) ;
#18223=CARTESIAN_POINT ( 'NONE',  ( 13.98191416104776685, 5.331502061239655532, -16.22335970869868760 ) ) ;
#18224=CARTESIAN_POINT ( 'NONE',  ( 28.93285792728966044, -11.80516759558957673, -13.86517224201260134 ) ) ;
#18233=CARTESIAN_POINT ( 'NONE',  ( 21.35588827150667512, -4.635113535248831518, -19.58358080364444476 ) ) ;
#18234=CARTESIAN_POINT ( 'NONE',  ( 21.58357356133149807, 4.347441036859617469, -17.91576365920758107 ) ) ;
#18235=CARTESIAN_POINT ( 'NONE',  ( 34.08234396701924851, -12.11069646272769162, -20.88346212624082909 ) ) ;
#18237=CARTESIAN_POINT ( 'NONE',  ( 11.47310491742633687, 9.268236560789974376, -15.86081749295074594 ) ) ;
#18241=CARTESIAN_POINT ( 'NONE',  ( 9.667859621686535121, 16.22741736728331929, -17.88507964468380251 ) ) ;
#18247=CARTESIAN_POINT ( 'NONE',  ( 12.55500454421123457, 8.595009676161804890, -15.08633542003848049 ) ) ;
#18254=CARTESIAN_POINT ( 'NONE',  ( 9.090073284221231731, 16.28436349189565391, -17.07021669716791124 ) ) ;
#18255=CARTESIAN_POINT ( 'NONE',  ( 33.19064478275001306, -12.59149944747283989, -20.68751865480438212 ) ) ;
#18256=CARTESIAN_POINT ( 'NONE',  ( 19.50094987086785636, 1.087406662839465632, -19.92270839898774781 ) ) ;
#18257=CARTESIAN_POINT ( 'NONE',  ( 19.14730738223925854, 6.711798791111892371, -15.43835307388804701 ) ) ;
#18259=CARTESIAN_POINT ( 'NONE',  ( 21.36789492492977871, -4.378045371801569274, -13.15753336270543095 ) ) ;
#18270=CARTESIAN_POINT ( 'NONE',  ( 34.34130860390597206, -11.59244310827663149, -18.69197402374579653 ) ) ;
#18271=CARTESIAN_POINT ( 'NONE',  ( 10.67817636951947868, 9.002809132723193386, -16.40714615800424880 ) ) ;
#18273=CARTESIAN_POINT ( 'NONE',  ( 28.67486520862709654, -7.888541471525570614, -13.83454100519475105 ) ) ;
#18275=CARTESIAN_POINT ( 'NONE',  ( 10.36219267574928260, 16.95587413069128857, -17.77286471925143019 ) ) ;
#18286=CARTESIAN_POINT ( 'NONE',  ( 9.748920381043669536, 15.85566239202790406, -17.85155811514292878 ) ) ;
#18287=CARTESIAN_POINT ( 'NONE',  ( 24.51656338950621361, -2.114370418465405521, -18.20187689272319176 ) ) ;
#18288=CARTESIAN_POINT ( 'NONE',  ( 24.98402180921622673, -1.135180495641346266, -16.01319527449767932 ) ) ;
#18289=CARTESIAN_POINT ( 'NONE',  ( 20.51209521231993094, 3.083376493849706801, -19.38174501956431683 ) ) ;
#18294=CARTESIAN_POINT ( 'NONE',  ( 24.00918528248616468, -0.5066965781341161712, -13.81223085940890627 ) ) ;
#18304=CARTESIAN_POINT ( 'NONE',  ( 10.44197622278032611, 16.58997661396885803, -17.36392598754248695 ) ) ;
#18305=CARTESIAN_POINT ( 'NONE',  ( 35.54859390953723874, -22.18451583373416014, -15.00000000000000000 ) ) ;
#18310=CARTESIAN_POINT ( 'NONE',  ( 14.17177033308128031, 6.273687421093853800, -17.36430109743762173 ) ) ;
#18311=CARTESIAN_POINT ( 'NONE',  ( 11.24654891281740987, 16.81286035451327265, -16.80493547870787197 ) ) ;
#18315=CARTESIAN_POINT ( 'NONE',  ( 9.915973561396301150, 16.40943619918981256, -16.50475030878699556 ) ) ;
#18317=CARTESIAN_POINT ( 'NONE',  ( 12.75938622741416140, 7.627299838292535661, -14.92343961094405103 ) ) ;
#18323=CARTESIAN_POINT ( 'NONE',  ( 12.97729766242475868, 9.564223303342972216, -16.02852426037668465 ) ) ;
#18325=CARTESIAN_POINT ( 'NONE',  ( 33.40535544545146251, -10.40465400369240356, -18.27852168438239389 ) ) ;
#18326=CARTESIAN_POINT ( 'NONE',  ( 24.14158683625483803, -3.940216521628096658, -13.50644477367014673 ) ) ;
#18332=CARTESIAN_POINT ( 'NONE',  ( 22.33774198005919587, -7.088069534354142220, -17.87445411435389886 ) ) ;
#18333=CARTESIAN_POINT ( 'NONE',  ( 24.12676367385581244, 0.3224161365626431741, -13.25522683364457777 ) ) ;
#18348=CARTESIAN_POINT ( 'NONE',  ( 10.72183334705107960, 16.62641715516447150, -15.95376865854981929 ) ) ;
#18349=CARTESIAN_POINT ( 'NONE',  ( 29.49448338005720416, -10.05855281841770221, -18.88094824714235642 ) ) ;
#18352=ORIENTED_EDGE ( 'NONE', *, *, #14608, .F. ) ;
#18353=CARTESIAN_POINT ( 'NONE',  ( 9.655099948573186097, 17.60583584124798051, -17.48406748397995614 ) ) ;
#18354=CARTESIAN_POINT ( 'NONE',  ( 18.71812633715165575, 6.658065805436550910, -18.41436643113302551 ) ) ;
#18357=CARTESIAN_POINT ( 'NONE',  ( 26.72610680620850232, -7.491537437428757329, -18.63066883040512067 ) ) ;
#18361=CARTESIAN_POINT ( 'NONE',  ( 12.24557421509628519, 9.516296637964343219, -15.33295685416265286 ) ) ;
#18362=CARTESIAN_POINT ( 'NONE',  ( 33.40713826534622655, -12.56408340279653757, -19.71064172033093698 ) ) ;
#18367=CARTESIAN_POINT ( 'NONE',  ( 23.48045015178454165, 1.263488895044508897, -17.26779756161726098 ) ) ;
#18370=SURFACE_SIDE_STYLE ('',( #24968 ) ) ;
#18371=CARTESIAN_POINT ( 'NONE',  ( 15.10175627602374249, 9.741420229655037843, -13.89989488922661742 ) ) ;
#18373=CARTESIAN_POINT ( 'NONE',  ( 29.25075025305862653, -5.797754334661411768, -14.89650002867986878 ) ) ;
#18388=CARTESIAN_POINT ( 'NONE',  ( 19.07173961884560498, -1.856618079973750390, -13.92706601484911033 ) ) ;
#18389=CARTESIAN_POINT ( 'NONE',  ( 20.38603433104324480, 7.363110203939331022, -17.91596102798271062 ) ) ;
#18390=CARTESIAN_POINT ( 'NONE',  ( 34.17142927738225922, -16.99764464586957402, -20.98398627866201238 ) ) ;
#18394=CARTESIAN_POINT ( 'NONE',  ( 11.47372892693763902, 9.265404009280679531, -15.86055721330185619 ) ) ;
#18397=CARTESIAN_POINT ( 'NONE',  ( 9.992064777962580635, 14.74057119405591543, -17.75100935390776158 ) ) ;
#18402=CARTESIAN_POINT ( 'NONE',  ( 12.07641845611955489, 8.540206757827041528, -15.45582622123028216 ) ) ;
#18410=CARTESIAN_POINT ( 'NONE',  ( 9.112894736278665420, 16.17970140370183785, -17.05457397994698709 ) ) ;
#18411=CARTESIAN_POINT ( 'NONE',  ( 34.84906220094974572, -20.04189041930405324, -21.18881845514476581 ) ) ;
#18412=CARTESIAN_POINT ( 'NONE',  ( 15.35879474092683594, 2.467707791974911302, -18.63256289774529151 ) ) ;
#18413=CARTESIAN_POINT ( 'NONE',  ( 19.04375517570889187, 9.961537237715642590, -16.65452713690489617 ) ) ;
#18416=CARTESIAN_POINT ( 'NONE',  ( 23.96443177966278881, -0.8440764653970969089, -20.02211457469898548 ) ) ;
#18429=CARTESIAN_POINT ( 'NONE',  ( 35.36378496564391583, -20.35426714484339783, -19.25178739305277631 ) ) ;
#18430=CARTESIAN_POINT ( 'NONE',  ( 10.66893569228806271, 9.043500038842159583, -16.41109624600252559 ) ) ;
#18435=CARTESIAN_POINT ( 'NONE',  ( 11.70392491148546732, 10.80251906652491556, -16.82536866641744311 ) ) ;
#18442=ORIENTED_EDGE ( 'NONE', *, *, #15818, .T. ) ;
#18443=ORIENTED_EDGE ( 'NONE', *, *, #2983, .T. ) ;
#18447=CARTESIAN_POINT ( 'NONE',  ( 9.667875940510226584, 16.22734252707768832, -17.88507284477129033 ) ) ;
#18449=CARTESIAN_POINT ( 'NONE',  ( 22.36047763332208405, -4.488847068091893711, -15.41575731358746104 ) ) ;
#18450=CARTESIAN_POINT ( 'NONE',  ( 20.06573045921589227, -2.681363122285017386, -18.07621394912722934 ) ) ;
#18451=CARTESIAN_POINT ( 'NONE',  ( 22.61876936045522513, 2.364863857962155258, -15.74433402521326819 ) ) ;
#18455=CARTESIAN_POINT ( 'NONE',  ( 26.84970692451943819, -5.812874930055231815, -14.04107299160273037 ) ) ;
#18461=CARTESIAN_POINT ( 'NONE',  ( 10.37265302513970688, 16.90790163500151166, -17.63730412279738147 ) ) ;
#18468=CARTESIAN_POINT ( 'NONE',  ( 15.94478687392618355, 4.193953704849600506, -19.05305658475056063 ) ) ;
#18469=CARTESIAN_POINT ( 'NONE',  ( 11.27553273857261296, 16.67993683502164615, -16.78480078315762469 ) ) ;
#18473=CARTESIAN_POINT ( 'NONE',  ( 9.641350777746193756, 17.66889129127197577, -17.91630266473768884 ) ) ;
#18474=CARTESIAN_POINT ( 'NONE',  ( 12.97376706329020557, 7.722038565090276308, -14.75257430067278719 ) ) ;
#18480=CARTESIAN_POINT ( 'NONE',  ( 10.63408956504272140, 15.70892033759881734, -17.26778321585235787 ) ) ;
#18483=CARTESIAN_POINT ( 'NONE',  ( 36.54859390953724585, -21.18451583373416014, -16.11276402859391510 ) ) ;
#18484=CARTESIAN_POINT ( 'NONE',  ( 24.87127057246125972, -9.548149280147088191, -14.79180087847266556 ) ) ;
#18491=CLOSED_SHELL ( 'NONE', ( #3448, #14777, #7502, #4574, #6823, #28735, #3986, #16173 ) ) ;
#18492=CARTESIAN_POINT ( 'NONE',  ( 16.98323446405135329, 7.186294067752427850, -20.40390978395066313 ) ) ;
#18493=CARTESIAN_POINT ( 'NONE',  ( 27.14379157474815685, -3.097389544916523185, -14.25532379610351263 ) ) ;
#18501=CARTESIAN_POINT ( 'NONE',  ( 10.33811696370167077, 18.38618940166710303, -17.91541423781815112 ) ) ;
#18507=CARTESIAN_POINT ( 'NONE',  ( 11.47219014545126647, 9.272428573238919114, -15.86119603109536058 ) ) ;
#18509=CARTESIAN_POINT ( 'NONE',  ( 18.42634509371275797, 7.189141296957872740, -15.94500943014882210 ) ) ;
#18512=CARTESIAN_POINT ( 'NONE',  ( 27.21278356834291756, -7.014839303453253905, -18.45691071023835761 ) ) ;
#18516=CARTESIAN_POINT ( 'NONE',  ( 11.13911793526871463, 17.30555251181618814, -17.04533519337964975 ) ) ;
#18519=CARTESIAN_POINT ( 'NONE',  ( 35.03938282813840743, -19.89690018161999419, -20.20402626681843117 ) ) ;
#18524=CARTESIAN_POINT ( 'NONE',  ( 22.08234585817149664, -3.071498426668943793, -18.09723855971599704 ) ) ;
#18530=CARTESIAN_POINT ( 'NONE',  ( 22.83681518364245022, 2.349634567491368564, -16.30468554850739338 ) ) ;
#18531=CARTESIAN_POINT ( 'NONE',  ( 29.08439603799166306, -5.802884797086306001, -14.52222230071497755 ) ) ;
#18539=CARTESIAN_POINT ( 'NONE',  ( 9.641352920869014298, 17.66888146263751125, -17.91030124961049097 ) ) ;
#18540=CARTESIAN_POINT ( 'NONE',  ( 27.14379157474815685, -3.097389544916523185, -14.25532379610351263 ) ) ;
#18541=CARTESIAN_POINT ( 'NONE',  ( 19.54218497767158169, 4.227554098413554229, -14.22708607227295730 ) ) ;
#18542=CARTESIAN_POINT ( 'NONE',  ( 36.54859390953724585, -23.18451583373416014, -17.78191007148576119 ) ) ;
#18548=CARTESIAN_POINT ( 'NONE',  ( 15.94478687392618355, 4.193953704849600506, -19.05305658475056063 ) ) ;
#18551=CARTESIAN_POINT ( 'NONE',  ( 12.60945047077962933, 8.619070305187777947, -15.04294105552940231 ) ) ;
#18556=CARTESIAN_POINT ( 'NONE',  ( 14.79111372287554715, 6.954724682967856175, -19.27298399620107361 ) ) ;
#18562=CARTESIAN_POINT ( 'NONE',  ( 35.54859390953724585, -23.18451583373416014, -18.06010107863414405 ) ) ;
#18564=CARTESIAN_POINT ( 'NONE',  ( 23.81787570424677014, -0.6874775570582684070, -15.56398403670522157 ) ) ;
#18566=CARTESIAN_POINT ( 'NONE',  ( 18.51435942584036454, 8.743714487506315081, -19.56092670885941587 ) ) ;
#18569=CARTESIAN_POINT ( 'NONE',  ( 25.07021298685211619, 1.093672866225363638, -16.25732641482299812 ) ) ;
#18577=CARTESIAN_POINT ( 'NONE',  ( 13.39606018151479461, 8.691252192278360766, -15.69476314099692971 ) ) ;
#18579=CARTESIAN_POINT ( 'NONE',  ( 36.21506517127201619, -19.68614788779310132, -19.44682451121369482 ) ) ;
#18580=AXIS2_PLACEMENT_3D ( 'NONE', #22851, #29474, #11379 ) ;
#18581=CARTESIAN_POINT ( 'NONE',  ( 10.66768918063838179, 9.049215891674000645, -16.41161178408055932 ) ) ;
#18584=CARTESIAN_POINT ( 'NONE',  ( 10.47193650065820592, 16.45257496057443802, -17.33483926051624735 ) ) ;
#18597=CARTESIAN_POINT ( 'NONE',  ( 9.661958148507006072, 16.25448227554711167, -17.91102859374088752 ) ) ;
#18598=CARTESIAN_POINT ( 'NONE',  ( 24.16216977846044145, 1.369666316211566093, -18.31128106405367006 ) ) ;
#18599=CARTESIAN_POINT ( 'NONE',  ( 20.53830075755067952, -2.223150928429542095, -18.95983797452030828 ) ) ;
#18601=CARTESIAN_POINT ( 'NONE',  ( 22.28231863826031756, 1.183864898644814811, -18.90614694914491167 ) ) ;
#18604=CARTESIAN_POINT ( 'NONE',  ( 10.00000000000007816, 17.32050807568872486, -23.00000000000000711 ) ) ;
#18605=CARTESIAN_POINT ( 'NONE',  ( 22.34083945069921739, -4.755659482961629436, -14.12236044035638116 ) ) ;
#18616=CARTESIAN_POINT ( 'NONE',  ( 33.43446274600908907, -12.68684440242773448, -19.71889742777951327 ) ) ;
#18618=CARTESIAN_POINT ( 'NONE',  ( 13.27290874800832121, 7.583804977141803683, -15.79253525446438999 ) ) ;
#18622=CARTESIAN_POINT ( 'NONE',  ( 21.04385110482095200, 5.766204710259658306, -15.30406332615466347 ) ) ;
#18623=CARTESIAN_POINT ( 'NONE',  ( 11.27582353004791216, 16.67860322824865449, -16.78467813988110890 ) ) ;
#18624=CARTESIAN_POINT ( 'NONE',  ( 34.82539348385352440, -18.93555941106099993, -20.13934242161363741 ) ) ;
#18628=CARTESIAN_POINT ( 'NONE',  ( 9.898178882064430084, 16.49104486689975246, -16.51464960819000893 ) ) ;
#18630=CARTESIAN_POINT ( 'NONE',  ( 13.19155076956097083, 7.818281081198240834, -14.57899684263624351 ) ) ;
#18638=CARTESIAN_POINT ( 'NONE',  ( 10.44197622278032611, 16.58997661396885803, -17.36392598754248695 ) ) ;
#18640=CARTESIAN_POINT ( 'NONE',  ( 31.25429145842602452, -9.414624517878500853, -14.20845315089566441 ) ) ;
#18641=CARTESIAN_POINT ( 'NONE',  ( 26.92971693216691165, -8.617903733377630715, -13.36642543767191427 ) ) ;
#18647=CARTESIAN_POINT ( 'NONE',  ( 18.93384218461971358, 6.651393094135895190, -15.21227712214292538 ) ) ;
#18648=CARTESIAN_POINT ( 'NONE',  ( 28.13717792526295014, -10.23527491042630011, -17.83415580063453376 ) ) ;
#18654=DIRECTION ( 'NONE',  ( 1.665334536937734318E-16, -2.498001805406601723E-16, -1.000000000000000000 ) ) ;
#18659=CARTESIAN_POINT ( 'NONE',  ( 10.33811987107833552, 18.38617606806709048, -17.90816805339326834 ) ) ;
#18663=CARTESIAN_POINT ( 'NONE',  ( 10.24089172292967298, 14.91932009296530559, -16.37038124228770997 ) ) ;
#18666=CARTESIAN_POINT ( 'NONE',  ( 18.17852402710872894, 9.427450501112501158, -16.79750701094832266 ) ) ;
#18669=CARTESIAN_POINT ( 'NONE',  ( 27.78884322698630882, -6.380937659459246625, -17.89340433249687834 ) ) ;
#18672=CARTESIAN_POINT ( 'NONE',  ( 11.09873500484433606, 17.49075377836879497, -17.25232203421226274 ) ) ;
#18673=CARTESIAN_POINT ( 'NONE',  ( 35.53758243340352863, -21.13504710440451007, -18.64505253599016044 ) ) ;
#18676=CARTESIAN_POINT ( 'NONE',  ( 28.44965076230254653, -4.228683950944192027, -16.16799691904953562 ) ) ;
#18680=CARTESIAN_POINT ( 'NONE',  ( 18.53947781130984751, 1.256531364521723537, -18.82393729036428098 ) ) ;
#18681=CARTESIAN_POINT ( 'NONE',  ( 17.24934648279766947, 4.534969372434432877, -15.14864769235989073 ) ) ;
#18695=CARTESIAN_POINT ( 'NONE',  ( 9.641350944112486943, 17.66889052829492002, -17.91441860517739215 ) ) ;
#18696=CARTESIAN_POINT ( 'NONE',  ( 27.68339325353806046, -3.782361434017075474, -17.87574284786517964 ) ) ;
#18697=CARTESIAN_POINT ( 'NONE',  ( 22.61876936045522513, 2.364863857962155258, -15.74433402521326819 ) ) ;
#18698=CARTESIAN_POINT ( 'NONE',  ( 31.68531546575670532, -10.25520638109567173, -17.65856934995331784 ) ) ;
#18700=CARTESIAN_POINT ( 'NONE',  ( 16.84948243412402036, 10.49281628697410262, -11.66356073909478575 ) ) ;
#18703=CARTESIAN_POINT ( 'NONE',  ( 15.73644607668725826, 9.740111719757674535, -14.94734896276200153 ) ) ;
#18706=CARTESIAN_POINT ( 'NONE',  ( 10.72107673987424015, 16.62988705212242735, -15.95408154060974404 ) ) ;
#18711=CARTESIAN_POINT ( 'NONE',  ( 15.78240017141095741, 4.038647184180326200, -18.77507866864583619 ) ) ;
#18713=CARTESIAN_POINT ( 'NONE',  ( 12.89848499713582441, 9.804829593628518580, -14.81257543621576112 ) ) ;
#18715=CARTESIAN_POINT ( 'NONE',  ( 33.20847722810714231, -12.67161117835268058, -20.69290897523819694 ) ) ;
#18716=CARTESIAN_POINT ( 'NONE',  ( 25.50636554463319072, -2.203555497659483553, -15.54816553724606187 ) ) ;
#18717=CARTESIAN_POINT ( 'NONE',  ( 15.96850636225579656, 5.405031054132949819, -14.95518105802344344 ) ) ;
#18718=CARTESIAN_POINT ( 'NONE',  ( 25.07031029108804887, -10.85539403410516535, -16.40584363908930499 ) ) ;
#18730=CARTESIAN_POINT ( 'NONE',  ( 36.54859390953724585, -21.18451583373416014, -18.06010107863414405 ) ) ;
#18731=CARTESIAN_POINT ( 'NONE',  ( 12.78320632028979809, 7.637826363492710158, -14.90445457646871574 ) ) ;
#18736=CARTESIAN_POINT ( 'NONE',  ( 10.47195275365909595, 16.45250042224058618, -17.33483252618548676 ) ) ;
#18744=CARTESIAN_POINT ( 'NONE',  ( 9.661887760751893595, 16.25480508276471525, -17.91458275280492884 ) ) ;
#18745=CARTESIAN_POINT ( 'NONE',  ( 26.88076058338416274, -6.009164776401831887, -18.61148891559023255 ) ) ;
#18747=CARTESIAN_POINT ( 'NONE',  ( 18.53947781130984751, 1.256531364521723537, -18.82393729036428098 ) ) ;
#18752=CARTESIAN_POINT ( 'NONE',  ( 27.21278356834291756, -7.014839303453253905, -18.45691071023835761 ) ) ;
#18760=CARTESIAN_POINT ( 'NONE',  ( 10.46722255365007115, 16.47419372244215197, -17.33720764016775462 ) ) ;
#18761=CARTESIAN_POINT ( 'NONE',  ( 35.37764311538968087, -21.41652447078215005, -19.89511094362359955 ) ) ;
#18762=CARTESIAN_POINT ( 'NONE',  ( 31.15806985163746390, -10.82494328065958911, -14.16671120874331358 ) ) ;
#18764=CARTESIAN_POINT ( 'NONE',  ( 8.944592922245861999, 16.95155497634765851, -17.90742740301624991 ) ) ;
#18768=CARTESIAN_POINT ( 'NONE',  ( 19.07848178107829540, -2.338951347401693859, -17.85627120065723616 ) ) ;
#18769=CARTESIAN_POINT ( 'NONE',  ( 11.27146506517978786, 16.69859170370891377, -16.78668372539920739 ) ) ;
#18773=CARTESIAN_POINT ( 'NONE',  ( 9.641384570184822422, 17.66873631484086715, -17.89388817125738385 ) ) ;
#18775=CARTESIAN_POINT ( 'NONE',  ( 10.82443827553465177, 12.24310121783546634, -16.12906421532448675 ) ) ;
#18778=ORIENTED_EDGE ( 'NONE', *, *, #26748, .T. ) ;
#18782=CARTESIAN_POINT ( 'NONE',  ( 10.47184394332236224, 16.45299944031493311, -17.33487789703667303 ) ) ;
#18784=CARTESIAN_POINT ( 'NONE',  ( 36.54859390953724585, -22.18451583373416014, -17.22552805718784441 ) ) ;
#18785=CARTESIAN_POINT ( 'NONE',  ( 26.07968421886551980, -9.001936657367064498, -13.61655714643126913 ) ) ;
#18786=CARTESIAN_POINT ( 'NONE',  ( 26.47492910780048447, -3.130564378024159211, -15.09640780237150892 ) ) ;
#18790=CARTESIAN_POINT ( 'NONE',  ( 33.24108837279852224, -10.36619216719171632, -17.82210672427467912 ) ) ;
#18791=CARTESIAN_POINT ( 'NONE',  ( 15.40919527484693319, 5.754234090002595003, -19.70842740302703078 ) ) ;
#18792=CARTESIAN_POINT ( 'NONE',  ( 27.11308663627701776, -11.54974243744149653, -14.54931088138702933 ) ) ;
#18798=DIRECTION ( 'NONE',  ( -0.7172983783020616677, 0.6967661275386687336, 0.000000000000000000 ) ) ;
#18802=CARTESIAN_POINT ( 'NONE',  ( 10.41323547201801958, 18.04168634714536168, -16.76531574090561350 ) ) ;
#18807=CARTESIAN_POINT ( 'NONE',  ( 11.40798482813988635, 9.566882342703072695, -15.88774718835883348 ) ) ;
#18810=CARTESIAN_POINT ( 'NONE',  ( 17.24934648279766947, 4.534969372434432877, -15.14864769235989073 ) ) ;
#18813=CARTESIAN_POINT ( 'NONE',  ( 25.26806593431409453, -8.821542497490490575, -18.05414547114721557 ) ) ;
#18815=CARTESIAN_POINT ( 'NONE',  ( 11.06231504941914423, 17.65778033641372957, -17.63750823492871334 ) ) ;
#18817=CARTESIAN_POINT ( 'NONE',  ( 35.30103323675335503, -20.07235686745416103, -19.24079536022738068 ) ) ;
#18820=CARTESIAN_POINT ( 'NONE',  ( 24.09482019364002880, -4.431952660107454811, -19.05667854325333721 ) ) ;
#18825=CARTESIAN_POINT ( 'NONE',  ( 17.20140313730510684, 4.016069822000726042, -19.84498366692964666 ) ) ;
#18826=CARTESIAN_POINT ( 'NONE',  ( 17.26923406770577074, 6.766716122889627094, -15.27140832040383422 ) ) ;
#18837=CARTESIAN_POINT ( 'NONE',  ( 9.893572868141015775, 16.51216863388285461, -16.51808063826580408 ) ) ;
#18838=CARTESIAN_POINT ( 'NONE',  ( 21.64995824428719828, -4.359751022247916552, -19.89060884261010287 ) ) ;
#18839=CARTESIAN_POINT ( 'NONE',  ( 20.53420570626898822, -0.4664991210283321310, -19.04361528682417415 ) ) ;
#18840=CARTESIAN_POINT ( 'NONE',  ( 33.19064478275001306, -12.59149944747283989, -20.68751865480438212 ) ) ;
#18847=CARTESIAN_POINT ( 'NONE',  ( 14.29829396236512729, 6.476847147513518088, -18.28004444394726491 ) ) ;
#18850=CARTESIAN_POINT ( 'NONE',  ( 10.72132679622416696, 16.62874026182691267, -15.95397813513572061 ) ) ;
#18856=CARTESIAN_POINT ( 'NONE',  ( 19.51440197245297270, 8.071880087464508691, -17.28625796899888201 ) ) ;
#18858=CARTESIAN_POINT ( 'NONE',  ( 27.55585723563325473, -10.26521964199731407, -19.78748283923107820 ) ) ;
#18860=CARTESIAN_POINT ( 'NONE',  ( 35.09535884372434111, -21.14837076832613860, -21.10414782775458420 ) ) ;
#18864=CARTESIAN_POINT ( 'NONE',  ( 20.68883037063079300, -1.960602941680898548, -15.52464631352181001 ) ) ;
#18866=CARTESIAN_POINT ( 'NONE',  ( 17.00902653454025071, 3.367308883600929281, -16.20218648120260951 ) ) ;
#18867=CARTESIAN_POINT ( 'NONE',  ( 30.22932097093386261, -9.048247045011217793, -15.48080783641366942 ) ) ;
#18875=CARTESIAN_POINT ( 'NONE',  ( 36.31991209326969283, -20.15716956937155047, -19.46864736847591359 ) ) ;
#18876=( BOUNDED_SURFACE ( )  B_SPLINE_SURFACE ( 3, 3, ( 
 ( #20058, #24344, #29114, #1306, #17312, #3442, #29432, #22513, #10595, #12733, #14862, #1157, #26968, #6028, #24644, #3739, #10751, #1613, #8453, #5579, #24201, #3304, #10291, #28969, #21898, #9194, #13779, #4633, #1758, #18362, #6330, #8746, #27720, #6481, #13479, #22961, #11343, #11484, #27426, #13334, #15918, #22657, #30032, #20798, #15770, #30184, #27569, #4488, #18519, #25540, #11047, #20349, #6625, #4335, #25095, #25248, #27877, #6932, #6780, #18213, #11640, #16226, #13631, #29740, #18065, #16070, #2062, #20645, #4185, #9040, #22811, #1915, #9347, #25398, #13923, #11193, #23107, #23255 ),
 ( #20503, #29889, #2210, #2368, #20951, #8897, #63, #27280, #15625, #24959, #4039, #7233, #21564, #18973, #26159, #9948, #16982, #4785, #11790, #28332, #26005, #16532, #16682, #12246, #663, #28475, #9654, #3120, #19261, #7387, #21109, #2521, #19119, #5084, #2812, #215, #14372, #14075, #23404, #809, #23710, #26308, #25855, #12096, #7674, #24020, #21412, #517, #25693, #18817, #5390, #4934, #5233, #9807, #9493, #14225, #12392, #28175, #21704, #7523, #14677, #18673, #28018, #16827, #28619, #14527, #23557, #7077, #16374, #2658, #23869, #11934, #2969, #21256, #367, #5987, #10251, #15127 ),
 ( #19564, #10101, #17720, #969, #10554, #24457, #1124, #19863, #26771, #5693, #24764, #8263, #3853, #3553, #24607, #28932, #14972, #24308, #12540, #21859, #3699, #27079, #3404, #7968, #19414, #26612, #12695, #12845, #17276, #22157, #1267, #29389, #29227, #17573, #22016, #10402, #5540, #14825, #19709, #22312, #26928, #6138, #24160, #15275, #29075, #17422, #8117, #5841, #13000, #1421, #10710, #20020, #13150, #8415, #15434, #22474, #3265, #28783, #7826, #17133, #26460, #8861, #27239, #6289, #13889, #18179, #9154, #29698, #1880, #20759, #6902, #29855, #6591, #8563, #1720, #18483, #8712, #9005 ),
 ( #16192, #11005, #18027, #13446, #2030, #22929, #15735, #15881, #15585, #27839, #17863, #6743, #20309, #27393, #27537, #18325, #1572, #4455, #6446, #25062, #23075, #2174, #11450, #10851, #4149, #30147, #25360, #25214, #13601, #13747, #22774, #25510, #4601, #24920, #20162, #11161, #29544, #22619, #20466, #4302, #11309, #16035, #4001, #27683, #20612, #30000, #13300, #23367, #27986, #5199, #181, #25815, #28292, #19085, #23518, #23672, #20914, #2627, #9768, #12208, #25655, #7346, #4747, #14493, #7046, #21527, #9315, #16337, #18936, #23830, #9460, #28437, #28, #18784, #2776, #16646, #629, #14038 ),
 ( #18640, #25964, #7489, #11757, #26121, #11902, #479, #2928, #9914, #2483, #21074, #28138, #21218, #333, #7195, #9618, #16794, #19225, #12058, #14191, #7636, #28582, #5045, #16489, #4896, #21371, #14336, #16943, #26272, #5354, #23216, #2331, #11600, #22401, #22701, #12502, #15355, #4084, #20391, #13078, #20101, #21666, #14786, #1808, #21825, #22557, #6220, #17096, #10217, #29782, #10065, #8790, #17798, #11090, #18107, #27469, #15513, #25001, #24694, #5501, #23987, #3084, #12353, #20244, #14640, #29631, #24847, #768, #10933, #24126, #29479, #3781, #19377, #6069, #3224, #28741, #7787, #925 ),
 ( #13377, #26421, #19948, #17651, #29315, #8349, #1504, #10794, #27013, #8643, #15668, #17946, #3933, #8499, #6377, #27160, #13236, #27321, #1655, #9086, #11527, #2406, #6828, #6974, #4229, #16116, #23294, #25740, #8939, #20839, #18255, #18715, #11239, #4822, #22855, #20543, #2254, #28063, #13679, #11682, #13530, #23005, #16261, #30220, #14120, #29932, #23449, #1957, #6523, #18411, #25437, #107, #27610, #9389, #20996, #7116, #18860, #16420, #25573, #15813, #2561, #4672, #6673, #11835, #27761, #15962, #25292, #21147, #9232, #18562, #4528, #25138, #27915, #13964, #13816, #258, #9536, #4381 ),
 ( #2107, #11384, #23144, #20688, #30074, #407, #12288, #564, #19458, #5280, #2853, #21300, #14567, #25898, #9692, #17027, #16575, #12139, #3310, #7427, #14416, #9849, #28669, #19307, #21456, #21608, #11980, #5586, #4975, #3162, #16727, #26048, #23917, #5432, #10297, #856, #5126, #19162, #28828, #7865, #17175, #7272, #23756, #26504, #21753, #3011, #9991, #10146, #28519, #12586, #14867, #14266, #21905, #7567, #24207, #19018, #16873, #706, #26202, #12434, #1020, #24062, #7718, #26353, #28222, #28372, #2697, #23601, #14719, #22201, #24651, #15478, #19912, #20064, #17319, #29276, #6183, #8607 ) ),
 .UNSPECIFIED., .T., .F., .F. ) 
 B_SPLINE_SURFACE_WITH_KNOTS ( ( 4, 3, 4 ),
 ( 4, 2, 2, 2, 2, 2, 2, 2, 2, 2, 2, 2, 2, 2, 2, 2, 2, 2, 2, 2, 2, 2, 2, 2, 2, 2, 2, 2, 2, 2, 2, 2, 2, 2, 2, 2, 2, 2, 4 ),
 ( 0.000000000000000000, 0.5000000000000000000, 1.000000000000000000 ),
 ( 0.000000000000000000, 0.1003381136405422785, 0.1505071704608134109, 0.1755916988709489979, 0.1881339630760167636, 0.1944050951785506465, 0.2006762272810845571, 0.2086934065084689038, 0.2167105857358532783, 0.2327449441906219718, 0.2648136611001593588, 0.2968823780096967457, 0.3129167364644654947, 0.3209339156918498137, 0.3289510949192341882, 0.3346579968240730452, 0.3403648987289118466, 0.3517787025385894495, 0.3746063101579446553, 0.4202615253966550668, 0.5115719558740758899, 0.6028823863514967130, 0.6485376015902071245, 0.6713652092095623303, 0.6827790130192399332, 0.6941928168289175360, 0.7036545619149295883, 0.7131163070009416405, 0.7320397971729657449, 0.7698867775170139538, 0.8077337578610621627, 0.8266572480330862671, 0.8361189931190984304, 0.8455807382051104826, 0.8552319420672911399, 0.8648831459294716861, 0.8841855536538327787, 0.9227903691025551858, 1.000000000000000000 ),
 .UNSPECIFIED. ) 
 GEOMETRIC_REPRESENTATION_ITEM ( )  RATIONAL_B_SPLINE_SURFACE ( (
 ( 1.000000000000000000, 1.000000000000000000, 1.000000000000000000, 1.000000000000000000, 1.000000000000000000, 1.000000000000000000, 1.000000000000000000, 1.000000000000000000, 1.000000000000000000, 1.000000000000000000, 1.000000000000000000, 1.000000000000000000, 1.000000000000000000, 1.000000000000000000, 1.000000000000000000, 1.000000000000000000, 1.000000000000000000, 1.000000000000000000, 1.000000000000000000, 1.000000000000000000, 1.000000000000000000, 1.000000000000000000, 1.000000000000000000, 1.000000000000000000, 1.000000000000000000, 1.000000000000000000, 1.000000000000000000, 1.000000000000000000, 1.000000000000000000, 1.000000000000000000, 1.000000000000000000, 1.000000000000000000, 1.000000000000000000, 1.000000000000000000, 1.000000000000000000, 1.000000000000000000, 1.000000000000000000, 1.000000000000000000, 1.000000000000000000, 1.000000000000000000, 1.000000000000000000, 1.000000000000000000, 1.000000000000000000, 1.000000000000000000, 1.000000000000000000, 1.000000000000000000, 1.000000000000000000, 1.000000000000000000, 1.000000000000000000, 1.000000000000000000, 1.000000000000000000, 1.000000000000000000, 1.000000000000000000, 1.000000000000000000, 1.000000000000000000, 1.000000000000000000, 1.000000000000000000, 1.000000000000000000, 1.000000000000000000, 1.000000000000000000, 1.000000000000000000, 1.000000000000000000, 1.000000000000000000, 1.000000000000000000, 1.000000000000000000, 1.000000000000000000, 1.000000000000000000, 1.000000000000000000, 1.000000000000000000, 1.000000000000000000, 1.000000000000000000, 1.000000000000000000, 1.000000000000000000, 1.000000000000000000, 1.000000000000000000, 1.000000000000000000, 1.000000000000000000, 1.000000000000000000),
 ( 0.3333333333333333703, 0.3333333333333333703, 0.3333333333333333703, 0.3333333333333333703, 0.3333333333333333703, 0.3333333333333333703, 0.3333333333333333703, 0.3333333333333333703, 0.3333333333333333703, 0.3333333333333333703, 0.3333333333333333703, 0.3333333333333333703, 0.3333333333333333703, 0.3333333333333333703, 0.3333333333333333703, 0.3333333333333333703, 0.3333333333333333703, 0.3333333333333333703, 0.3333333333333333703, 0.3333333333333333703, 0.3333333333333333703, 0.3333333333333333703, 0.3333333333333333703, 0.3333333333333333703, 0.3333333333333333703, 0.3333333333333333703, 0.3333333333333333703, 0.3333333333333333703, 0.3333333333333333703, 0.3333333333333333703, 0.3333333333333333703, 0.3333333333333333703, 0.3333333333333333703, 0.3333333333333333703, 0.3333333333333333703, 0.3333333333333333703, 0.3333333333333333703, 0.3333333333333333703, 0.3333333333333333703, 0.3333333333333333703, 0.3333333333333333703, 0.3333333333333333703, 0.3333333333333333703, 0.3333333333333333703, 0.3333333333333333703, 0.3333333333333333703, 0.3333333333333333703, 0.3333333333333333703, 0.3333333333333333703, 0.3333333333333333703, 0.3333333333333333703, 0.3333333333333333703, 0.3333333333333333703, 0.3333333333333333703, 0.3333333333333333703, 0.3333333333333333703, 0.3333333333333333703, 0.3333333333333333703, 0.3333333333333333703, 0.3333333333333333703, 0.3333333333333333703, 0.3333333333333333703, 0.3333333333333333703, 0.3333333333333333703, 0.3333333333333333703, 0.3333333333333333703, 0.3333333333333333703, 0.3333333333333333703, 0.3333333333333333703, 0.3333333333333333703, 0.3333333333333333703, 0.3333333333333333703, 0.3333333333333333703, 0.3333333333333333703, 0.3333333333333333703, 0.3333333333333333703, 0.3333333333333333703, 0.3333333333333333703),
 ( 0.3333333333333333703, 0.3333333333333333703, 0.3333333333333333703, 0.3333333333333333703, 0.3333333333333333703, 0.3333333333333333703, 0.3333333333333333703, 0.3333333333333333703, 0.3333333333333333703, 0.3333333333333333703, 0.3333333333333333703, 0.3333333333333333703, 0.3333333333333333703, 0.3333333333333333703, 0.3333333333333333703, 0.3333333333333333703, 0.3333333333333333703, 0.3333333333333333703, 0.3333333333333333703, 0.3333333333333333703, 0.3333333333333333703, 0.3333333333333333703, 0.3333333333333333703, 0.3333333333333333703, 0.3333333333333333703, 0.3333333333333333703, 0.3333333333333333703, 0.3333333333333333703, 0.3333333333333333703, 0.3333333333333333703, 0.3333333333333333703, 0.3333333333333333703, 0.3333333333333333703, 0.3333333333333333703, 0.3333333333333333703, 0.3333333333333333703, 0.3333333333333333703, 0.3333333333333333703, 0.3333333333333333703, 0.3333333333333333703, 0.3333333333333333703, 0.3333333333333333703, 0.3333333333333333703, 0.3333333333333333703, 0.3333333333333333703, 0.3333333333333333703, 0.3333333333333333703, 0.3333333333333333703, 0.3333333333333333703, 0.3333333333333333703, 0.3333333333333333703, 0.3333333333333333703, 0.3333333333333333703, 0.3333333333333333703, 0.3333333333333333703, 0.3333333333333333703, 0.3333333333333333703, 0.3333333333333333703, 0.3333333333333333703, 0.3333333333333333703, 0.3333333333333333703, 0.3333333333333333703, 0.3333333333333333703, 0.3333333333333333703, 0.3333333333333333703, 0.3333333333333333703, 0.3333333333333333703, 0.3333333333333333703, 0.3333333333333333703, 0.3333333333333333703, 0.3333333333333333703, 0.3333333333333333703, 0.3333333333333333703, 0.3333333333333333703, 0.3333333333333333703, 0.3333333333333333703, 0.3333333333333333703, 0.3333333333333333703),
 ( 1.000000000000000000, 1.000000000000000000, 1.000000000000000000, 1.000000000000000000, 1.000000000000000000, 1.000000000000000000, 1.000000000000000000, 1.000000000000000000, 1.000000000000000000, 1.000000000000000000, 1.000000000000000000, 1.000000000000000000, 1.000000000000000000, 1.000000000000000000, 1.000000000000000000, 1.000000000000000000, 1.000000000000000000, 1.000000000000000000, 1.000000000000000000, 1.000000000000000000, 1.000000000000000000, 1.000000000000000000, 1.000000000000000000, 1.000000000000000000, 1.000000000000000000, 1.000000000000000000, 1.000000000000000000, 1.000000000000000000, 1.000000000000000000, 1.000000000000000000, 1.000000000000000000, 1.000000000000000000, 1.000000000000000000, 1.000000000000000000, 1.000000000000000000, 1.000000000000000000, 1.000000000000000000, 1.000000000000000000, 1.000000000000000000, 1.000000000000000000, 1.000000000000000000, 1.000000000000000000, 1.000000000000000000, 1.000000000000000000, 1.000000000000000000, 1.000000000000000000, 1.000000000000000000, 1.000000000000000000, 1.000000000000000000, 1.000000000000000000, 1.000000000000000000, 1.000000000000000000, 1.000000000000000000, 1.000000000000000000, 1.000000000000000000, 1.000000000000000000, 1.000000000000000000, 1.000000000000000000, 1.000000000000000000, 1.000000000000000000, 1.000000000000000000, 1.000000000000000000, 1.000000000000000000, 1.000000000000000000, 1.000000000000000000, 1.000000000000000000, 1.000000000000000000, 1.000000000000000000, 1.000000000000000000, 1.000000000000000000, 1.000000000000000000, 1.000000000000000000, 1.000000000000000000, 1.000000000000000000, 1.000000000000000000, 1.000000000000000000, 1.000000000000000000, 1.000000000000000000),
 ( 0.3333333333333333703, 0.3333333333333333703, 0.3333333333333333703, 0.3333333333333333703, 0.3333333333333333703, 0.3333333333333333703, 0.3333333333333333703, 0.3333333333333333703, 0.3333333333333333703, 0.3333333333333333703, 0.3333333333333333703, 0.3333333333333333703, 0.3333333333333333703, 0.3333333333333333703, 0.3333333333333333703, 0.3333333333333333703, 0.3333333333333333703, 0.3333333333333333703, 0.3333333333333333703, 0.3333333333333333703, 0.3333333333333333703, 0.3333333333333333703, 0.3333333333333333703, 0.3333333333333333703, 0.3333333333333333703, 0.3333333333333333703, 0.3333333333333333703, 0.3333333333333333703, 0.3333333333333333703, 0.3333333333333333703, 0.3333333333333333703, 0.3333333333333333703, 0.3333333333333333703, 0.3333333333333333703, 0.3333333333333333703, 0.3333333333333333703, 0.3333333333333333703, 0.3333333333333333703, 0.3333333333333333703, 0.3333333333333333703, 0.3333333333333333703, 0.3333333333333333703, 0.3333333333333333703, 0.3333333333333333703, 0.3333333333333333703, 0.3333333333333333703, 0.3333333333333333703, 0.3333333333333333703, 0.3333333333333333703, 0.3333333333333333703, 0.3333333333333333703, 0.3333333333333333703, 0.3333333333333333703, 0.3333333333333333703, 0.3333333333333333703, 0.3333333333333333703, 0.3333333333333333703, 0.3333333333333333703, 0.3333333333333333703, 0.3333333333333333703, 0.3333333333333333703, 0.3333333333333333703, 0.3333333333333333703, 0.3333333333333333703, 0.3333333333333333703, 0.3333333333333333703, 0.3333333333333333703, 0.3333333333333333703, 0.3333333333333333703, 0.3333333333333333703, 0.3333333333333333703, 0.3333333333333333703, 0.3333333333333333703, 0.3333333333333333703, 0.3333333333333333703, 0.3333333333333333703, 0.3333333333333333703, 0.3333333333333333703),
 ( 0.3333333333333333703, 0.3333333333333333703, 0.3333333333333333703, 0.3333333333333333703, 0.3333333333333333703, 0.3333333333333333703, 0.3333333333333333703, 0.3333333333333333703, 0.3333333333333333703, 0.3333333333333333703, 0.3333333333333333703, 0.3333333333333333703, 0.3333333333333333703, 0.3333333333333333703, 0.3333333333333333703, 0.3333333333333333703, 0.3333333333333333703, 0.3333333333333333703, 0.3333333333333333703, 0.3333333333333333703, 0.3333333333333333703, 0.3333333333333333703, 0.3333333333333333703, 0.3333333333333333703, 0.3333333333333333703, 0.3333333333333333703, 0.3333333333333333703, 0.3333333333333333703, 0.3333333333333333703, 0.3333333333333333703, 0.3333333333333333703, 0.3333333333333333703, 0.3333333333333333703, 0.3333333333333333703, 0.3333333333333333703, 0.3333333333333333703, 0.3333333333333333703, 0.3333333333333333703, 0.3333333333333333703, 0.3333333333333333703, 0.3333333333333333703, 0.3333333333333333703, 0.3333333333333333703, 0.3333333333333333703, 0.3333333333333333703, 0.3333333333333333703, 0.3333333333333333703, 0.3333333333333333703, 0.3333333333333333703, 0.3333333333333333703, 0.3333333333333333703, 0.3333333333333333703, 0.3333333333333333703, 0.3333333333333333703, 0.3333333333333333703, 0.3333333333333333703, 0.3333333333333333703, 0.3333333333333333703, 0.3333333333333333703, 0.3333333333333333703, 0.3333333333333333703, 0.3333333333333333703, 0.3333333333333333703, 0.3333333333333333703, 0.3333333333333333703, 0.3333333333333333703, 0.3333333333333333703, 0.3333333333333333703, 0.3333333333333333703, 0.3333333333333333703, 0.3333333333333333703, 0.3333333333333333703, 0.3333333333333333703, 0.3333333333333333703, 0.3333333333333333703, 0.3333333333333333703, 0.3333333333333333703, 0.3333333333333333703),
 ( 1.000000000000000000, 1.000000000000000000, 1.000000000000000000, 1.000000000000000000, 1.000000000000000000, 1.000000000000000000, 1.000000000000000000, 1.000000000000000000, 1.000000000000000000, 1.000000000000000000, 1.000000000000000000, 1.000000000000000000, 1.000000000000000000, 1.000000000000000000, 1.000000000000000000, 1.000000000000000000, 1.000000000000000000, 1.000000000000000000, 1.000000000000000000, 1.000000000000000000, 1.000000000000000000, 1.000000000000000000, 1.000000000000000000, 1.000000000000000000, 1.000000000000000000, 1.000000000000000000, 1.000000000000000000, 1.000000000000000000, 1.000000000000000000, 1.000000000000000000, 1.000000000000000000, 1.000000000000000000, 1.000000000000000000, 1.000000000000000000, 1.000000000000000000, 1.000000000000000000, 1.000000000000000000, 1.000000000000000000, 1.000000000000000000, 1.000000000000000000, 1.000000000000000000, 1.000000000000000000, 1.000000000000000000, 1.000000000000000000, 1.000000000000000000, 1.000000000000000000, 1.000000000000000000, 1.000000000000000000, 1.000000000000000000, 1.000000000000000000, 1.000000000000000000, 1.000000000000000000, 1.000000000000000000, 1.000000000000000000, 1.000000000000000000, 1.000000000000000000, 1.000000000000000000, 1.000000000000000000, 1.000000000000000000, 1.000000000000000000, 1.000000000000000000, 1.000000000000000000, 1.000000000000000000, 1.000000000000000000, 1.000000000000000000, 1.000000000000000000, 1.000000000000000000, 1.000000000000000000, 1.000000000000000000, 1.000000000000000000, 1.000000000000000000, 1.000000000000000000, 1.000000000000000000, 1.000000000000000000, 1.000000000000000000, 1.000000000000000000, 1.000000000000000000, 1.000000000000000000) ) ) 
 REPRESENTATION_ITEM ( '' )  SURFACE ( )  );
#18877=CARTESIAN_POINT ( 'NONE',  ( 9.641350810849047548, 17.66889113945805789, -17.91796598306941135 ) ) ;
#18881=CARTESIAN_POINT ( 'NONE',  ( 12.56022695423237145, 8.580358410770909217, -16.34122335808152826 ) ) ;
#18893=CARTESIAN_POINT ( 'NONE',  ( 9.669138625804738041, 16.22155169136211583, -17.88455067742322413 ) ) ;
#18896=CARTESIAN_POINT ( 'NONE',  ( 23.13192804015912785, -6.366449129859712563, -15.65771855518050870 ) ) ;
#18899=CARTESIAN_POINT ( 'NONE',  ( 26.68443370873975340, -2.140902173977853540, -15.79004130932784555 ) ) ;
#18905=CARTESIAN_POINT ( 'NONE',  ( 28.12266609392075267, -5.599633216697744942, -16.00068813756295327 ) ) ;
#18913=CARTESIAN_POINT ( 'NONE',  ( 10.47204342302745417, 16.45208460095963687, -17.33479495221483901 ) ) ;
#18918=CARTESIAN_POINT ( 'NONE',  ( 13.38350887602579142, 7.627675785621035764, -15.70476675302002612 ) ) ;
#18921=CARTESIAN_POINT ( 'NONE',  ( 22.89472691350227507, 1.279074496056108901, -19.72372301458170796 ) ) ;
#18922=CARTESIAN_POINT ( 'NONE',  ( 11.27712745377669101, 16.67262326781682802, -16.78413812462462573 ) ) ;
#18926=CARTESIAN_POINT ( 'NONE',  ( 9.641350810849047548, 17.66889113945805789, -17.92981046679734547 ) ) ;
#18928=CARTESIAN_POINT ( 'NONE',  ( 9.917015787971365626, 16.40465641526357743, -16.50431533440121257 ) ) ;
#18934=CARTESIAN_POINT ( 'NONE',  ( 10.45306510330410177, 16.53912159438435125, -17.34933906371858114 ) ) ;
#18936=CARTESIAN_POINT ( 'NONE',  ( 36.54859390953724585, -22.18451583373416014, -18.19919658220850778 ) ) ;
#18937=CARTESIAN_POINT ( 'NONE',  ( 24.68825858685077179, -9.385095155728059524, -16.92495907518576104 ) ) ;
#18938=CARTESIAN_POINT ( 'NONE',  ( 23.21730923944814506, -4.364887171357101359, -13.63095412955673247 ) ) ;
#18944=CARTESIAN_POINT ( 'NONE',  ( 34.63381380623899020, -13.58242311684542081, -20.01117170570581649 ) ) ;
#18946=CARTESIAN_POINT ( 'NONE',  ( 26.35635630057183576, -13.06715036242849948, -16.03892985609963873 ) ) ;
#18948=CARTESIAN_POINT ( 'NONE',  ( 29.29807706749550889, -8.594015191909356588, -15.50881839395299444 ) ) ;
#18956=CARTESIAN_POINT ( 'NONE',  ( 10.71920666609040573, 16.63846344887410922, -15.95486870256106648 ) ) ;
#18961=CARTESIAN_POINT ( 'NONE',  ( 9.916953853453376766, 16.40494045485788632, -16.50434094533541085 ) ) ;
#18963=CARTESIAN_POINT ( 'NONE',  ( 9.667670487869566287, 16.22828475907693146, -17.88517164372263579 ) ) ;
#18964=CARTESIAN_POINT ( 'NONE',  ( 20.76503381105741397, 0.5146303624313508518, -20.54264311693622602 ) ) ;
#18967=CARTESIAN_POINT ( 'NONE',  ( 26.32595758385100382, -12.12905223104374386, -14.21117607008287642 ) ) ;
#18971=CARTESIAN_POINT ( 'NONE',  ( 11.05541802266494855, 17.68941098027438841, -17.91029082024824959 ) ) ;
#18973=CARTESIAN_POINT ( 'NONE',  ( 33.23402178976249388, -11.79005478413273522, -18.03234444571244666 ) ) ;
#18978=CARTESIAN_POINT ( 'NONE',  ( 9.144997394934375023, 16.03247451896970688, -17.04129840131518492 ) ) ;
#18979=CARTESIAN_POINT ( 'NONE',  ( 28.04121823296437199, -4.154284946049297211, -14.96295611916008994 ) ) ;
#18985=CARTESIAN_POINT ( 'NONE',  ( 20.37871551743239351, 7.600776799596193456, -17.08157252577618479 ) ) ;
#18986=CARTESIAN_POINT ( 'NONE',  ( 17.68287507214707688, 6.939063861736925354, -15.39301800483504934 ) ) ;
#18995=CARTESIAN_POINT ( 'NONE',  ( 9.641364314812712166, 17.66882920855936590, -17.90209449470656722 ) ) ;
#18996=CARTESIAN_POINT ( 'NONE',  ( 28.63694740700460173, -9.765300015774602826, -17.75617681614052046 ) ) ;
#18997=CARTESIAN_POINT ( 'NONE',  ( 24.38930386813997586, -0.5518329404549096040, -18.38842912410832753 ) ) ;
#18999=CARTESIAN_POINT ( 'NONE',  ( 36.54859105337858693, -23.18450300252589003, -18.42496455282032386 ) ) ;
#19005=CARTESIAN_POINT ( 'NONE',  ( 17.54642605795894994, 9.676486402519270058, -18.74681543856335608 ) ) ;
#19008=CARTESIAN_POINT ( 'NONE',  ( 10.33811696370167077, 18.38618940166710303, -17.91541423781815112 ) ) ;
#19012=CARTESIAN_POINT ( 'NONE',  ( 17.78594395145776019, 10.14170102421038422, -17.68001733040774681 ) ) ;
#19015=CARTESIAN_POINT ( 'NONE',  ( 13.46306793452363770, 5.846312397186087750, -15.11995136480861746 ) ) ;
#19018=CARTESIAN_POINT ( 'NONE',  ( 35.22227017426903473, -20.71851614966110233, -20.19360243392694088 ) ) ;
#19019=CARTESIAN_POINT ( 'NONE',  ( 24.12901349891383163, -0.6887463444711696692, -16.28517635256633156 ) ) ;
#19020=CARTESIAN_POINT ( 'NONE',  ( 18.67986154365276619, -0.9315889389632653339, -17.94220784458306994 ) ) ;
#19021=CARTESIAN_POINT ( 'NONE',  ( 30.18376337559066158, -9.479172175342087669, -16.86143889264288021 ) ) ;
#19030=CARTESIAN_POINT ( 'NONE',  ( 34.85979932414094407, -13.59765634092047470, -19.03716015824713281 ) ) ;
#19031=CARTESIAN_POINT ( 'NONE',  ( 9.642214727206800617, 17.66492910891761525, -17.80644250212319690 ) ) ;
#19035=CARTESIAN_POINT ( 'NONE',  ( 12.03055882466574289, 9.304755949677762317, -16.69027714870545864 ) ) ;
#19047=CARTESIAN_POINT ( 'NONE',  ( 11.24427277393626134, 9.004760228429224966, -17.23264536074314179 ) ) ;
#19048=CARTESIAN_POINT ( 'NONE',  ( 24.00126410897001605, -3.753019607378720757, -14.48453144943877113 ) ) ;
#19049=CARTESIAN_POINT ( 'NONE',  ( 24.70156281743647142, 0.04986695427254615731, -17.03102378627558977 ) ) ;
#19060=CARTESIAN_POINT ( 'NONE',  ( 12.02406503409520333, 9.334315655862766903, -16.69297946412503819 ) ) ;
#19064=CARTESIAN_POINT ( 'NONE',  ( 34.93238815599637803, -19.41622979634004764, -20.17168434421570922 ) ) ;
#19066=CARTESIAN_POINT ( 'NONE',  ( 13.92371455371928590, 7.866402339252101861, -15.27421329262669936 ) ) ;
#19071=CARTESIAN_POINT ( 'NONE',  ( 17.88091890332929523, 4.544920326333207861, -13.91018511019278669 ) ) ;
#19072=CARTESIAN_POINT ( 'NONE',  ( 12.70256148071318414, 10.13540111970991653, -16.19467101188346092 ) ) ;
#19076=CARTESIAN_POINT ( 'NONE',  ( 11.44040408106239326, 9.418203516307107392, -15.87434068686103394 ) ) ;
#19078=CARTESIAN_POINT ( 'NONE',  ( 9.914377700407460026, 16.41675502110963336, -16.50544604630902867 ) ) ;
#19083=CARTESIAN_POINT ( 'NONE',  ( 10.35865266338826984, 16.97210907862488938, -17.91126819201198472 ) ) ;
#19085=CARTESIAN_POINT ( 'NONE',  ( 36.12281451779777797, -20.27171456826661355, -20.44288436412734100 ) ) ;
#19087=CARTESIAN_POINT ( 'NONE',  ( 28.75197783424699693, -9.407057218516385433, -18.70835418409691542 ) ) ;
#19088=CARTESIAN_POINT ( 'NONE',  ( 26.08768104250457753, -11.87935956797728210, -17.28510650846989805 ) ) ;
#19090=CARTESIAN_POINT ( 'NONE',  ( 33.19592593216645326, -10.35933293216661610, -17.69446280125821147 ) ) ;
#19092=CARTESIAN_POINT ( 'NONE',  ( 19.55510877418759819, -0.09764134006120470111, -19.21341144728512518 ) ) ;
#19093=CARTESIAN_POINT ( 'NONE',  ( 29.00298259868716499, -8.617193473538632631, -14.90553363820342092 ) ) ;
#19104=CARTESIAN_POINT ( 'NONE',  ( 12.27593128402378753, 9.499125914797495795, -15.31109449298900671 ) ) ;
#19110=CARTESIAN_POINT ( 'NONE',  ( 11.39177520167864266, 9.641221755901229429, -15.89445043910815336 ) ) ;
#19112=CARTESIAN_POINT ( 'NONE',  ( 20.46796597391333350, 5.758383238370681667, -16.38968713894368534 ) ) ;
#19113=CARTESIAN_POINT ( 'NONE',  ( 31.84774147790582433, -10.54213090804960018, -15.00000000011102763 ) ) ;
#19117=CARTESIAN_POINT ( 'NONE',  ( 11.28117986039200815, 16.65403841451731637, -16.78246231193739035 ) ) ;
#19119=CARTESIAN_POINT ( 'NONE',  ( 33.66936448658974257, -12.74213349194280553, -18.74758104053764995 ) ) ;
#19120=CARTESIAN_POINT ( 'NONE',  ( 19.91209246711783010, 5.411768277715644615, -14.29674560697521457 ) ) ;
#19123=CARTESIAN_POINT ( 'NONE',  ( 9.098468484354940600, 16.24586203394349582, -17.06302340752861824 ) ) ;
#19124=CARTESIAN_POINT ( 'NONE',  ( 30.28780241637438664, -8.987295266975118935, -19.34112676082218840 ) ) ;
#19127=CARTESIAN_POINT ( 'NONE',  ( 21.10828700581006601, 3.717818950362942854, -18.90958453460783417 ) ) ;
#19128=CARTESIAN_POINT ( 'NONE',  ( 18.48188012193690710, 6.385789046977964567, -18.71539758422269628 ) ) ;
#19142=CARTESIAN_POINT ( 'NONE',  ( 9.910898653440767703, 16.43271037397421708, -16.50709950392603531 ) ) ;
#19144=CARTESIAN_POINT ( 'NONE',  ( 27.63516133065608926, -10.68623331565014034, -17.71408682504818088 ) ) ;
#19145=CARTESIAN_POINT ( 'NONE',  ( 19.75232399841803854, 1.290101960903724754, -14.36573431580270999 ) ) ;
#19146=CARTESIAN_POINT ( 'NONE',  ( 34.84906220094974572, -20.04189041930405324, -21.18881845514476581 ) ) ;
#19152=CARTESIAN_POINT ( 'NONE',  ( 18.55171814111300321, 6.637122934506423988, -19.73184648383247364 ) ) ;
#19155=CARTESIAN_POINT ( 'NONE',  ( 10.33830461362823883, 18.38532881518400686, -17.85494544563047370 ) ) ;
#19159=CARTESIAN_POINT ( 'NONE',  ( 19.05868480923028940, 8.129737193291200370, -16.02886444249750042 ) ) ;
#19160=CARTESIAN_POINT ( 'NONE',  ( 15.74206018803408469, 8.560804325426111916, -21.16119476544194100 ) ) ;
#19162=CARTESIAN_POINT ( 'NONE',  ( 33.68411698100747032, -13.80840863474736935, -19.79436191385186916 ) ) ;
#19163=CARTESIAN_POINT ( 'NONE',  ( 21.44242187996815119, -3.785596145164559445, -16.19382493935754397 ) ) ;
#19164=CARTESIAN_POINT ( 'NONE',  ( 21.26848695057635297, 1.468789200266592099, -19.53654423682621299 ) ) ;
#19167=CARTESIAN_POINT ( 'NONE',  ( 26.63012090756776828, -10.30360588212082007, -13.56444477573641905 ) ) ;
#19176=CARTESIAN_POINT ( 'NONE',  ( 31.87116100697361887, -10.15812870475309815, -13.95024105943860171 ) ) ;
#19177=CARTESIAN_POINT ( 'NONE',  ( 9.641350810849047548, 17.66889113945805789, -23.00000000000000711 ) ) ;
#19181=CARTESIAN_POINT ( 'NONE',  ( 12.01798642417223739, 9.362192935812041483, -16.69549318315592856 ) ) ;
#19190=CARTESIAN_POINT ( 'NONE',  ( 11.21994398240249957, 9.109360644301018439, -17.24323810967081982 ) ) ;
#19191=CARTESIAN_POINT ( 'NONE',  ( 22.62754675296084983, -4.373583220233932423, -15.05708262856468060 ) ) ;
#19192=CARTESIAN_POINT ( 'NONE',  ( 24.47846259200217034, 0.2319951948203725633, -15.89054235832688278 ) ) ;
#19204=CARTESIAN_POINT ( 'NONE',  ( 11.12037835888041393, 13.47873794165536410, -17.06668569338069830 ) ) ;
#19208=CARTESIAN_POINT ( 'NONE',  ( 13.44731269622883296, 7.655871835264917102, -15.65391398210326201 ) ) ;
#19210=CARTESIAN_POINT ( 'NONE',  ( 19.18841159021359033, -2.222386543571284179, -18.22349448661670834 ) ) ;
#19211=CARTESIAN_POINT ( 'NONE',  ( 12.83225835781710344, 9.540595166069421040, -16.14103675596956933 ) ) ;
#19214=CARTESIAN_POINT ( 'NONE',  ( 11.47269659055779378, 9.270105954394804115, -15.86098659800193644 ) ) ;
#19217=CARTESIAN_POINT ( 'NONE',  ( 9.920751600319857033, 16.38752350362809551, -16.50277044458016107 ) ) ;
#19223=CARTESIAN_POINT ( 'NONE',  ( 13.09695832212169364, 8.559710067821024282, -15.93310406974445392 ) ) ;
#19225=CARTESIAN_POINT ( 'NONE',  ( 32.94969931363368687, -9.746457777152386370, -18.95700739231402920 ) ) ;
#19226=CARTESIAN_POINT ( 'NONE',  ( 17.06037746458228810, 10.50611453990982191, -19.02300506704843741 ) ) ;
#19227=CARTESIAN_POINT ( 'NONE',  ( 28.01381056668970260, -10.10121741814351459, -18.82353034625045041 ) ) ;
#19231=CARTESIAN_POINT ( 'NONE',  ( 33.25614251967556356, -10.36847857886694868, -17.86465469861353483 ) ) ;
#19235=CARTESIAN_POINT ( 'NONE',  ( 16.89975486243277913, 3.514059009776604015, -17.86885937027150817 ) ) ;
#19237=CARTESIAN_POINT ( 'NONE',  ( 27.38292679376507266, -11.43094998702963849, -14.23096243513112036 ) ) ;
#19246=CARTESIAN_POINT ( 'NONE',  ( 12.27694278248960558, 9.494486990809335225, -15.31067620760345527 ) ) ;
#19251=CARTESIAN_POINT ( 'NONE',  ( 12.39803340617553928, 8.535179507765855433, -15.21071672276548625 ) ) ;
#19252=CARTESIAN_POINT ( 'NONE',  ( 18.66675855576620791, -1.414919486740021881, -19.12600662388792117 ) ) ;
#19259=CARTESIAN_POINT ( 'NONE',  ( 12.84300253770136990, 9.521034635873322216, -16.13432743836305505 ) ) ;
#19261=CARTESIAN_POINT ( 'NONE',  ( 33.61574637963836665, -12.50126044309498496, -18.73137083807847958 ) ) ;
#19262=CARTESIAN_POINT ( 'NONE',  ( 16.57956996521092918, 4.788269978297743812, -19.71382457362092566 ) ) ;
#19266=CARTESIAN_POINT ( 'NONE',  ( 25.84292692831908766, -2.469955994367391661, -17.24682881138801704 ) ) ;
#19271=CARTESIAN_POINT ( 'NONE',  ( 24.59961324288297391, 0.2024632608770970121, -16.27125138369466484 ) ) ;
#19273=CARTESIAN_POINT ( 'NONE',  ( 15.83821057800014920, 6.120979864746498578, -15.70533851924537672 ) ) ;
#19287=CARTESIAN_POINT ( 'NONE',  ( 11.46775782571576130, 9.292755756535285627, -15.86302895122203616 ) ) ;
#19288=CARTESIAN_POINT ( 'NONE',  ( 27.54771222089439320, -11.35863810494041459, -14.08592588049474692 ) ) ;
#19289=CARTESIAN_POINT ( 'NONE',  ( 22.16683763302808430, -0.5050174593055701822, -13.96310542101677044 ) ) ;
#19290=CARTESIAN_POINT ( 'NONE',  ( 35.54859390953724585, -23.18451583373416014, -17.78191007148576119 ) ) ;
#19298=CARTESIAN_POINT ( 'NONE',  ( 23.36212950203212557, 2.915605996956767587, -15.34809340432955693 ) ) ;
#19300=CARTESIAN_POINT ( 'NONE',  ( 10.33886748782435561, 18.38274740237080351, -17.79416814676874381 ) ) ;
#19304=CARTESIAN_POINT ( 'NONE',  ( 19.71807001554888217, -1.708786246101231532, -19.21472004699903380 ) ) ;
#19305=CARTESIAN_POINT ( 'NONE',  ( 13.78422571733443647, 6.778978001458615843, -20.29761332830707232 ) ) ;
#19307=CARTESIAN_POINT ( 'NONE',  ( 33.27037009343090546, -12.05169513820189309, -19.60996450177851713 ) ) ;
#19308=CARTESIAN_POINT ( 'NONE',  ( 27.22116495027615812, -8.412805768781604243, -11.93592671293571605 ) ) ;
#19311=CARTESIAN_POINT ( 'NONE',  ( 18.22321846687148650, 1.664438589611230812, -15.57940112478783945 ) ) ;
#19322=CARTESIAN_POINT ( 'NONE',  ( 36.54859590101256828, -22.18452478037840336, -18.26685560724362034 ) ) ;
#19324=CARTESIAN_POINT ( 'NONE',  ( 9.641350810849047548, 17.66889113945805789, -17.91752729848689185 ) ) ;
#19328=CARTESIAN_POINT ( 'NONE',  ( 12.02932678857878734, 9.310239991255825132, -16.69079931733866218 ) ) ;
#19338=CARTESIAN_POINT ( 'NONE',  ( 11.21386537247953363, 9.137237924250291243, -17.24575182870169598 ) ) ;
#19339=CARTESIAN_POINT ( 'NONE',  ( 25.04368804655567970, -3.332730676350641463, -14.85212872609148427 ) ) ;
#19341=CARTESIAN_POINT ( 'NONE',  ( 22.96196402503608169, -2.069733343145511828, -19.51364111617685992 ) ) ;
#19354=CARTESIAN_POINT ( 'NONE',  ( 12.01798642417223739, 9.362192935812041483, -16.69549318315592856 ) ) ;
#19356=CARTESIAN_POINT ( 'NONE',  ( 32.73840480032550460, -11.71477781474665925, -16.63156947497440541 ) ) ;
#19358=CARTESIAN_POINT ( 'NONE',  ( 13.51537010444165254, 7.685947621549766851, -15.59967102646339043 ) ) ;
#19361=CARTESIAN_POINT ( 'NONE',  ( 21.57856661146780652, -4.666631351218505586, -18.28211233923166645 ) ) ;
#19362=CARTESIAN_POINT ( 'NONE',  ( 12.83173194157631514, 9.543008920787411142, -16.14125448247791184 ) ) ;
#19368=CARTESIAN_POINT ( 'NONE',  ( 11.48043977940431226, 9.236673419044803879, -15.85762597608872326 ) ) ;
#19370=CARTESIAN_POINT ( 'NONE',  ( 9.936961226781097167, 16.31318409042999917, -16.49606719383117337 ) ) ;
#19375=CARTESIAN_POINT ( 'NONE',  ( 12.05017172662707381, 9.228765020691243492, -16.68110209197688221 ) ) ;
#19377=CARTESIAN_POINT ( 'NONE',  ( 36.54859390953724585, -23.18451583373416014, -17.64281456791166391 ) ) ;
#19378=CARTESIAN_POINT ( 'NONE',  ( 25.24878800877705487, -9.370948223588685622, -14.18615728435988288 ) ) ;
#19379=CARTESIAN_POINT ( 'NONE',  ( 29.76939623719675510, -8.219725197086590995, -17.35520659559267287 ) ) ;
#19384=CARTESIAN_POINT ( 'NONE',  ( 34.38415957124060895, -12.46085888452578594, -19.93570721963346060 ) ) ;
#19385=CARTESIAN_POINT ( 'NONE',  ( 21.44849557978440657, 3.047722651366359781, -15.04725200041975341 ) ) ;
#19386=CARTESIAN_POINT ( 'NONE',  ( 15.22033579473957410, 7.355362781181614018, -19.64495939069069763 ) ) ;
#19395=CARTESIAN_POINT ( 'NONE',  ( 12.27693042220145969, 9.494543488390625896, -15.31068133337694803 ) ) ;
#19401=CARTESIAN_POINT ( 'NONE',  ( 12.50268541164654756, 8.571888915454989544, -15.12803469218787811 ) ) ;
#19404=CARTESIAN_POINT ( 'NONE',  ( 16.22630451241072436, 4.170241327582352220, -17.06284370071109535 ) ) ;
#19411=CARTESIAN_POINT ( 'NONE',  ( 12.79981923948071554, 9.689364640521217709, -16.15445150739013158 ) ) ;
#19414=CARTESIAN_POINT ( 'NONE',  ( 34.49426285277334614, -12.00696374527110066, -18.89673795385250799 ) ) ;
#19415=CARTESIAN_POINT ( 'NONE',  ( 21.41025690189560748, 5.821651141963339882, -16.00656683556521998 ) ) ;
#19418=CARTESIAN_POINT ( 'NONE',  ( 28.90796184913828171, -12.27476343136570414, -11.88515153054143347 ) ) ;
#19423=CARTESIAN_POINT ( 'NONE',  ( 19.47299019774181161, -1.479546722229555744, -17.51644493673600067 ) ) ;
#19424=CARTESIAN_POINT ( 'NONE',  ( 19.07048665705943336, 2.338351316274200453, -13.70053041002553407 ) ) ;
#19433=CARTESIAN_POINT ( 'NONE',  ( 11.45256130090833935, 9.362448956408465861, -15.86931324879919991 ) ) ;
#19435=CARTESIAN_POINT ( 'NONE',  ( 29.40876261992080032, -8.787110225502646088, -16.42709622331022956 ) ) ;
#19436=CARTESIAN_POINT ( 'NONE',  ( 26.00956027078203192, -8.595392566010074731, -19.46287731774799212 ) ) ;
#19438=CARTESIAN_POINT ( 'NONE',  ( 35.51409509342218485, -23.02953092745895347, -19.29936871477319826 ) ) ;
#19449=CARTESIAN_POINT ( 'NONE',  ( 16.06572049258021195, 3.735912457719189117, -15.00855390560170477 ) ) ;
#19452=CARTESIAN_POINT ( 'NONE',  ( 12.25826188308600351, 9.517053581970603915, -15.32321445922237224 ) ) ;
#19455=CARTESIAN_POINT ( 'NONE',  ( 18.98200677837107264, -2.562081333921657933, -16.63161468174866187 ) ) ;
#19456=CARTESIAN_POINT ( 'NONE',  ( 18.53087132295907935, 5.398958961476600038, -21.24745519132487459 ) ) ;
#19458=CARTESIAN_POINT ( 'NONE',  ( 32.48283477683061449, -11.02614750807341260, -17.91093295056291979 ) ) ;
#19461=CARTESIAN_POINT ( 'NONE',  ( 26.37963984661160310, -4.639223599391875119, -13.30093322687953616 ) ) ;
#19462=CARTESIAN_POINT ( 'NONE',  ( 22.33718609693395862, 3.185771058179875492, -16.53122240148476152 ) ) ;
#19464=ORIENTED_EDGE ( 'NONE', *, *, #18000, .T. ) ;
#19465=CARTESIAN_POINT ( 'NONE',  ( 22.16846437878366061, -4.107540447007581363, -19.06500358040360865 ) ) ;
#19472=CARTESIAN_POINT ( 'NONE',  ( 14.73435313093308174, 9.569269045654692718, -13.91804818168885305 ) ) ;
#19473=CARTESIAN_POINT ( 'NONE',  ( 35.06179249480944549, -15.50510465796065596, -20.14053939611612520 ) ) ;
#19475=CARTESIAN_POINT ( 'NONE',  ( 9.893572868141015775, 16.51216863388285461, -16.51808063826580408 ) ) ;
#19482=CARTESIAN_POINT ( 'NONE',  ( 12.02761088988360783, 9.318053909225662679, -16.69151312802368636 ) ) ;
#19493=CARTESIAN_POINT ( 'NONE',  ( 11.15915788317279578, 9.388133443793682531, -17.26837529997955301 ) ) ;
#19494=CARTESIAN_POINT ( 'NONE',  ( 15.74206018803408469, 8.560804325426111916, -21.16119476544194100 ) ) ;
#19495=CARTESIAN_POINT ( 'NONE',  ( 24.59961324288297391, 0.2024632608770970121, -16.27125138369466484 ) ) ;
#19508=CARTESIAN_POINT ( 'NONE',  ( 12.02609123740286101, 9.325023229212996867, -16.69214155778140096 ) ) ;
#19509=CARTESIAN_POINT ( 'NONE',  ( 33.47764622482974062, -12.08535443106849883, -18.57070694247861553 ) ) ;
#19511=CARTESIAN_POINT ( 'NONE',  ( 10.14999423553203606, 11.42343090068832190, -16.62569685487721571 ) ) ;
#19513=CARTESIAN_POINT ( 'NONE',  ( 23.60870351872479844, -7.222488552757559077, -14.83554404960226947 ) ) ;
#19515=CARTESIAN_POINT ( 'NONE',  ( 12.83192189813640738, 9.542137755788996145, -16.14117592875819440 ) ) ;
#19522=CARTESIAN_POINT ( 'NONE',  ( 11.47155695691762212, 9.275332456566969697, -15.86145787682774078 ) ) ;
#19527=CARTESIAN_POINT ( 'NONE',  ( 11.86602117609799301, 10.05912493454434120, -16.75833615892761586 ) ) ;
#19529=CARTESIAN_POINT ( 'NONE',  ( 22.66942224714451370, 5.529188492372526298, -17.57712505567429773 ) ) ;
#19530=CARTESIAN_POINT ( 'NONE',  ( 13.25083620024415332, 6.663885870737293438, -17.30077526834593016 ) ) ;
#19534=CARTESIAN_POINT ( 'NONE',  ( 36.18478257229246964, -20.55010421171508028, -20.40673782175607442 ) ) ;
#19538=CARTESIAN_POINT ( 'NONE',  ( 19.19659130220728116, 4.347481709847851761, -15.16398724834160916 ) ) ;
#19540=CARTESIAN_POINT ( 'NONE',  ( 21.66440995182641416, 5.535554982823286174, -17.57621636221614025 ) ) ;
#19548=CARTESIAN_POINT ( 'NONE',  ( 11.23952829215726901, 14.25220214615140257, -15.73968358775164056 ) ) ;
#19555=CARTESIAN_POINT ( 'NONE',  ( 12.55500454421123457, 8.595009676161804890, -15.08633542003848049 ) ) ;
#19556=CARTESIAN_POINT ( 'NONE',  ( 10.67622114788023246, 9.011142735252827052, -16.40800301137445416 ) ) ;
#19563=CARTESIAN_POINT ( 'NONE',  ( 12.83296646064745339, 9.537815246119466295, -16.14070827264395547 ) ) ;
#19564=CARTESIAN_POINT ( 'NONE',  ( 32.48803055552120611, -10.90163289162770432, -13.69202896798154256 ) ) ;
#19565=CARTESIAN_POINT ( 'NONE',  ( 19.51440197245297270, 8.071880087464508691, -17.28625796899888201 ) ) ;
#19569=CARTESIAN_POINT ( 'NONE',  ( 26.40146419187390947, -13.39824708621661919, -13.49681364666919059 ) ) ;
#19574=CARTESIAN_POINT ( 'NONE',  ( 20.59283418570449697, -4.290598171560842111, -16.90930062131523215 ) ) ;
#19575=CARTESIAN_POINT ( 'NONE',  ( 18.89276694006714052, 5.271756288042509730, -14.92826338805148190 ) ) ;
#19584=CARTESIAN_POINT ( 'NONE',  ( 11.47511325496290624, 9.259230714725578792, -15.85997136665693041 ) ) ;
#19585=CARTESIAN_POINT ( 'NONE',  ( 27.32111546295355708, -6.651148440249742499, -13.76656720552121982 ) ) ;
#19586=CARTESIAN_POINT ( 'NONE',  ( 25.46127020808262387, -4.208148299910691392, -19.59612275642668777 ) ) ;
#19595=CARTESIAN_POINT ( 'NONE',  ( 21.48529164538665981, 5.106035544247377267, -18.65531623833433628 ) ) ;
#19598=CARTESIAN_POINT ( 'NONE',  ( 12.27441163154304071, 9.506095234784829984, -15.31172292274672664 ) ) ;
#19601=CARTESIAN_POINT ( 'NONE',  ( 23.86551563699305234, 2.542095107771292106, -17.79649620197707094 ) ) ;
#19603=CARTESIAN_POINT ( 'NONE',  ( 19.82966512453777952, 6.730073478465656400, -20.48479553209826065 ) ) ;
#19606=DIRECTION ( 'NONE',  ( 0.000000000000000000, 0.000000000000000000, 1.000000000000000000 ) ) ;
#19607=CARTESIAN_POINT ( 'NONE',  ( 25.62874891556376511, -2.832145142407604510, -18.00902499482074148 ) ) ;
#19609=CARTESIAN_POINT ( 'NONE',  ( 22.91777464530744268, -8.256078323855359002, -14.14386909076557686 ) ) ;
#19613=CARTESIAN_POINT ( 'NONE',  ( 26.36224721256908410, -8.875037662531589433, -13.49479840426202948 ) ) ;
#19622=CARTESIAN_POINT ( 'NONE',  ( 33.78657425947636739, -10.78854458652579495, -19.16640759269550287 ) ) ;
#19623=CARTESIAN_POINT ( 'NONE',  ( 9.936961226781097167, 16.31318409042999917, -16.49606719383117337 ) ) ;
#19626=CARTESIAN_POINT ( 'NONE',  ( 13.12404665403065707, 8.571044468271947991, -15.91156272984762765 ) ) ;
#19637=CARTESIAN_POINT ( 'NONE',  ( 13.24589568141979612, 7.574869496316740225, -15.81383618087551746 ) ) ;
#19639=CARTESIAN_POINT ( 'NONE',  ( 17.25718654270123409, 10.07213275844434364, -20.48022200034118612 ) ) ;
#19640=CARTESIAN_POINT ( 'NONE',  ( 26.35635630057183576, -13.06715036242849948, -16.03892985609963873 ) ) ;
#19655=CARTESIAN_POINT ( 'NONE',  ( 12.02871927673971619, 9.312984558958580905, -16.69105371450780595 ) ) ;
#19656=CARTESIAN_POINT ( 'NONE',  ( 33.06959603162382422, -11.76507887159725030, -17.56762491042838903 ) ) ;
#19658=CARTESIAN_POINT ( 'NONE',  ( 8.945111769380243771, 16.94917547725161810, -17.84906893764549451 ) ) ;
#19659=CARTESIAN_POINT ( 'NONE',  ( 25.21413058671614849, -1.115224416820481457, -18.44856734933592080 ) ) ;
#19660=CARTESIAN_POINT ( 'NONE',  ( 12.82413367917259706, 9.577855520724041227, -16.14439663126654523 ) ) ;
#19665=CARTESIAN_POINT ( 'NONE',  ( 12.49428694376680049, 8.568214790255201052, -15.13472557389765072 ) ) ;
#19671=CARTESIAN_POINT ( 'NONE',  ( 12.02001262747988797, 9.352900509162292764, -16.69465527681230199 ) ) ;
#19673=CARTESIAN_POINT ( 'NONE',  ( 13.51959648670337444, 7.024181567627514333, -18.72314150793285492 ) ) ;
#19674=CARTESIAN_POINT ( 'NONE',  ( 28.47856004806874353, -11.16640101040803401, -12.66155532224275149 ) ) ;
#19679=CARTESIAN_POINT ( 'NONE',  ( 36.07559364978101968, -20.05957622185551870, -20.44697815928661200 ) ) ;
#19681=CARTESIAN_POINT ( 'NONE',  ( 18.53362878050275597, 1.800236982614616510, -15.18126852959267481 ) ) ;
#19682=CARTESIAN_POINT ( 'NONE',  ( 21.04385110482095200, 5.766204710259658306, -15.30406332615466347 ) ) ;
#19696=CARTESIAN_POINT ( 'NONE',  ( 12.25660130062383146, 9.517454774955181662, -15.32445140518387028 ) ) ;
#19701=CARTESIAN_POINT ( 'NONE',  ( 11.55687758731922798, 9.016417257711555777, -15.81607864292198329 ) ) ;
#19703=CARTESIAN_POINT ( 'NONE',  ( 10.66838568802538845, 9.046021620013140918, -16.41132375377494057 ) ) ;
#19708=CARTESIAN_POINT ( 'NONE',  ( 12.83225436833568089, 9.540613290865683993, -16.14103841883858337 ) ) ;
#19709=CARTESIAN_POINT ( 'NONE',  ( 34.93112910557051976, -13.91810326443952306, -19.05872143998290014 ) ) ;
#19710=CARTESIAN_POINT ( 'NONE',  ( 14.29829396236512729, 6.476847147513518088, -18.28004444394726491 ) ) ;
#19713=CARTESIAN_POINT ( 'NONE',  ( 16.02150382621726976, 6.204807860950024789, -14.00014022580063155 ) ) ;
#19717=CARTESIAN_POINT ( 'NONE',  ( 24.77705064808911217, -2.604154092221317551, -13.46095375842554098 ) ) ;
#19718=CARTESIAN_POINT ( 'NONE',  ( 16.84217415841480303, 1.412180072802544872, -16.35713574856416841 ) ) ;
#19731=CARTESIAN_POINT ( 'NONE',  ( 11.47269659055779378, 9.270105954394804115, -15.86098659800193644 ) ) ;
#19732=CARTESIAN_POINT ( 'NONE',  ( 15.87806330829146617, 7.947701475055697351, -19.83831759000646855 ) ) ;
#19733=CARTESIAN_POINT ( 'NONE',  ( 25.71810023473615203, -5.953606672203104466, -12.71518937071605038 ) ) ;
#19741=CARTESIAN_POINT ( 'NONE',  ( 17.72480397827495224, 1.356124466512965476, -19.40231245121514903 ) ) ;
#19744=CARTESIAN_POINT ( 'NONE',  ( 12.27697253541231426, 9.494350595542041304, -15.31066389949581463 ) ) ;
#19748=CARTESIAN_POINT ( 'NONE',  ( 22.51149892830068211, -1.106640851078940502, -13.23823320067571885 ) ) ;
#19750=CARTESIAN_POINT ( 'NONE',  ( 18.68528716101036480, 3.575476808761081760, -13.14399490972872186 ) ) ;
#19754=CARTESIAN_POINT ( 'NONE',  ( 23.14387462191455214, -5.292040767005758539, -18.71731562455695297 ) ) ;
#19755=CARTESIAN_POINT ( 'NONE',  ( 27.03394943597420408, -2.104382873295748801, -14.19367964525161163 ) ) ;
#19765=CARTESIAN_POINT ( 'NONE',  ( 13.78676817088038931, 5.425489125369224119, -17.89072192914586168 ) ) ;
#19766=CARTESIAN_POINT ( 'NONE',  ( 34.35798975979065517, -12.34328324435382207, -19.92780167937219815 ) ) ;
#19767=CARTESIAN_POINT ( 'NONE',  ( 11.14863080475985591, 10.75631295387255548, -15.99499920034263489 ) ) ;
#19771=CARTESIAN_POINT ( 'NONE',  ( 16.24089679924285790, 9.948436389806387226, -13.42737814189079337 ) ) ;
#19787=CARTESIAN_POINT ( 'NONE',  ( 8.944584698556434788, 16.95159269123564272, -17.91535980893264224 ) ) ;
#19788=CARTESIAN_POINT ( 'NONE',  ( 12.84881458348222516, 5.748695638350556969, -17.40385974964576477 ) ) ;
#19789=CARTESIAN_POINT ( 'NONE',  ( 24.51672896724849338, -10.45039314358892035, -14.45231470433035170 ) ) ;
#19806=CARTESIAN_POINT ( 'NONE',  ( 13.13744203029165369, 8.576964204390579383, -15.90088637244482150 ) ) ;
#19807=CARTESIAN_POINT ( 'NONE',  ( 33.15992091288699584, -11.77879734164826786, -17.82291275646110407 ) ) ;
#19809=CARTESIAN_POINT ( 'NONE',  ( 9.112894736278665420, 16.17970140370183785, -17.05457397994698709 ) ) ;
#19811=CARTESIAN_POINT ( 'NONE',  ( 25.57370974413349884, -0.4222200280313516685, -16.88676729435558599 ) ) ;
#19812=CARTESIAN_POINT ( 'NONE',  ( 10.35866308580767026, 16.97206128008099313, -17.90676409391864610 ) ) ;
#19819=CARTESIAN_POINT ( 'NONE',  ( 12.37169234869624646, 8.529253869913038244, -15.23127513898213081 ) ) ;
#19825=CARTESIAN_POINT ( 'NONE',  ( 12.03006260835556951, 9.306948544855226046, -16.69048869075990638 ) ) ;
#19828=CARTESIAN_POINT ( 'NONE',  ( 18.86526831082781541, 1.353360947173176232, -20.65364330072180366 ) ) ;
#19829=CARTESIAN_POINT ( 'NONE',  ( 20.04052888069229610, 8.940267654624740601, -17.40200224619232117 ) ) ;
#19834=CARTESIAN_POINT ( 'NONE',  ( 17.29421355564066332, 9.360779442694735053, -19.18964209290773937 ) ) ;
#19844=CARTESIAN_POINT ( 'NONE',  ( 11.05541533671906684, 17.68942329836457361, -17.91521986731755334 ) ) ;
#19850=CARTESIAN_POINT ( 'NONE',  ( 12.50396148805030627, 8.572452836447732594, -15.12701763676990119 ) ) ;
#19853=CARTESIAN_POINT ( 'NONE',  ( 12.49426214472998176, 7.541115143590324088, -15.13238550383361769 ) ) ;
#19862=CARTESIAN_POINT ( 'NONE',  ( 12.76739998655820685, 9.838043466917183011, -16.16785800888773394 ) ) ;
#19863=CARTESIAN_POINT ( 'NONE',  ( 33.78268718695997563, -11.09826429569044670, -17.35115476112383348 ) ) ;
#19864=CARTESIAN_POINT ( 'NONE',  ( 19.18841159021359033, -2.222386543571284179, -18.22349448661670834 ) ) ;
#19868=CARTESIAN_POINT ( 'NONE',  ( 15.10175627602374249, 9.741420229655037843, -13.89989488922661742 ) ) ;
#19871=CARTESIAN_POINT ( 'NONE',  ( 19.39248696316839116, -1.610358169686434193, -16.91126230894791860 ) ) ;
#19873=CARTESIAN_POINT ( 'NONE',  ( 19.38139026969670553, 5.460277215109251792, -15.14974238112136540 ) ) ;
#19885=CARTESIAN_POINT ( 'NONE',  ( 11.22458689634746776, 9.088074461393535586, -17.24131758186684138 ) ) ;
#19886=CARTESIAN_POINT ( 'NONE',  ( 11.47288049726737214, 9.269262779257836371, -15.86091052746238184 ) ) ;
#19887=CARTESIAN_POINT ( 'NONE',  ( 23.87675077653036126, -6.787291307973906562, -13.16608595595566733 ) ) ;
#19897=CARTESIAN_POINT ( 'NONE',  ( 19.61192361542596529, -2.405681417800469291, -14.70675912396028906 ) ) ;
#19903=CARTESIAN_POINT ( 'NONE',  ( 12.27187887740847039, 9.517710768097034091, -15.31277030567625452 ) ) ;
#19908=CARTESIAN_POINT ( 'NONE',  ( 20.39549844898813191, -2.061726703908969505, -13.85117726305786512 ) ) ;
#19910=CARTESIAN_POINT ( 'NONE',  ( 15.90442531705523876, 3.007083446286336947, -19.83189509879157697 ) ) ;
#19912=CARTESIAN_POINT ( 'NONE',  ( 35.54859390953724585, -22.18451583373416014, -17.64281456791166036 ) ) ;
#19915=CARTESIAN_POINT ( 'NONE',  ( 28.44965076230254653, -4.228683950944192027, -16.16799691904953562 ) ) ;
#19916=CARTESIAN_POINT ( 'NONE',  ( 18.73701609394335321, -1.228702115187185973, -15.37238819164404369 ) ) ;
#19928=CARTESIAN_POINT ( 'NONE',  ( 23.59197141788265384, -6.183129490800155281, -14.78464116683282015 ) ) ;
#19930=CARTESIAN_POINT ( 'NONE',  ( 34.49115424338278046, -12.94152926980570939, -19.96804914223585925 ) ) ;
#19932=CARTESIAN_POINT ( 'NONE',  ( 9.898178882064430084, 16.49104486689975246, -16.51464960819000893 ) ) ;
#19935=CARTESIAN_POINT ( 'NONE',  ( 9.661883061612440926, 16.25482663361732705, -17.91664992932185996 ) ) ;
#19939=CARTESIAN_POINT ( 'NONE',  ( 11.46471852075427478, 9.306694396509932687, -15.86428581073749378 ) ) ;
#19945=STYLED_ITEM ( 'NONE', ( #3796 ), #1479 ) ;
#19947=CARTESIAN_POINT ( 'NONE',  ( 13.37894900189793290, 7.625660844661456217, -15.70840104182326513 ) ) ;
#19948=CARTESIAN_POINT ( 'NONE',  ( 31.02293300316137348, -10.15460426738793664, -15.78645847904462052 ) ) ;
#19950=CARTESIAN_POINT ( 'NONE',  ( 29.60394739741320080, -6.827861936862228198, -14.22031441372854843 ) ) ;
#19951=CARTESIAN_POINT ( 'NONE',  ( 24.97892660363778106, -6.291154998746494087, -12.74939059104742256 ) ) ;
#19962=ORIENTED_EDGE ( 'NONE', *, *, #2685, .T. ) ;
#19966=CARTESIAN_POINT ( 'NONE',  ( 13.12174330432777047, 8.570030634161971861, -15.91339823077023929 ) ) ;
#19967=CARTESIAN_POINT ( 'NONE',  ( 33.40448403937627830, -11.94904316976568914, -18.43672998654903239 ) ) ;
#19969=CARTESIAN_POINT ( 'NONE',  ( 9.144997394934375023, 16.03247451896970688, -17.04129840131518492 ) ) ;
#19971=CARTESIAN_POINT ( 'NONE',  ( 26.47492910780048447, -3.130564378024159211, -15.09640780237150892 ) ) ;
#19972=CARTESIAN_POINT ( 'NONE',  ( 12.87010724449035415, 9.516853939945930208, -16.11395691550788101 ) ) ;
#19977=CARTESIAN_POINT ( 'NONE',  ( 11.51951884677450266, 9.108496074915260365, -15.83757232928968683 ) ) ;
#19983=CARTESIAN_POINT ( 'NONE',  ( 13.19188795686497429, 8.601024833420110483, -15.85749200792911573 ) ) ;
#19986=CARTESIAN_POINT ( 'NONE',  ( 15.79264427988833219, 7.655968387373099482, -13.90199225654327897 ) ) ;
#19987=CARTESIAN_POINT ( 'NONE',  ( 22.09051738352356153, 1.573095004317974333, -13.27920415769822426 ) ) ;
#19992=CARTESIAN_POINT ( 'NONE',  ( 36.54859390953724585, -22.18451583373416014, -17.64281456791166036 ) ) ;
#19993=CARTESIAN_POINT ( 'NONE',  ( 15.94478687392618355, 4.193953704849600506, -19.05305658475056063 ) ) ;
#20004=CARTESIAN_POINT ( 'NONE',  ( 34.75406370242679799, -18.61511248754081294, -20.11778113987843852 ) ) ;
#20008=CARTESIAN_POINT ( 'NONE',  ( 12.24710219714225268, 9.516853694884586545, -15.33174803936941366 ) ) ;
#20009=CARTESIAN_POINT ( 'NONE',  ( 33.27037009343090546, -12.05169513820189309, -19.60996450177851713 ) ) ;
#20013=CARTESIAN_POINT ( 'NONE',  ( 12.54775956925048774, 7.553149829897631840, -15.09063234640338003 ) ) ;
#20018=CARTESIAN_POINT ( 'NONE',  ( 12.86829554393394659, 9.516053645290590168, -16.11540084779614546 ) ) ;
#20020=CARTESIAN_POINT ( 'NONE',  ( 36.29797175594614345, -20.05860325589622661, -19.47188034632657150 ) ) ;
#20022=CARTESIAN_POINT ( 'NONE',  ( 22.51149892830068211, -1.106640851078940502, -13.23823320067571885 ) ) ;
#20028=CARTESIAN_POINT ( 'NONE',  ( 22.75855789899217640, -7.280205122891536540, -14.30210469086359915 ) ) ;
#20029=CARTESIAN_POINT ( 'NONE',  ( 17.05751464226099401, 1.788256342680895949, -18.14502383782993888 ) ) ;
#20044=CARTESIAN_POINT ( 'NONE',  ( 11.22373969136065242, 9.091953032947756697, -17.24166845096988609 ) ) ;
#20046=CARTESIAN_POINT ( 'NONE',  ( 10.33811693838771717, 18.38618951776012267, -17.91796598306941135 ) ) ;
#20047=CARTESIAN_POINT ( 'NONE',  ( 26.86433939054618492, -2.362129714094441724, -16.96571632802953644 ) ) ;
#20052=CARTESIAN_POINT ( 'NONE',  ( 9.910898653440767703, 16.43271037397421708, -16.50709950392603531 ) ) ;
#20054=CARTESIAN_POINT ( 'NONE',  ( 24.81358459371387326, -5.676498915796258871, -18.90393244824272756 ) ) ;
#20057=CARTESIAN_POINT ( 'NONE',  ( 12.27670864112623583, 9.495496515443743846, -15.31077793565516565 ) ) ;
#20058=CARTESIAN_POINT ( 'NONE',  ( 31.15806985163746390, -10.82494328065958911, -14.16671120874331358 ) ) ;
#20060=CARTESIAN_POINT ( 'NONE',  ( 25.73595588610537277, -4.826321120321507507, -18.84379041344559269 ) ) ;
#20062=CARTESIAN_POINT ( 'NONE',  ( 22.65699622776610411, 4.567421951779635947, -17.29570926971318556 ) ) ;
#20064=CARTESIAN_POINT ( 'NONE',  ( 35.54859390953724585, -22.18451583373416014, -17.22552805718784441 ) ) ;
#20066=CARTESIAN_POINT ( 'NONE',  ( 18.35279563442798079, 9.979516425631709708, -19.26739628155305439 ) ) ;
#20067=CARTESIAN_POINT ( 'NONE',  ( 27.84123584509972815, -2.508445798277625371, -17.45642919975013285 ) ) ;
#20069=CARTESIAN_POINT ( 'NONE',  ( 29.76939623719675510, -8.219725197086590995, -17.35520659559267287 ) ) ;
#20083=CARTESIAN_POINT ( 'NONE',  ( 27.58270427615865472, -5.135490454175970498, -17.42064064436273085 ) ) ;
#20085=CARTESIAN_POINT ( 'NONE',  ( 33.60507142094932931, -10.68002793468083134, -20.32431474444524255 ) ) ;
#20087=CARTESIAN_POINT ( 'NONE',  ( 9.920751600319857033, 16.38752350362809551, -16.50277044458016107 ) ) ;
#20090=CARTESIAN_POINT ( 'NONE',  ( 13.13744203029165369, 8.576964204390579383, -15.90088637244482150 ) ) ;
#20093=CARTESIAN_POINT ( 'NONE',  ( 9.936961226781097167, 16.31318409042999917, -16.49606719383117337 ) ) ;
#20100=CARTESIAN_POINT ( 'NONE',  ( 8.944592922245861999, 16.95155497634765851, -17.90742740301624991 ) ) ;
#20101=CARTESIAN_POINT ( 'NONE',  ( 34.83580697690636185, -15.48987143388560384, -21.11455094357481244 ) ) ;
#20102=CARTESIAN_POINT ( 'NONE',  ( 12.89848499713582441, 9.804829593628518580, -14.81257543621576112 ) ) ;
#20103=CARTESIAN_POINT ( 'NONE',  ( 28.67543231808702942, -10.82877479041544433, -19.00874469794426602 ) ) ;
#20115=CARTESIAN_POINT ( 'NONE',  ( 13.25994536507779742, 8.631100619704961119, -15.80324905228922994 ) ) ;
#20116=CARTESIAN_POINT ( 'NONE',  ( 34.33808118748100924, -15.74632339993765484, -18.94971805680347998 ) ) ;
#20117=CARTESIAN_POINT ( 'NONE',  ( 9.112830967032516938, 16.17999385759334885, -17.05460035006107589 ) ) ;
#20120=CARTESIAN_POINT ( 'NONE',  ( 12.86829554393394659, 9.516053645290590168, -16.11540084779614546 ) ) ;
#20126=CARTESIAN_POINT ( 'NONE',  ( 11.92109019680886206, 8.606374460406147620, -15.56934379943068336 ) ) ;
#20130=CARTESIAN_POINT ( 'NONE',  ( 9.661883073086391605, 16.25482658099627642, -17.91571305590050400 ) ) ;
#20133=CARTESIAN_POINT ( 'NONE',  ( 17.64024190839899120, 8.465516882244152441, -14.08803959672746586 ) ) ;
#20134=CARTESIAN_POINT ( 'NONE',  ( 16.96299543436377633, 3.857017182823994084, -13.23919852190412527 ) ) ;
#20138=CARTESIAN_POINT ( 'NONE',  ( 22.51149892830068211, -1.106640851078940502, -13.23823320067571885 ) ) ;
#20144=CARTESIAN_POINT ( 'NONE',  ( 34.93238815599637803, -19.41622979634004764, -20.17168434421570922 ) ) ;
#20149=CARTESIAN_POINT ( 'NONE',  ( 11.05541531668977662, 17.68942339022145305, -17.95086732675816776 ) ) ;
#20150=CARTESIAN_POINT ( 'NONE',  ( 32.74314609665832165, -11.10724048739539782, -18.62249297335446840 ) ) ;
#20152=CARTESIAN_POINT ( 'NONE',  ( 9.641350810849047548, 17.66889113945805789, -19.66666666666842644 ) ) ;
#20154=CARTESIAN_POINT ( 'NONE',  ( 10.63628302936969483, 9.193248504745362482, -16.42459933240677827 ) ) ;
#20159=CARTESIAN_POINT ( 'NONE',  ( 10.35864918915110877, 16.97212501191939538, -17.92279151347709032 ) ) ;
#20162=CARTESIAN_POINT ( 'NONE',  ( 34.43765690731135720, -12.70119407716533111, -19.95187818093482335 ) ) ;
#20163=CARTESIAN_POINT ( 'NONE',  ( 22.86252235622482587, -0.9498377794471745128, -13.29674124224850118 ) ) ;
#20172=CARTESIAN_POINT ( 'NONE',  ( 27.15293434934692129, -9.258526923162836653, -12.62629486378885701 ) ) ;
#20173=CARTESIAN_POINT ( 'NONE',  ( 28.35258904315412920, -6.370284285516064848, -14.91745349193007364 ) ) ;
#20183=CARTESIAN_POINT ( 'NONE',  ( 11.22782251818125232, 9.073501160497098539, -17.23995927586370769 ) ) ;
#20185=CARTESIAN_POINT ( 'NONE',  ( 12.51417009928267099, 8.576964204390579383, -15.11888119342340353 ) ) ;
#20186=CARTESIAN_POINT ( 'NONE',  ( 27.03191753302054323, -12.88672130028117735, -14.08881772908025454 ) ) ;
#20191=CARTESIAN_POINT ( 'NONE',  ( 9.641350835837977584, 17.66889102485563612, -17.91507476468484938 ) ) ;
#20195=CARTESIAN_POINT ( 'NONE',  ( 26.72181814967143509, -3.137724904577397389, -15.69709663067708050 ) ) ;
#20199=CARTESIAN_POINT ( 'NONE',  ( 12.24513942169458858, 9.516104476910269838, -15.33330339355663519 ) ) ;
#20205=CARTESIAN_POINT ( 'NONE',  ( 24.14317479683219858, -6.286850201977149055, -18.60698471650063723 ) ) ;
#20209=CARTESIAN_POINT ( 'NONE',  ( 21.34664435287406903, -1.670712410592182895, -14.88600020661825063 ) ) ;
#20212=CARTESIAN_POINT ( 'NONE',  ( 31.01114313885700824, -11.37490951371675507, -12.31627997798639917 ) ) ;
#20213=CARTESIAN_POINT ( 'NONE',  ( 24.28706804496593463, -0.4963248009486594392, -19.74393692370418307 ) ) ;
#20215=CARTESIAN_POINT ( 'NONE',  ( 24.62590367393082502, -9.567571807129121808, -15.85044010117769098 ) ) ;
#20223=CARTESIAN_POINT ( 'NONE',  ( 27.43603605124483025, -4.716368786860208218, -15.63773258035017300 ) ) ;
#20224=CARTESIAN_POINT ( 'NONE',  ( 16.63724033897865340, 2.930722838386041751, -15.17604395537502526 ) ) ;
#20225=CARTESIAN_POINT ( 'NONE',  ( 33.34778169882233811, -10.20066162918134367, -19.85315749909214844 ) ) ;
#20227=CARTESIAN_POINT ( 'NONE',  ( 11.46877092736959014, 9.288109543210406827, -15.86260999805022820 ) ) ;
#20230=CARTESIAN_POINT ( 'NONE',  ( 9.661883060892410668, 16.25482663691947849, -17.91599866193395485 ) ) ;
#20233=CARTESIAN_POINT ( 'NONE',  ( 12.51757296969303290, 8.578467993704791184, -15.11616904564172792 ) ) ;
#20243=CARTESIAN_POINT ( 'NONE',  ( 8.944584683310379702, 16.95159276115599667, -17.92981046679734547 ) ) ;
#20244=CARTESIAN_POINT ( 'NONE',  ( 36.53927379715840829, -23.14264550581856739, -18.86160504153442830 ) ) ;
#20245=CARTESIAN_POINT ( 'NONE',  ( 15.19363621961471722, 2.181190162186355419, -17.24139079752846015 ) ) ;
#20246=CARTESIAN_POINT ( 'NONE',  ( 28.67999647541807207, -5.919990246138143952, -18.25217309140403188 ) ) ;
#20249=CARTESIAN_POINT ( 'NONE',  ( 19.78633661418711043, -4.982883274218824710, -16.00186916550291727 ) ) ;
#20259=CARTESIAN_POINT ( 'NONE',  ( 34.76605987604303749, -17.66900494105776787, -19.07908574721388462 ) ) ;
#20262=CARTESIAN_POINT ( 'NONE',  ( 10.76353862942338147, 8.717528283631100550, -16.36374602157236779 ) ) ;
#20265=CARTESIAN_POINT ( 'NONE',  ( 29.82081855766934453, -7.722587238354316597, -15.76009366473342332 ) ) ;
#20266=CARTESIAN_POINT ( 'NONE',  ( 12.97729766242475868, 9.564223303342972216, -16.02852426037668465 ) ) ;
#20271=CARTESIAN_POINT ( 'NONE',  ( 12.60945047077962933, 8.619070305187777947, -15.04294105552940231 ) ) ;
#20277=CARTESIAN_POINT ( 'NONE',  ( 9.661883061612440926, 16.25482663361732705, -19.66666666666843000 ) ) ;
#20278=CARTESIAN_POINT ( 'NONE',  ( 22.18718699900398761, -4.329393945612883599, -17.49580572735151307 ) ) ;
#20279=CARTESIAN_POINT ( 'NONE',  ( 18.26434493437671946, 4.448125397982363616, -12.89349226661579273 ) ) ;
#20284=CARTESIAN_POINT ( 'NONE',  ( 23.86551563699305234, 2.542095107771292106, -17.79649620197707094 ) ) ;
#20291=CARTESIAN_POINT ( 'NONE',  ( 32.63711423693117553, -11.05166607373017484, -18.34576405707344549 ) ) ;
#20296=CARTESIAN_POINT ( 'NONE',  ( 15.39489021548154568, 6.697694061803245447, -14.95590323207311734 ) ) ;
#20297=CARTESIAN_POINT ( 'NONE',  ( 12.24525513380350539, 9.516155168367477657, -15.33321120281095773 ) ) ;
#20298=CARTESIAN_POINT ( 'NONE',  ( 33.48796008207983022, -12.92717959506727965, -19.73506838908087246 ) ) ;
#20301=CARTESIAN_POINT ( 'NONE',  ( 9.641350810849047548, 17.66889113945805789, -17.98596209335946128 ) ) ;
#20303=CARTESIAN_POINT ( 'NONE',  ( 9.641566850259106758, 17.66790035518494051, -17.86107206016944460 ) ) ;
#20308=CARTESIAN_POINT ( 'NONE',  ( 10.35864918915110877, 16.97212501191939538, -19.66666666666842644 ) ) ;
#20309=CARTESIAN_POINT ( 'NONE',  ( 33.30032953382602301, -10.37518355935928938, -17.98954529685971337 ) ) ;
#20310=CARTESIAN_POINT ( 'NONE',  ( 19.25770813156441008, -2.543370271471735222, -15.40753146551623587 ) ) ;
#20317=CARTESIAN_POINT ( 'NONE',  ( 26.09074415779471323, -5.786596670875995940, -12.76770422508296932 ) ) ;
#20318=CARTESIAN_POINT ( 'NONE',  ( 26.04927874075684713, 0.2391533594452614209, -17.67486400872287788 ) ) ;
#20331=CARTESIAN_POINT ( 'NONE',  ( 11.20373435594124878, 9.183700057499073921, -17.24994136041982529 ) ) ;
#20332=CARTESIAN_POINT ( 'NONE',  ( 12.47535353872619446, 8.560407331872438519, -15.14977315560688176 ) ) ;
#20338=CARTESIAN_POINT ( 'NONE',  ( 9.641350810849047548, 17.66889113945805789, -17.92454625180715766 ) ) ;
#20343=CARTESIAN_POINT ( 'NONE',  ( 21.43917814492346707, -4.799604530101110988, -17.97822123721208243 ) ) ;
#20347=CARTESIAN_POINT ( 'NONE',  ( 11.05541531668977662, 17.68942339022145305, -17.91928203681695564 ) ) ;
#20349=CARTESIAN_POINT ( 'NONE',  ( 35.12509383387676820, -20.28195432802065312, -20.22992657050740917 ) ) ;
#20352=CARTESIAN_POINT ( 'NONE',  ( 26.04489551603160180, -6.130266781319400948, -13.71289979607875154 ) ) ;
#20354=CARTESIAN_POINT ( 'NONE',  ( 23.33733100364600688, 1.020658515592549609, -17.81090727445316446 ) ) ;
#20357=CARTESIAN_POINT ( 'NONE',  ( 17.27944038698359464, 10.59897317215052226, -14.78577975581568360 ) ) ;
#20358=CARTESIAN_POINT ( 'NONE',  ( 26.92475197568164802, -10.17130474311345800, -13.43658410890694732 ) ) ;
#20372=CARTESIAN_POINT ( 'NONE',  ( 25.27232213581778808, -7.536446408081735271, -18.87890555733638465 ) ) ;
#20373=CARTESIAN_POINT ( 'NONE',  ( 21.63689124574611711, 4.661388338709377521, -16.95871344450652174 ) ) ;
#20374=CARTESIAN_POINT ( 'NONE',  ( 34.01601630636088913, -11.85276864474937852, -20.84012540857256823 ) ) ;
#20376=CARTESIAN_POINT ( 'NONE',  ( 12.49899259368311988, 8.570259324921714494, -15.13097775544467005 ) ) ;
#20379=CARTESIAN_POINT ( 'NONE',  ( 9.672937757006597081, 16.20412839139380168, -17.88297960302892520 ) ) ;
#20383=CARTESIAN_POINT ( 'NONE',  ( 12.50076791318051761, 8.571041463825640250, -15.12956297801270900 ) ) ;
#20390=CARTESIAN_POINT ( 'NONE',  ( 13.37763225631166542, 7.625080029534266224, -15.70945042905673006 ) ) ;
#20391=CARTESIAN_POINT ( 'NONE',  ( 34.47915806976548936, -13.88763681628941349, -21.00674453490027460 ) ) ;
#20393=CARTESIAN_POINT ( 'NONE',  ( 21.48460829514769799, 2.948577479130256584, -19.81588663513211657 ) ) ;
#20394=CARTESIAN_POINT ( 'NONE',  ( 17.18133768520950255, 3.791981501156216350, -18.48732239789962506 ) ) ;
#20398=CARTESIAN_POINT ( 'NONE',  ( 18.73701609394335321, -1.228702115187185973, -15.37238819164404369 ) ) ;
#20411=CARTESIAN_POINT ( 'NONE',  ( 35.54859390953724585, -21.18451583373416014, -16.11276402859391510 ) ) ;
#20414=CARTESIAN_POINT ( 'NONE',  ( 10.66616952815763320, 9.056185211661334833, -16.41224021383828102 ) ) ;
#20416=CARTESIAN_POINT ( 'NONE',  ( 27.89048517759004753, -11.43816616845083445, -12.79876095355805177 ) ) ;
#20418=CARTESIAN_POINT ( 'NONE',  ( 12.87053260329167692, 9.517041913610183812, -16.11361789703515868 ) ) ;
#20429=CARTESIAN_POINT ( 'NONE',  ( 13.12595734265553205, 8.571888915454989544, -15.91003987120930319 ) ) ;
#20430=CARTESIAN_POINT ( 'NONE',  ( 20.35037346166061312, -2.402462631129500092, -18.68063351227773694 ) ) ;
#20431=CARTESIAN_POINT ( 'NONE',  ( 23.69691533927305116, -2.951365702903132604, -18.66995449711026822 ) ) ;
#20432=CARTESIAN_POINT ( 'NONE',  ( 17.70500667399921824, 3.403337836861581867, -14.36321643528369663 ) ) ;
#20436=CARTESIAN_POINT ( 'NONE',  ( 19.50856600871340873, -1.908691058934758100, -18.90332006808282728 ) ) ;
#20444=CARTESIAN_POINT ( 'NONE',  ( 10.35864917552468611, 16.97212507441191320, -17.91611982430173455 ) ) ;
#20445=CARTESIAN_POINT ( 'NONE',  ( 32.52799721746220740, -11.03300674309804386, -18.03857687357939099 ) ) ;
#20450=CARTESIAN_POINT ( 'NONE',  ( 17.95327243003904982, 7.812726124483462264, -14.88485059575767266 ) ) ;
#20451=CARTESIAN_POINT ( 'NONE',  ( 12.24938746628909492, 9.517981781931423413, -15.32991762565031202 ) ) ;
#20452=CARTESIAN_POINT ( 'NONE',  ( 35.37764311538968087, -21.41652447078215005, -19.89511094362359955 ) ) ;
#20457=CARTESIAN_POINT ( 'NONE',  ( 17.10490717348788081, 9.547663288818908356, -11.45998271326893381 ) ) ;
#20465=CARTESIAN_POINT ( 'NONE',  ( 13.14063544215093948, 9.636405190433555035, -15.89834116682275145 ) ) ;
#20466=CARTESIAN_POINT ( 'NONE',  ( 34.70514358766799745, -13.90287004036446739, -20.03273298744158737 ) ) ;
#20467=CARTESIAN_POINT ( 'NONE',  ( 23.63863231746517712, -2.790269051896475450, -19.68844555248840678 ) ) ;
#20474=CARTESIAN_POINT ( 'NONE',  ( 22.09907825138052218, -7.445301066569870230, -16.29136317631293807 ) ) ;
#20476=CARTESIAN_POINT ( 'NONE',  ( 28.68006932781580076, -6.484681432979621185, -16.07205306641353104 ) ) ;
#20486=CARTESIAN_POINT ( 'NONE',  ( 12.63667343406881294, 8.631100619704961119, -15.02124387326777111 ) ) ;
#20493=CARTESIAN_POINT ( 'NONE',  ( 9.843778300897430000, 16.74053286659246709, -16.57516421589427225 ) ) ;
#20494=CARTESIAN_POINT ( 'NONE',  ( 15.09270446591840731, 5.883488971450414162, -17.42782692652931331 ) ) ;
#20497=CARTESIAN_POINT ( 'NONE',  ( 24.00918528248616468, -0.5066965781341161712, -13.81223085940890627 ) ) ;
#20499=ORIENTED_EDGE ( 'NONE', *, *, #1169, .F. ) ;
#20501=CARTESIAN_POINT ( 'NONE',  ( 11.05541531668977662, 17.68942339022145305, -17.91752729848688830 ) ) ;
#20503=CARTESIAN_POINT ( 'NONE',  ( 31.77493940018505114, -11.56844746753418640, -13.90849911728625266 ) ) ;
#20506=CARTESIAN_POINT ( 'NONE',  ( 21.57856661146780652, -4.666631351218505586, -18.28211233923166645 ) ) ;
#20508=CARTESIAN_POINT ( 'NONE',  ( 24.07691212630517796, -1.086650970500502300, -17.53382830850624785 ) ) ;
#20512=CARTESIAN_POINT ( 'NONE',  ( 27.50131297508284334, -11.63919202702402167, -19.74788458503752864 ) ) ;
#20513=CARTESIAN_POINT ( 'NONE',  ( 30.28771073495105881, -9.259452824753982014, -16.33981616121770131 ) ) ;
#20518=( GEOMETRIC_REPRESENTATION_CONTEXT ( 3 ) GLOBAL_UNCERTAINTY_ASSIGNED_CONTEXT ( ( #14354 ) ) GLOBAL_UNIT_ASSIGNED_CONTEXT ( ( #8465, #6789, #30040 ) ) REPRESENTATION_CONTEXT ( 'NONE', 'WORKASPACE' ) );
#20523=CARTESIAN_POINT ( 'NONE',  ( 24.24519292511275737, -8.489478586693508078, -18.02380513063773648 ) ) ;
#20524=CARTESIAN_POINT ( 'NONE',  ( 17.90640022563237110, 0.6078909361919438981, -17.24624654394265377 ) ) ;
#20525=CARTESIAN_POINT ( 'NONE',  ( 35.54910479118309041, -18.69434066908399217, -21.33016376092627553 ) ) ;
#20528=CARTESIAN_POINT ( 'NONE',  ( 12.50140887008201851, 8.571324787501421127, -15.12905211845398412 ) ) ;
#20531=CARTESIAN_POINT ( 'NONE',  ( 9.668122305056073174, 16.22621266786625327, -17.88497096177859191 ) ) ;
#20535=CARTESIAN_POINT ( 'NONE',  ( 12.56861602585598980, 8.601024833420110483, -15.07548682890769243 ) ) ;
#20540=CARTESIAN_POINT ( 'NONE',  ( 13.77718166750866224, 8.859676595473322536, -15.39100258941132715 ) ) ;
#20542=CARTESIAN_POINT ( 'NONE',  ( 9.177416647856844634, 15.88379569257361190, -17.02789189981719176 ) ) ;
#20543=CARTESIAN_POINT ( 'NONE',  ( 33.31547190024930671, -13.15228156363260581, -20.72525089784059560 ) ) ;
#20546=CARTESIAN_POINT ( 'NONE',  ( 20.23665759668125474, 8.554704514664523529, -15.35188933034790182 ) ) ;
#20548=CARTESIAN_POINT ( 'NONE',  ( 16.66981565813235733, 9.362922448895053762, -13.87743608138566920 ) ) ;
#20551=CARTESIAN_POINT ( 'NONE',  ( 27.27607810006200140, -2.061267822988343656, -14.60586277656102006 ) ) ;
#20554=SURFACE_STYLE_USAGE ( .BOTH. , #13689 ) ;
#20559=CARTESIAN_POINT ( 'NONE',  ( 33.81279548071420038, -11.10283711904122050, -17.43625070980107594 ) ) ;
#20561=CARTESIAN_POINT ( 'NONE',  ( 12.49426214472998176, 7.541115143590324088, -15.13238550383361769 ) ) ;
#20565=CARTESIAN_POINT ( 'NONE',  ( 29.88803641097454999, -7.968445601786871002, -16.75847372370488131 ) ) ;
#20567=CARTESIAN_POINT ( 'NONE',  ( 10.48212431696843439, 16.40585233633115436, -17.33062619162406293 ) ) ;
#20572=CARTESIAN_POINT ( 'NONE',  ( 13.04501788334644630, 8.811555337407297017, -14.69578613943112799 ) ) ;
#20578=CARTESIAN_POINT ( 'NONE',  ( 9.661883061612440926, 16.25482663361732705, -17.92279151347708677 ) ) ;
#20580=CARTESIAN_POINT ( 'NONE',  ( 24.36273546358933828, 1.710929640254579720, -17.54733717687237160 ) ) ;
#20581=CARTESIAN_POINT ( 'NONE',  ( 22.87531825017061848, 1.851759407679815173, -13.77476424085121742 ) ) ;
#20584=CARTESIAN_POINT ( 'NONE',  ( 20.55949567978923298, 1.660703385868308235, -14.27713627412184039 ) ) ;
#20588=CARTESIAN_POINT ( 'NONE',  ( 23.16390915794477223, 2.882539813099532555, -14.99485278278146438 ) ) ;
#20593=CARTESIAN_POINT ( 'NONE',  ( 10.36007019289729847, 16.96560810760319882, -17.82599398985513872 ) ) ;
#20599=CARTESIAN_POINT ( 'NONE',  ( 19.51440197245297270, 8.071880087464508691, -17.28625796899888201 ) ) ;
#20600=CARTESIAN_POINT ( 'NONE',  ( 11.53546837550287130, 15.48783886997274450, -16.67730506581143501 ) ) ;
#20601=CARTESIAN_POINT ( 'NONE',  ( 35.54859390953724585, -22.18451583373416014, -16.94733705004010460 ) ) ;
#20605=CARTESIAN_POINT ( 'NONE',  ( 9.641404825192898542, 17.66864342279195199, -17.88841768828662282 ) ) ;
#20611=CARTESIAN_POINT ( 'NONE',  ( 12.87180867969543385, 9.517605834602926862, -16.11260084161717998 ) ) ;
#20612=CARTESIAN_POINT ( 'NONE',  ( 35.77509030908504428, -18.70957389315904962, -20.35615221346758474 ) ) ;
#20613=CARTESIAN_POINT ( 'NONE',  ( 23.84106988684860440, -4.080291168153947545, -13.50610408985603250 ) ) ;
#20625=CARTESIAN_POINT ( 'NONE',  ( 24.97892660363778106, -6.291154998746494087, -12.74939059104742256 ) ) ;
#20626=CARTESIAN_POINT ( 'NONE',  ( 28.66609726738115071, -6.663921799113727396, -16.65640135049372006 ) ) ;
#20633=CARTESIAN_POINT ( 'NONE',  ( 14.38576730248667701, 9.404056492746565965, -13.62718518646353161 ) ) ;
#20634=CARTESIAN_POINT ( 'NONE',  ( 30.76698452600511402, -8.440788201038053273, -16.67119366161266925 ) ) ;
#20637=CARTESIAN_POINT ( 'NONE',  ( 9.641485839925177714, 17.66827187890266160, -17.87200850766020110 ) ) ;
#20638=CARTESIAN_POINT ( 'NONE',  ( 15.41580380672748163, 5.935325531760808460, -16.22756139702874023 ) ) ;
#20641=CARTESIAN_POINT ( 'NONE',  ( 24.95482030053459965, -6.624749414579512496, -13.76522253407564733 ) ) ;
#20644=CARTESIAN_POINT ( 'NONE',  ( 12.25660130062383146, 9.517454774955181662, -15.32445140518387028 ) ) ;
#20645=CARTESIAN_POINT ( 'NONE',  ( 35.54859569580823830, -22.18452385850428499, -18.27063337037174762 ) ) ;
#20646=CARTESIAN_POINT ( 'NONE',  ( 15.87806330829146617, 7.947701475055697351, -19.83831759000646855 ) ) ;
#20648=CARTESIAN_POINT ( 'NONE',  ( 26.47492910780048447, -3.130564378024159211, -15.09640780237150892 ) ) ;
#20650=CARTESIAN_POINT ( 'NONE',  ( 21.43024726678804726, -3.720057188146618010, -16.74626013867020902 ) ) ;
#20655=( BOUNDED_SURFACE ( )  B_SPLINE_SURFACE ( 3, 3, ( 
 ( #20952, #16683, #64, #9348, #11344, #28334, #28019, #11791, #16375, #4786, #9494, #14076, #23405, #5085, #21257, #14373, #2522, #9655, #7388, #23711, #20646, #30033, #9041, #27721, #19710, #26309, #21565, #12097, #664, #3266, #9949, #810, #12393, #17134, #7969, #26461, #21860, #5392, #23870, #28476, #7524, #21705, #14973, #19565, #28933, #17277, #26613, #17423, #14528, #12541, #12247, #19262, #28784, #5541, #5694, #2971, #14826, #24161, #28620, #24309, #3405, #7675, #12697, #3121, #10253, #22017, #1125, #19120, #26160, #10102, #19415, #16983, #7827, #10403, #29076, #970, #24021, #14678, #2813, #8118, #26772, #5842, #15129, #21413, #519, #9808, #16828, #5234, #22620, #18180, #8564, #8713, #24608, #29390, #8416, #26929, #5988, #18028, #11162, #17721, #13001, #3554, #22313, #24922, #1422, #22476, #3854, #17864, #29699, #27240, #13301, #27080, #15276, #19864, #29228, #13151, #6447, #11006, #20310, #27395, #15736, #8862, #3700, #4002, #10711, #20022, #20163, #6290, #25063, #6139, #15586, #1721, #15435, #4150, #13447, #24765, #22775, #1573, #1881, #20467, #29857, #10555, #17574, #10852, #29545, #27538, #6592, #24458, #12846, #22158, #1268, #8264, #18938, #20613, #18326, #30001, #16338, #6904, #18786, #13748, #9317, #9006, #27684, #28294, #23217, #23520, #23076, #16193, #4898, #21220, #25656, #28140, #4748, #14194, #30148, #27840, #4602, #16036, #6744, #11451, #335, #11310, #25361, #2629, #4457, #2175, #9620, #7047, #25817, #25511, #20760, #25215, #4303, #13602, #21075, #11904, #183, #14039, #22930, #11759, #9155, #20915, #13890, #15882, #2032, #11601, #29, #18484, #2332, #23368, #9462, #18641, #27987, #7197, #2484, #16491, #481, #23832, #12661, #2930, #9916, #19379, #14495, #9770, #21668, #19227, #28901, #14940, #5201, #7638, #12504, #19088, #28439, #21979, #12210, #21530, #1092, #16796, #631, #26574, #19674, #28584, #28743, #770, #21373, #24275 ),
 ( #17098, #5047, #3226, #7491, #12355, #16945, #10369, #26274, #26123, #7348, #3374, #5356, #7789, #10067, #14642, #26423, #23989, #3086, #16649, #5503, #25966, #14788, #21827, #24128, #927, #10219, #19530, #7932, #17243, #14338, #5658, #23674, #2778, #12060, #29512, #26895, #27049, #8384, #13114, #3972, #22440, #17834, #1387, #19829, #24426, #3521, #17690, #10970, #15552, #24887, #13271, #22588, #13414, #10515, #8533, #8229, #15247, #24732, #1540, #1689, #29192, #10823, #20134, #5959, #20279, #29666, #17539, #8681, #29358, #6257, #17987, #27359, #15090, #22127, #6104, #15398, #24579, #3820, #3667, #27206, #6415, #15704, #12963, #25033, #4119, #22278, #22739, #1852, #10678, #11130, #29039, #8079, #17388, #26733, #12814, #1231, #5805, #19987, #20581, #2143, #30259, #9271, #25471, #11417, #13998, #21035, #15848, #4269, #25178, #4562, #4421, #18599, #29966, #18450, #13569, #6557, #141, #20722, #4705, #8973, #13715, #16296, #23327, #13851, #27950, #23177, #25609, #6713, #25330, #30109, #1997, #22895, #18288, #2440, #11276, #27645, #11718, #16001, #23041, #20431, #2289, #29823, #9119, #27799, #18144, #27506, #6866, #7007, #8831, #16153, #11560, #20877, #13357, #17634, #22537, #27138, #22833, #8477, #26989, #17485, #25119, #8331, #17925, #1635, #17778, #27301, #3913, #13056, #1938, #15648, #11220, #10914, #1783, #6047, #22379, #1484, #19928, #29294, #11068, #4209, #10774, #15336, #26834, #24673, #6355, #3763, #15494, #6201, #20223, #22682, #29609, #24981, #20083, #29459, #12904, #22218, #24825, #29762, #4064, #20372, #8771, #18086, #20523, #13213, #27448, #8625, #6501, #15792, #13506, #29910, #5905, #15187, #24519, #3612, #1327, #10618, #9534, #9847, #23754, #4820, #28220, #17025, #28061, #14117, #704, #23447, #18858, #26351, #2851, #12286, #2695, #2559, #11679, #20994, #104, #7565, #9989, #16871, #12137, #9387, #28517, #11832, #7425, #11978, #7716, #23598 ),
 ( #18713, #5430, #4973, #28667, #21145, #21298, #9690, #256, #26200, #3009, #5278, #21454, #26046, #23915, #7270, #7114, #14565, #16573, #562, #19160, #16418, #21606, #19305, #25737, #25896, #14264, #14717, #405, #16725, #19015, #2404, #28370, #5123, #14414, #8310, #13043, #29437, #29119, #29274, #21751, #10295, #3593, #17466, #22359, #7863, #1464, #24649, #19603, #22059, #19456, #17615, #28826, #26975, #19910, #6032, #6181, #15317, #24505, #17173, #10755, #5736, #3308, #26502, #8460, #19750, #8160, #17764, #27119, #12885, #3743, #24349, #24059, #20062, #26814, #28973, #5583, #8010, #3160, #17316, #26657, #5889, #15170, #14865, #12432, #854, #10144, #12584, #21903, #10442, #1311, #24205, #1018, #15019, #3449, #12738, #1161, #22199, #10599, #13339, #4492, #9044, #22815, #27574, #18367, #20354, #20802, #13783, #22517, #30187, #18069, #11487, #6334, #25100, #1919, #4043, #30037, #16073, #11347, #25255, #8901, #6786, #15629, #20209, #27723, #22662, #4339, #22966, #29587, #23110, #13637, #8605, #24963, #1766, #2216, #17905, #20508, #27284, #25401, #11052, #9197, #1617, #18524, #27880, #15476, #29893, #20650, #13195, #29744, #2068, #18218, #24809, #8750, #3896, #10895, #27430, #13488, #6485, #15774, #4190, #11197, #6629, #15922, #19266, #21417, #7391, #20955, #26163, #18820, #16377, #68, #21568, #2661, #21259, #666, #9951, #26010, #12100, #7237, #6937, #523, #11940, #2525, #9351, #23407, #12250, #11796, #9498, #18979, #14078, #18676, #371, #28179, #28481, #14531, #4788, #16535, #9811, #4637, #28024, #5090, #25543, #21113, #16230, #25699, #219, #5239, #13927, #25859, #14377, #28337, #7082, #4937, #23259, #2370, #14229, #23874, #23563, #9658, #11643, #16687, #16834, #23714, #2817, #19124, #7527, #2974, #3558, #5993, #12850, #8122, #26311, #24462, #28786, #3409, #7973, #3705, #19569, #7830, #28624, #15280, #19418, #29082, #12700, #28937, #17427, #14978 ),
 ( #29233, #22163, #26775, #22021, #19868, #17138, #3123, #10561, #5548, #5845, #15133, #12396, #17578, #1272, #21708, #26466, #14829, #26936, #812, #1128, #10108, #8268, #24167, #24612, #14682, #13003, #22320, #1853, #10407, #11131, #5395, #3269, #7679, #19713, #16985, #12545, #24025, #21865, #973, #26617, #10256, #17281, #5697, #24313, #16298, #25613, #2591, #4707, #20878, #4271, #9421, #2146, #29967, #13571, #4855, #16154, #4564, #14156, #23484, #9272, #13999, #20724, #20432, #23328, #25473, #16002, #22896, #6714, #25777, #25331, #23043, #2290, #27646, #1998, #13855, #11418, #11719, #28094, #18289, #30111, #2442, #18146, #11277, #25179, #18747, #6559, #21037, #7158, #29825, #23178, #143, #27507, #4422, #30261, #11562, #16454, #20584, #8834, #15849, #13716, #18451, #8974, #9120, #27800, #6867, #18601, #27951, #7008, #26390, #12317, #25930, #893, #23793, #21335, #5012, #26540, #7600, #26236, #5620, #14900, #730, #14301, #23636, #21633, #2891, #14754, #9727, #5316, #16609, #2734, #24241, #19192, #19495, #19049, #12173, #10184, #17212, #10027, #24092, #19341, #28866, #7901, #28405, #28705, #3045, #12017, #7458, #11867, #7304, #443, #21180, #16762, #26084, #291, #7753, #21793, #21491, #5164, #9574, #18899, #28254, #17062, #14454, #5469, #3193, #595, #12470, #9880, #16905, #28548, #14600, #23955, #3489, #3342, #10936, #24390, #3786, #8352, #24544, #13081, #19951, #29154, #17949, #1508, #27326, #17655, #17800, #12777, #8195, #17505, #5773, #15054, #27163, #20246, #26859, #22094, #12624, #1199, #22403, #10481, #1352, #12924, #27016, #8501, #6071, #10796, #5926, #19789, #29007, #8044, #15211, #22559, #6222, #10641, #15357, #15519, #3631, #8645, #1658, #10332, #6381, #22243, #29633, #29320, #24696, #20103, #29482, #24850, #3937, #13239, #15670, #21943, #1056, #19640, #17353, #26698, #1960, #4530, #2257, #8797, #13966, #13821, #29784, #25141, #11242, #23296 ),
 ( #11529, #20842, #9391, #6525, #25439, #4233, #20548, #20691, #9089, #9234, #13532, #18413, #27765, #29934, #30225, #18566, #22858, #27917, #25295, #6976, #16264, #2410, #11092, #18109, #4383, #2112, #8941, #23007, #25579, #4675, #23146, #15966, #18717, #11684, #13683, #27471, #15815, #21001, #11386, #109, #18257, #6830, #27613, #6675, #7122, #30077, #28065, #16120, #25003, #4086, #13379, #22705, #1811, #20394, #5439, #3165, #23603, #23921, #7570, #18866, #11983, #859, #11837, #28224, #14722, #7275, #2699, #10149, #16876, #26356, #16730, #16577, #25742, #4826, #14122, #21610, #24064, #708, #26204, #23454, #12291, #25902, #21458, #26051, #21759, #21302, #14419, #21149, #9994, #260, #19311, #28672, #7720, #28830, #17030, #5282, #9539, #12436, #28377, #4978, #14269, #19462, #12145, #568, #5130, #16423, #19164, #9852, #23758, #2563, #412, #28521, #9695, #19020, #7429, #2855, #14570, #3015, #19916, #15023, #10302, #22206, #10449, #29444, #15483, #5740, #8164, #13047, #5589, #1023, #26980, #26507, #22064, #13201, #17322, #24355, #27125, #20213, #29125, #29279, #1316, #21909, #24813, #14870, #22366, #26663, #3453, #24510, #15323, #7869, #10759, #12745, #1165, #8467, #17769, #6187, #17181, #19755, #3902, #1469, #15175, #8315, #20067, #17470, #22524, #1622, #24211, #10900, #26820, #3312, #28980, #5893, #3597, #12890, #12589, #19609, #3750, #17620, #10606, #8014, #6038, #24655, #11493, #6489, #9048, #6791, #13343, #18531, #18373, #4049, #29749, #15779, #27885, #1771, #4344, #11057, #20807, #22667, #6942, #15636, #13788, #16234, #4642, #13643, #4497, #27290, #25104, #27729, #22971, #25548, #20358, #13933, #30192, #16080, #6339, #25405, #8758, #2075, #8908, #23265, #20513, #18074, #29594, #2374, #27436, #30042, #11352, #29898, #23114, #15927, #4194, #11647, #2223, #8611, #20657, #9201, #13493, #22821, #1924, #11203, #18224, #17910, #24970, #27578, #6633, #25259 ),
 ( #14382, #9816, #23567, #11800, #16382, #25708, #377, #2980, #7534, #16838, #26168, #5244, #5401, #2529, #21421, #224, #7243, #16693, #5094, #14536, #21117, #23719, #2822, #28186, #23881, #12256, #9502, #21573, #21263, #28485, #671, #19273, #7087, #14082, #9663, #28342, #18826, #18986, #9956, #28628, #531, #11944, #14687, #7684, #7395, #23413, #4792, #19128, #26017, #16991, #16540, #12107, #25864, #4942, #3127, #26316, #24031, #14234, #20962, #74, #9355, #18681, #28029, #2665, #1430, #29404, #19575, #19873, #3564, #14833, #7978, #27087, #7834, #24171, #10718, #3273, #28942, #6148, #12855, #22327, #12705, #12551, #21713, #818, #10113, #17586, #20029, #26941, #19718, #24468, #15285, #17288, #17728, #8427, #19424, #15444, #14984, #24774, #21871, #22026, #29089, #980, #5997, #13007, #8273, #22169, #5851, #3712, #10262, #17143, #24616, #26623, #1276, #29238, #26471, #12400, #10568, #5555, #5701, #24321, #28790, #3414, #17431, #1132, #10413, #8127, #26781, #15138, #18333, #23083, #9166, #8873, #9011, #1583, #20318, #13607, #27544, #2187, #17870, #11455, #4462, #29708, #1889, #29554, #27694, #8571, #6753, #30005, #16043, #16200, #25369, #4309, #27250, #20766, #15743, #13307, #6298, #18493, #29863, #18187, #4157, #3865, #6597, #15892, #13453, #27848, #13753, #25223, #8720, #15596, #18034, #6909, #27402, #6452, #22938, #11014, #24929, #2039, #25068, #30155, #13159, #1731, #22781, #22483, #10864, #4009, #11314, #20173, #11169, #22629, #20476, #20626, #14501, #7649, #16499, #7356, #9625, #9323, #2936, #2338, #493, #14046, #4755, #11909, #2784, #25517, #28446, #23374, #190, #16801, #26132, #5209, #4608, #2496, #23840, #19093, #5055, #18948, #12222, #25667, #39, #7501, #11766, #14344, #12066, #18648, #21536, #23681, #27994, #21083, #9470, #637, #7054, #341, #16343, #9924, #18792, #19237, #11609, #9779, #28594, #13899, #28300, #23224, #20925, #28148 ),
 ( #7206, #25824, #4905, #14204, #23529, #21382, #2634, #21226, #16655, #25977, #17253, #24284, #5516, #14946, #10526, #19834, #26739, #7939, #1392, #17548, #26582, #19386, #780, #17393, #5665, #29197, #14796, #10376, #21676, #10072, #29366, #3380, #24583, #24135, #12669, #5963, #22285, #5816, #8234, #15099, #15252, #3672, #3235, #24434, #8086, #28755, #12514, #10683, #12364, #7799, #12970, #17106, #21834, #19993, #3526, #26903, #21988, #26431, #26281, #5365, #14649, #22132, #16952, #1238, #12819, #23999, #3094, #940, #1099, #19682, #10226, #29049, #19540, #28908, #16008, #29519, #8839, #13417, #29671, #18149, #25037, #3977, #23046, #6564, #2150, #22745, #22900, #8537, #13274, #22593, #1693, #6421, #3827, #2001, #13120, #11282, #4275, #13574, #20728, #20588, #27510, #22445, #27654, #20284, #17839, #1547, #11422, #4125, #1857, #8684, #8389, #11135, #20436, #17993, #17693, #29970, #29828, #10977, #10829, #24892, #13720, #27366, #15708, #15855, #15558, #20138, #25185, #8978, #18294, #25335, #6262, #6717, #4425, #6109, #27212, #27054, #15404, #24737, #5590, #9278, #16303, #19465, #12595, #21043, #11871, #14161, #13861, #7873, #6871, #5016, #18605, #27955, #16458, #7310, #30117, #2738, #7012, #4713, #21339, #448, #9733, #9127, #25620, #28831, #23641, #7165, #21185, #12023, #14003, #14871, #17183, #16159, #24214, #2450, #26510, #20884, #9425, #25781, #23332, #14306, #3313, #25935, #9580, #23488, #18455, #21918, #4568, #27807, #11723, #18905, #16613, #23182, #25478, #28258, #2296, #147, #18752, #11566, #28099, #4861, #2597, #296, #26666, #10908, #8017, #6192, #20215, #27292, #26981, #27128, #19613, #8165, #1473, #15325, #29599, #5743, #8614, #22527, #6345, #10762, #3905, #20069, #17915, #15639, #29127, #29451, #13048, #24362, #17472, #24972, #17323, #3456, #4053, #12746, #26822, #21911, #22369, #1625, #22209, #22066, #1025, #10303, #28983, #15485, #15025, #24816 ) ),
 .UNSPECIFIED., .T., .F., .F. ) 
 B_SPLINE_SURFACE_WITH_KNOTS ( ( 4, 3, 4 ),
 ( 4, 2, 2, 2, 2, 2, 2, 2, 2, 2, 2, 2, 2, 2, 2, 2, 2, 2, 2, 2, 2, 2, 2, 2, 2, 2, 2, 2, 2, 2, 2, 2, 2, 2, 2, 2, 2, 2, 2, 2, 2, 2, 2, 2, 2, 2, 2, 2, 2, 2, 2, 2, 2, 2, 2, 2, 2, 2, 2, 2, 2, 2, 2, 2, 2, 2, 2, 2, 2, 2, 2, 2, 2, 2, 2, 2, 2, 2, 2, 2, 2, 2, 2, 2, 2, 2, 2, 2, 2, 2, 2, 2, 2, 2, 2, 2, 2, 2, 2, 2, 2, 2, 2, 2, 2, 2, 2, 2, 2, 2, 2, 2, 2, 2, 2, 2, 2, 2, 2, 2, 2, 2, 4 ),
 ( 0.000000000000000000, 0.5000000000000000000, 1.000000000000000000 ),
 ( 0.000000000000000000, 0.007812500000000000000, 0.01464843750000000000, 0.02148437500000000000, 0.02832031250000000000, 0.03515625000000000000, 0.04882812500000000000, 0.05566406250000000000, 0.06250000000000000000, 0.06933593750000000000, 0.07617187500000000000, 0.08984375000000000000, 0.09667968750000000000, 0.1035156250000000000, 0.1103515625000000000, 0.1171875000000000000, 0.1240234375000000000, 0.1308593750000000000, 0.1376953125000000000, 0.1445312500000000000, 0.1513671875000000000, 0.1582031250000000000, 0.1718750000000000000, 0.1787109375000000000, 0.1855468750000000000, 0.1992187500000000000, 0.2060546875000000000, 0.2128906250000000000, 0.2197265625000000000, 0.2265625000000000000, 0.2402343750000000000, 0.2470703125000000000, 0.2539062500000000000, 0.2607421875000000000, 0.2675781250000000000, 0.2812500000000000000, 0.2880859375000000000, 0.2949218750000000000, 0.3017578125000000000, 0.3085937500000000000, 0.3154296875000000000, 0.3222656250000000000, 0.3291015625000000000, 0.3359375000000000000, 0.3496093750000000000, 0.3564453125000000000, 0.3632812500000000000, 0.3701171875000000000, 0.3769531250000000000, 0.3906250000000000000, 0.3974609375000000000, 0.4042968750000000000, 0.4179687500000000000, 0.4316406250000000000, 0.4384765625000000000, 0.4453125000000000000, 0.4521484375000000000, 0.4589843750000000000, 0.4658203125000000000, 0.4726562500000000000, 0.4794921875000000000, 0.4863281250000000000, 0.4931640625000000000, 0.5000000000000000000, 0.5078125000000000000, 0.5156250000000000000, 0.5234375000000000000, 0.5312500000000000000, 0.5390625000000000000, 0.5468750000000000000, 0.5625000000000000000, 0.5693359375000000000, 0.5761718750000000000, 0.5898437500000000000, 0.5966796875000000000, 0.6035156250000000000, 0.6103515625000000000, 0.6171875000000000000, 0.6308593750000000000, 0.6376953125000000000, 0.6445312500000000000, 0.6513671875000000000, 0.6582031250000000000, 0.6718750000000000000, 0.6787109375000000000, 0.6855468750000000000, 0.6992187500000000000, 0.7128906250000000000, 0.7197265625000000000, 0.7265625000000000000, 0.7333984375000000000, 0.7402343750000000000, 0.7470703125000000000, 0.7539062500000000000, 0.7607421875000000000, 0.7675781250000000000, 0.7744140625000000000, 0.7812500000000000000, 0.7890625000000000000, 0.7968750000000000000, 0.8046875000000000000, 0.8125000000000000000, 0.8203125000000000000, 0.8281250000000000000, 0.8437500000000000000, 0.8505859375000000000, 0.8574218750000000000, 0.8710937500000000000, 0.8779296875000000000, 0.8847656250000000000, 0.8916015625000000000, 0.8984375000000000000, 0.9121093750000000000, 0.9189453125000000000, 0.9257812500000000000, 0.9326171875000000000, 0.9394531250000000000, 0.9531250000000000000, 0.9589843750000000000, 0.9648437500000000000, 0.9765625000000000000, 0.9882812500000000000, 1.000000000000000000 ),
 .UNSPECIFIED. ) 
 GEOMETRIC_REPRESENTATION_ITEM ( )  RATIONAL_B_SPLINE_SURFACE ( (
 ( 1.000000000000000000, 1.000000000000000000, 1.000000000000000000, 1.000000000000000000, 1.000000000000000000, 1.000000000000000000, 1.000000000000000000, 1.000000000000000000, 1.000000000000000000, 1.000000000000000000, 1.000000000000000000, 1.000000000000000000, 1.000000000000000000, 1.000000000000000000, 1.000000000000000000, 1.000000000000000000, 1.000000000000000000, 1.000000000000000000, 1.000000000000000000, 1.000000000000000000, 1.000000000000000000, 1.000000000000000000, 1.000000000000000000, 1.000000000000000000, 1.000000000000000000, 1.000000000000000000, 1.000000000000000000, 1.000000000000000000, 1.000000000000000000, 1.000000000000000000, 1.000000000000000000, 1.000000000000000000, 1.000000000000000000, 1.000000000000000000, 1.000000000000000000, 1.000000000000000000, 1.000000000000000000, 1.000000000000000000, 1.000000000000000000, 1.000000000000000000, 1.000000000000000000, 1.000000000000000000, 1.000000000000000000, 1.000000000000000000, 1.000000000000000000, 1.000000000000000000, 1.000000000000000000, 1.000000000000000000, 1.000000000000000000, 1.000000000000000000, 1.000000000000000000, 1.000000000000000000, 1.000000000000000000, 1.000000000000000000, 1.000000000000000000, 1.000000000000000000, 1.000000000000000000, 1.000000000000000000, 1.000000000000000000, 1.000000000000000000, 1.000000000000000000, 1.000000000000000000, 1.000000000000000000, 1.000000000000000000, 1.000000000000000000, 1.000000000000000000, 1.000000000000000000, 1.000000000000000000, 1.000000000000000000, 1.000000000000000000, 1.000000000000000000, 1.000000000000000000, 1.000000000000000000, 1.000000000000000000, 1.000000000000000000, 1.000000000000000000, 1.000000000000000000, 1.000000000000000000, 1.000000000000000000, 1.000000000000000000, 1.000000000000000000, 1.000000000000000000, 1.000000000000000000, 1.000000000000000000, 1.000000000000000000, 1.000000000000000000, 1.000000000000000000, 1.000000000000000000, 1.000000000000000000, 1.000000000000000000, 1.000000000000000000, 1.000000000000000000, 1.000000000000000000, 1.000000000000000000, 1.000000000000000000, 1.000000000000000000, 1.000000000000000000, 1.000000000000000000, 1.000000000000000000, 1.000000000000000000, 1.000000000000000000, 1.000000000000000000, 1.000000000000000000, 1.000000000000000000, 1.000000000000000000, 1.000000000000000000, 1.000000000000000000, 1.000000000000000000, 1.000000000000000000, 1.000000000000000000, 1.000000000000000000, 1.000000000000000000, 1.000000000000000000, 1.000000000000000000, 1.000000000000000000, 1.000000000000000000, 1.000000000000000000, 1.000000000000000000, 1.000000000000000000, 1.000000000000000000, 1.000000000000000000, 1.000000000000000000, 1.000000000000000000, 1.000000000000000000, 1.000000000000000000, 1.000000000000000000, 1.000000000000000000, 1.000000000000000000, 1.000000000000000000, 1.000000000000000000, 1.000000000000000000, 1.000000000000000000, 1.000000000000000000, 1.000000000000000000, 1.000000000000000000, 1.000000000000000000, 1.000000000000000000, 1.000000000000000000, 1.000000000000000000, 1.000000000000000000, 1.000000000000000000, 1.000000000000000000, 1.000000000000000000, 1.000000000000000000, 1.000000000000000000, 1.000000000000000000, 1.000000000000000000, 1.000000000000000000, 1.000000000000000000, 1.000000000000000000, 1.000000000000000000, 1.000000000000000000, 1.000000000000000000, 1.000000000000000000, 1.000000000000000000, 1.000000000000000000, 1.000000000000000000, 1.000000000000000000, 1.000000000000000000, 1.000000000000000000, 1.000000000000000000, 1.000000000000000000, 1.000000000000000000, 1.000000000000000000, 1.000000000000000000, 1.000000000000000000, 1.000000000000000000, 1.000000000000000000, 1.000000000000000000, 1.000000000000000000, 1.000000000000000000, 1.000000000000000000, 1.000000000000000000, 1.000000000000000000, 1.000000000000000000, 1.000000000000000000, 1.000000000000000000, 1.000000000000000000, 1.000000000000000000, 1.000000000000000000, 1.000000000000000000, 1.000000000000000000, 1.000000000000000000, 1.000000000000000000, 1.000000000000000000, 1.000000000000000000, 1.000000000000000000, 1.000000000000000000, 1.000000000000000000, 1.000000000000000000, 1.000000000000000000, 1.000000000000000000, 1.000000000000000000, 1.000000000000000000, 1.000000000000000000, 1.000000000000000000, 1.000000000000000000, 1.000000000000000000, 1.000000000000000000, 1.000000000000000000, 1.000000000000000000, 1.000000000000000000, 1.000000000000000000, 1.000000000000000000, 1.000000000000000000, 1.000000000000000000, 1.000000000000000000, 1.000000000000000000, 1.000000000000000000, 1.000000000000000000, 1.000000000000000000, 1.000000000000000000, 1.000000000000000000, 1.000000000000000000, 1.000000000000000000, 1.000000000000000000, 1.000000000000000000, 1.000000000000000000, 1.000000000000000000, 1.000000000000000000, 1.000000000000000000, 1.000000000000000000, 1.000000000000000000, 1.000000000000000000, 1.000000000000000000, 1.000000000000000000, 1.000000000000000000, 1.000000000000000000, 1.000000000000000000, 1.000000000000000000, 1.000000000000000000, 1.000000000000000000, 1.000000000000000000, 1.000000000000000000, 1.000000000000000000, 1.000000000000000000, 1.000000000000000000, 1.000000000000000000, 1.000000000000000000, 1.000000000000000000, 1.000000000000000000, 1.000000000000000000, 1.000000000000000000, 1.000000000000000000, 1.000000000000000000, 1.000000000000000000),
 ( 0.3333333333333333703, 0.3333333333333333703, 0.3333333333333333703, 0.3333333333333333703, 0.3333333333333333703, 0.3333333333333333703, 0.3333333333333333703, 0.3333333333333333703, 0.3333333333333333703, 0.3333333333333333703, 0.3333333333333333703, 0.3333333333333333703, 0.3333333333333333703, 0.3333333333333333703, 0.3333333333333333703, 0.3333333333333333703, 0.3333333333333333703, 0.3333333333333333703, 0.3333333333333333703, 0.3333333333333333703, 0.3333333333333333703, 0.3333333333333333703, 0.3333333333333333703, 0.3333333333333333703, 0.3333333333333333703, 0.3333333333333333703, 0.3333333333333333703, 0.3333333333333333703, 0.3333333333333333703, 0.3333333333333333703, 0.3333333333333333703, 0.3333333333333333703, 0.3333333333333333703, 0.3333333333333333703, 0.3333333333333333703, 0.3333333333333333703, 0.3333333333333333703, 0.3333333333333333703, 0.3333333333333333703, 0.3333333333333333703, 0.3333333333333333703, 0.3333333333333333703, 0.3333333333333333703, 0.3333333333333333703, 0.3333333333333333703, 0.3333333333333333703, 0.3333333333333333703, 0.3333333333333333703, 0.3333333333333333703, 0.3333333333333333703, 0.3333333333333333703, 0.3333333333333333703, 0.3333333333333333703, 0.3333333333333333703, 0.3333333333333333703, 0.3333333333333333703, 0.3333333333333333703, 0.3333333333333333703, 0.3333333333333333703, 0.3333333333333333703, 0.3333333333333333703, 0.3333333333333333703, 0.3333333333333333703, 0.3333333333333333703, 0.3333333333333333703, 0.3333333333333333703, 0.3333333333333333703, 0.3333333333333333703, 0.3333333333333333703, 0.3333333333333333703, 0.3333333333333333703, 0.3333333333333333703, 0.3333333333333333703, 0.3333333333333333703, 0.3333333333333333703, 0.3333333333333333703, 0.3333333333333333703, 0.3333333333333333703, 0.3333333333333333703, 0.3333333333333333703, 0.3333333333333333703, 0.3333333333333333703, 0.3333333333333333703, 0.3333333333333333703, 0.3333333333333333703, 0.3333333333333333703, 0.3333333333333333703, 0.3333333333333333703, 0.3333333333333333703, 0.3333333333333333703, 0.3333333333333333703, 0.3333333333333333703, 0.3333333333333333703, 0.3333333333333333703, 0.3333333333333333703, 0.3333333333333333703, 0.3333333333333333703, 0.3333333333333333703, 0.3333333333333333703, 0.3333333333333333703, 0.3333333333333333703, 0.3333333333333333703, 0.3333333333333333703, 0.3333333333333333703, 0.3333333333333333703, 0.3333333333333333703, 0.3333333333333333703, 0.3333333333333333703, 0.3333333333333333703, 0.3333333333333333703, 0.3333333333333333703, 0.3333333333333333703, 0.3333333333333333703, 0.3333333333333333703, 0.3333333333333333703, 0.3333333333333333703, 0.3333333333333333703, 0.3333333333333333703, 0.3333333333333333703, 0.3333333333333333703, 0.3333333333333333703, 0.3333333333333333703, 0.3333333333333333703, 0.3333333333333333703, 0.3333333333333333703, 0.3333333333333333703, 0.3333333333333333703, 0.3333333333333333703, 0.3333333333333333703, 0.3333333333333333703, 0.3333333333333333703, 0.3333333333333333703, 0.3333333333333333703, 0.3333333333333333703, 0.3333333333333333703, 0.3333333333333333703, 0.3333333333333333703, 0.3333333333333333703, 0.3333333333333333703, 0.3333333333333333703, 0.3333333333333333703, 0.3333333333333333703, 0.3333333333333333703, 0.3333333333333333703, 0.3333333333333333703, 0.3333333333333333703, 0.3333333333333333703, 0.3333333333333333703, 0.3333333333333333703, 0.3333333333333333703, 0.3333333333333333703, 0.3333333333333333703, 0.3333333333333333703, 0.3333333333333333703, 0.3333333333333333703, 0.3333333333333333703, 0.3333333333333333703, 0.3333333333333333703, 0.3333333333333333703, 0.3333333333333333703, 0.3333333333333333703, 0.3333333333333333703, 0.3333333333333333703, 0.3333333333333333703, 0.3333333333333333703, 0.3333333333333333703, 0.3333333333333333703, 0.3333333333333333703, 0.3333333333333333703, 0.3333333333333333703, 0.3333333333333333703, 0.3333333333333333703, 0.3333333333333333703, 0.3333333333333333703, 0.3333333333333333703, 0.3333333333333333703, 0.3333333333333333703, 0.3333333333333333703, 0.3333333333333333703, 0.3333333333333333703, 0.3333333333333333703, 0.3333333333333333703, 0.3333333333333333703, 0.3333333333333333703, 0.3333333333333333703, 0.3333333333333333703, 0.3333333333333333703, 0.3333333333333333703, 0.3333333333333333703, 0.3333333333333333703, 0.3333333333333333703, 0.3333333333333333703, 0.3333333333333333703, 0.3333333333333333703, 0.3333333333333333703, 0.3333333333333333703, 0.3333333333333333703, 0.3333333333333333703, 0.3333333333333333703, 0.3333333333333333703, 0.3333333333333333703, 0.3333333333333333703, 0.3333333333333333703, 0.3333333333333333703, 0.3333333333333333703, 0.3333333333333333703, 0.3333333333333333703, 0.3333333333333333703, 0.3333333333333333703, 0.3333333333333333703, 0.3333333333333333703, 0.3333333333333333703, 0.3333333333333333703, 0.3333333333333333703, 0.3333333333333333703, 0.3333333333333333703, 0.3333333333333333703, 0.3333333333333333703, 0.3333333333333333703, 0.3333333333333333703, 0.3333333333333333703, 0.3333333333333333703, 0.3333333333333333703, 0.3333333333333333703, 0.3333333333333333703, 0.3333333333333333703, 0.3333333333333333703, 0.3333333333333333703, 0.3333333333333333703, 0.3333333333333333703, 0.3333333333333333703, 0.3333333333333333703, 0.3333333333333333703, 0.3333333333333333703, 0.3333333333333333703, 0.3333333333333333703, 0.3333333333333333703, 0.3333333333333333703, 0.3333333333333333703, 0.3333333333333333703, 0.3333333333333333703, 0.3333333333333333703, 0.3333333333333333703, 0.3333333333333333703, 0.3333333333333333703, 0.3333333333333333703),
 ( 0.3333333333333333703, 0.3333333333333333703, 0.3333333333333333703, 0.3333333333333333703, 0.3333333333333333703, 0.3333333333333333703, 0.3333333333333333703, 0.3333333333333333703, 0.3333333333333333703, 0.3333333333333333703, 0.3333333333333333703, 0.3333333333333333703, 0.3333333333333333703, 0.3333333333333333703, 0.3333333333333333703, 0.3333333333333333703, 0.3333333333333333703, 0.3333333333333333703, 0.3333333333333333703, 0.3333333333333333703, 0.3333333333333333703, 0.3333333333333333703, 0.3333333333333333703, 0.3333333333333333703, 0.3333333333333333703, 0.3333333333333333703, 0.3333333333333333703, 0.3333333333333333703, 0.3333333333333333703, 0.3333333333333333703, 0.3333333333333333703, 0.3333333333333333703, 0.3333333333333333703, 0.3333333333333333703, 0.3333333333333333703, 0.3333333333333333703, 0.3333333333333333703, 0.3333333333333333703, 0.3333333333333333703, 0.3333333333333333703, 0.3333333333333333703, 0.3333333333333333703, 0.3333333333333333703, 0.3333333333333333703, 0.3333333333333333703, 0.3333333333333333703, 0.3333333333333333703, 0.3333333333333333703, 0.3333333333333333703, 0.3333333333333333703, 0.3333333333333333703, 0.3333333333333333703, 0.3333333333333333703, 0.3333333333333333703, 0.3333333333333333703, 0.3333333333333333703, 0.3333333333333333703, 0.3333333333333333703, 0.3333333333333333703, 0.3333333333333333703, 0.3333333333333333703, 0.3333333333333333703, 0.3333333333333333703, 0.3333333333333333703, 0.3333333333333333703, 0.3333333333333333703, 0.3333333333333333703, 0.3333333333333333703, 0.3333333333333333703, 0.3333333333333333703, 0.3333333333333333703, 0.3333333333333333703, 0.3333333333333333703, 0.3333333333333333703, 0.3333333333333333703, 0.3333333333333333703, 0.3333333333333333703, 0.3333333333333333703, 0.3333333333333333703, 0.3333333333333333703, 0.3333333333333333703, 0.3333333333333333703, 0.3333333333333333703, 0.3333333333333333703, 0.3333333333333333703, 0.3333333333333333703, 0.3333333333333333703, 0.3333333333333333703, 0.3333333333333333703, 0.3333333333333333703, 0.3333333333333333703, 0.3333333333333333703, 0.3333333333333333703, 0.3333333333333333703, 0.3333333333333333703, 0.3333333333333333703, 0.3333333333333333703, 0.3333333333333333703, 0.3333333333333333703, 0.3333333333333333703, 0.3333333333333333703, 0.3333333333333333703, 0.3333333333333333703, 0.3333333333333333703, 0.3333333333333333703, 0.3333333333333333703, 0.3333333333333333703, 0.3333333333333333703, 0.3333333333333333703, 0.3333333333333333703, 0.3333333333333333703, 0.3333333333333333703, 0.3333333333333333703, 0.3333333333333333703, 0.3333333333333333703, 0.3333333333333333703, 0.3333333333333333703, 0.3333333333333333703, 0.3333333333333333703, 0.3333333333333333703, 0.3333333333333333703, 0.3333333333333333703, 0.3333333333333333703, 0.3333333333333333703, 0.3333333333333333703, 0.3333333333333333703, 0.3333333333333333703, 0.3333333333333333703, 0.3333333333333333703, 0.3333333333333333703, 0.3333333333333333703, 0.3333333333333333703, 0.3333333333333333703, 0.3333333333333333703, 0.3333333333333333703, 0.3333333333333333703, 0.3333333333333333703, 0.3333333333333333703, 0.3333333333333333703, 0.3333333333333333703, 0.3333333333333333703, 0.3333333333333333703, 0.3333333333333333703, 0.3333333333333333703, 0.3333333333333333703, 0.3333333333333333703, 0.3333333333333333703, 0.3333333333333333703, 0.3333333333333333703, 0.3333333333333333703, 0.3333333333333333703, 0.3333333333333333703, 0.3333333333333333703, 0.3333333333333333703, 0.3333333333333333703, 0.3333333333333333703, 0.3333333333333333703, 0.3333333333333333703, 0.3333333333333333703, 0.3333333333333333703, 0.3333333333333333703, 0.3333333333333333703, 0.3333333333333333703, 0.3333333333333333703, 0.3333333333333333703, 0.3333333333333333703, 0.3333333333333333703, 0.3333333333333333703, 0.3333333333333333703, 0.3333333333333333703, 0.3333333333333333703, 0.3333333333333333703, 0.3333333333333333703, 0.3333333333333333703, 0.3333333333333333703, 0.3333333333333333703, 0.3333333333333333703, 0.3333333333333333703, 0.3333333333333333703, 0.3333333333333333703, 0.3333333333333333703, 0.3333333333333333703, 0.3333333333333333703, 0.3333333333333333703, 0.3333333333333333703, 0.3333333333333333703, 0.3333333333333333703, 0.3333333333333333703, 0.3333333333333333703, 0.3333333333333333703, 0.3333333333333333703, 0.3333333333333333703, 0.3333333333333333703, 0.3333333333333333703, 0.3333333333333333703, 0.3333333333333333703, 0.3333333333333333703, 0.3333333333333333703, 0.3333333333333333703, 0.3333333333333333703, 0.3333333333333333703, 0.3333333333333333703, 0.3333333333333333703, 0.3333333333333333703, 0.3333333333333333703, 0.3333333333333333703, 0.3333333333333333703, 0.3333333333333333703, 0.3333333333333333703, 0.3333333333333333703, 0.3333333333333333703, 0.3333333333333333703, 0.3333333333333333703, 0.3333333333333333703, 0.3333333333333333703, 0.3333333333333333703, 0.3333333333333333703, 0.3333333333333333703, 0.3333333333333333703, 0.3333333333333333703, 0.3333333333333333703, 0.3333333333333333703, 0.3333333333333333703, 0.3333333333333333703, 0.3333333333333333703, 0.3333333333333333703, 0.3333333333333333703, 0.3333333333333333703, 0.3333333333333333703, 0.3333333333333333703, 0.3333333333333333703, 0.3333333333333333703, 0.3333333333333333703, 0.3333333333333333703, 0.3333333333333333703, 0.3333333333333333703, 0.3333333333333333703, 0.3333333333333333703, 0.3333333333333333703, 0.3333333333333333703, 0.3333333333333333703, 0.3333333333333333703, 0.3333333333333333703, 0.3333333333333333703, 0.3333333333333333703, 0.3333333333333333703),
 ( 1.000000000000000000, 1.000000000000000000, 1.000000000000000000, 1.000000000000000000, 1.000000000000000000, 1.000000000000000000, 1.000000000000000000, 1.000000000000000000, 1.000000000000000000, 1.000000000000000000, 1.000000000000000000, 1.000000000000000000, 1.000000000000000000, 1.000000000000000000, 1.000000000000000000, 1.000000000000000000, 1.000000000000000000, 1.000000000000000000, 1.000000000000000000, 1.000000000000000000, 1.000000000000000000, 1.000000000000000000, 1.000000000000000000, 1.000000000000000000, 1.000000000000000000, 1.000000000000000000, 1.000000000000000000, 1.000000000000000000, 1.000000000000000000, 1.000000000000000000, 1.000000000000000000, 1.000000000000000000, 1.000000000000000000, 1.000000000000000000, 1.000000000000000000, 1.000000000000000000, 1.000000000000000000, 1.000000000000000000, 1.000000000000000000, 1.000000000000000000, 1.000000000000000000, 1.000000000000000000, 1.000000000000000000, 1.000000000000000000, 1.000000000000000000, 1.000000000000000000, 1.000000000000000000, 1.000000000000000000, 1.000000000000000000, 1.000000000000000000, 1.000000000000000000, 1.000000000000000000, 1.000000000000000000, 1.000000000000000000, 1.000000000000000000, 1.000000000000000000, 1.000000000000000000, 1.000000000000000000, 1.000000000000000000, 1.000000000000000000, 1.000000000000000000, 1.000000000000000000, 1.000000000000000000, 1.000000000000000000, 1.000000000000000000, 1.000000000000000000, 1.000000000000000000, 1.000000000000000000, 1.000000000000000000, 1.000000000000000000, 1.000000000000000000, 1.000000000000000000, 1.000000000000000000, 1.000000000000000000, 1.000000000000000000, 1.000000000000000000, 1.000000000000000000, 1.000000000000000000, 1.000000000000000000, 1.000000000000000000, 1.000000000000000000, 1.000000000000000000, 1.000000000000000000, 1.000000000000000000, 1.000000000000000000, 1.000000000000000000, 1.000000000000000000, 1.000000000000000000, 1.000000000000000000, 1.000000000000000000, 1.000000000000000000, 1.000000000000000000, 1.000000000000000000, 1.000000000000000000, 1.000000000000000000, 1.000000000000000000, 1.000000000000000000, 1.000000000000000000, 1.000000000000000000, 1.000000000000000000, 1.000000000000000000, 1.000000000000000000, 1.000000000000000000, 1.000000000000000000, 1.000000000000000000, 1.000000000000000000, 1.000000000000000000, 1.000000000000000000, 1.000000000000000000, 1.000000000000000000, 1.000000000000000000, 1.000000000000000000, 1.000000000000000000, 1.000000000000000000, 1.000000000000000000, 1.000000000000000000, 1.000000000000000000, 1.000000000000000000, 1.000000000000000000, 1.000000000000000000, 1.000000000000000000, 1.000000000000000000, 1.000000000000000000, 1.000000000000000000, 1.000000000000000000, 1.000000000000000000, 1.000000000000000000, 1.000000000000000000, 1.000000000000000000, 1.000000000000000000, 1.000000000000000000, 1.000000000000000000, 1.000000000000000000, 1.000000000000000000, 1.000000000000000000, 1.000000000000000000, 1.000000000000000000, 1.000000000000000000, 1.000000000000000000, 1.000000000000000000, 1.000000000000000000, 1.000000000000000000, 1.000000000000000000, 1.000000000000000000, 1.000000000000000000, 1.000000000000000000, 1.000000000000000000, 1.000000000000000000, 1.000000000000000000, 1.000000000000000000, 1.000000000000000000, 1.000000000000000000, 1.000000000000000000, 1.000000000000000000, 1.000000000000000000, 1.000000000000000000, 1.000000000000000000, 1.000000000000000000, 1.000000000000000000, 1.000000000000000000, 1.000000000000000000, 1.000000000000000000, 1.000000000000000000, 1.000000000000000000, 1.000000000000000000, 1.000000000000000000, 1.000000000000000000, 1.000000000000000000, 1.000000000000000000, 1.000000000000000000, 1.000000000000000000, 1.000000000000000000, 1.000000000000000000, 1.000000000000000000, 1.000000000000000000, 1.000000000000000000, 1.000000000000000000, 1.000000000000000000, 1.000000000000000000, 1.000000000000000000, 1.000000000000000000, 1.000000000000000000, 1.000000000000000000, 1.000000000000000000, 1.000000000000000000, 1.000000000000000000, 1.000000000000000000, 1.000000000000000000, 1.000000000000000000, 1.000000000000000000, 1.000000000000000000, 1.000000000000000000, 1.000000000000000000, 1.000000000000000000, 1.000000000000000000, 1.000000000000000000, 1.000000000000000000, 1.000000000000000000, 1.000000000000000000, 1.000000000000000000, 1.000000000000000000, 1.000000000000000000, 1.000000000000000000, 1.000000000000000000, 1.000000000000000000, 1.000000000000000000, 1.000000000000000000, 1.000000000000000000, 1.000000000000000000, 1.000000000000000000, 1.000000000000000000, 1.000000000000000000, 1.000000000000000000, 1.000000000000000000, 1.000000000000000000, 1.000000000000000000, 1.000000000000000000, 1.000000000000000000, 1.000000000000000000, 1.000000000000000000, 1.000000000000000000, 1.000000000000000000, 1.000000000000000000, 1.000000000000000000, 1.000000000000000000, 1.000000000000000000, 1.000000000000000000, 1.000000000000000000, 1.000000000000000000, 1.000000000000000000, 1.000000000000000000, 1.000000000000000000, 1.000000000000000000, 1.000000000000000000, 1.000000000000000000, 1.000000000000000000, 1.000000000000000000, 1.000000000000000000, 1.000000000000000000, 1.000000000000000000, 1.000000000000000000, 1.000000000000000000, 1.000000000000000000, 1.000000000000000000, 1.000000000000000000, 1.000000000000000000),
 ( 0.3333333333333333703, 0.3333333333333333703, 0.3333333333333333703, 0.3333333333333333703, 0.3333333333333333703, 0.3333333333333333703, 0.3333333333333333703, 0.3333333333333333703, 0.3333333333333333703, 0.3333333333333333703, 0.3333333333333333703, 0.3333333333333333703, 0.3333333333333333703, 0.3333333333333333703, 0.3333333333333333703, 0.3333333333333333703, 0.3333333333333333703, 0.3333333333333333703, 0.3333333333333333703, 0.3333333333333333703, 0.3333333333333333703, 0.3333333333333333703, 0.3333333333333333703, 0.3333333333333333703, 0.3333333333333333703, 0.3333333333333333703, 0.3333333333333333703, 0.3333333333333333703, 0.3333333333333333703, 0.3333333333333333703, 0.3333333333333333703, 0.3333333333333333703, 0.3333333333333333703, 0.3333333333333333703, 0.3333333333333333703, 0.3333333333333333703, 0.3333333333333333703, 0.3333333333333333703, 0.3333333333333333703, 0.3333333333333333703, 0.3333333333333333703, 0.3333333333333333703, 0.3333333333333333703, 0.3333333333333333703, 0.3333333333333333703, 0.3333333333333333703, 0.3333333333333333703, 0.3333333333333333703, 0.3333333333333333703, 0.3333333333333333703, 0.3333333333333333703, 0.3333333333333333703, 0.3333333333333333703, 0.3333333333333333703, 0.3333333333333333703, 0.3333333333333333703, 0.3333333333333333703, 0.3333333333333333703, 0.3333333333333333703, 0.3333333333333333703, 0.3333333333333333703, 0.3333333333333333703, 0.3333333333333333703, 0.3333333333333333703, 0.3333333333333333703, 0.3333333333333333703, 0.3333333333333333703, 0.3333333333333333703, 0.3333333333333333703, 0.3333333333333333703, 0.3333333333333333703, 0.3333333333333333703, 0.3333333333333333703, 0.3333333333333333703, 0.3333333333333333703, 0.3333333333333333703, 0.3333333333333333703, 0.3333333333333333703, 0.3333333333333333703, 0.3333333333333333703, 0.3333333333333333703, 0.3333333333333333703, 0.3333333333333333703, 0.3333333333333333703, 0.3333333333333333703, 0.3333333333333333703, 0.3333333333333333703, 0.3333333333333333703, 0.3333333333333333703, 0.3333333333333333703, 0.3333333333333333703, 0.3333333333333333703, 0.3333333333333333703, 0.3333333333333333703, 0.3333333333333333703, 0.3333333333333333703, 0.3333333333333333703, 0.3333333333333333703, 0.3333333333333333703, 0.3333333333333333703, 0.3333333333333333703, 0.3333333333333333703, 0.3333333333333333703, 0.3333333333333333703, 0.3333333333333333703, 0.3333333333333333703, 0.3333333333333333703, 0.3333333333333333703, 0.3333333333333333703, 0.3333333333333333703, 0.3333333333333333703, 0.3333333333333333703, 0.3333333333333333703, 0.3333333333333333703, 0.3333333333333333703, 0.3333333333333333703, 0.3333333333333333703, 0.3333333333333333703, 0.3333333333333333703, 0.3333333333333333703, 0.3333333333333333703, 0.3333333333333333703, 0.3333333333333333703, 0.3333333333333333703, 0.3333333333333333703, 0.3333333333333333703, 0.3333333333333333703, 0.3333333333333333703, 0.3333333333333333703, 0.3333333333333333703, 0.3333333333333333703, 0.3333333333333333703, 0.3333333333333333703, 0.3333333333333333703, 0.3333333333333333703, 0.3333333333333333703, 0.3333333333333333703, 0.3333333333333333703, 0.3333333333333333703, 0.3333333333333333703, 0.3333333333333333703, 0.3333333333333333703, 0.3333333333333333703, 0.3333333333333333703, 0.3333333333333333703, 0.3333333333333333703, 0.3333333333333333703, 0.3333333333333333703, 0.3333333333333333703, 0.3333333333333333703, 0.3333333333333333703, 0.3333333333333333703, 0.3333333333333333703, 0.3333333333333333703, 0.3333333333333333703, 0.3333333333333333703, 0.3333333333333333703, 0.3333333333333333703, 0.3333333333333333703, 0.3333333333333333703, 0.3333333333333333703, 0.3333333333333333703, 0.3333333333333333703, 0.3333333333333333703, 0.3333333333333333703, 0.3333333333333333703, 0.3333333333333333703, 0.3333333333333333703, 0.3333333333333333703, 0.3333333333333333703, 0.3333333333333333703, 0.3333333333333333703, 0.3333333333333333703, 0.3333333333333333703, 0.3333333333333333703, 0.3333333333333333703, 0.3333333333333333703, 0.3333333333333333703, 0.3333333333333333703, 0.3333333333333333703, 0.3333333333333333703, 0.3333333333333333703, 0.3333333333333333703, 0.3333333333333333703, 0.3333333333333333703, 0.3333333333333333703, 0.3333333333333333703, 0.3333333333333333703, 0.3333333333333333703, 0.3333333333333333703, 0.3333333333333333703, 0.3333333333333333703, 0.3333333333333333703, 0.3333333333333333703, 0.3333333333333333703, 0.3333333333333333703, 0.3333333333333333703, 0.3333333333333333703, 0.3333333333333333703, 0.3333333333333333703, 0.3333333333333333703, 0.3333333333333333703, 0.3333333333333333703, 0.3333333333333333703, 0.3333333333333333703, 0.3333333333333333703, 0.3333333333333333703, 0.3333333333333333703, 0.3333333333333333703, 0.3333333333333333703, 0.3333333333333333703, 0.3333333333333333703, 0.3333333333333333703, 0.3333333333333333703, 0.3333333333333333703, 0.3333333333333333703, 0.3333333333333333703, 0.3333333333333333703, 0.3333333333333333703, 0.3333333333333333703, 0.3333333333333333703, 0.3333333333333333703, 0.3333333333333333703, 0.3333333333333333703, 0.3333333333333333703, 0.3333333333333333703, 0.3333333333333333703, 0.3333333333333333703, 0.3333333333333333703, 0.3333333333333333703, 0.3333333333333333703, 0.3333333333333333703, 0.3333333333333333703, 0.3333333333333333703, 0.3333333333333333703, 0.3333333333333333703, 0.3333333333333333703, 0.3333333333333333703, 0.3333333333333333703, 0.3333333333333333703, 0.3333333333333333703, 0.3333333333333333703, 0.3333333333333333703, 0.3333333333333333703, 0.3333333333333333703, 0.3333333333333333703),
 ( 0.3333333333333333703, 0.3333333333333333703, 0.3333333333333333703, 0.3333333333333333703, 0.3333333333333333703, 0.3333333333333333703, 0.3333333333333333703, 0.3333333333333333703, 0.3333333333333333703, 0.3333333333333333703, 0.3333333333333333703, 0.3333333333333333703, 0.3333333333333333703, 0.3333333333333333703, 0.3333333333333333703, 0.3333333333333333703, 0.3333333333333333703, 0.3333333333333333703, 0.3333333333333333703, 0.3333333333333333703, 0.3333333333333333703, 0.3333333333333333703, 0.3333333333333333703, 0.3333333333333333703, 0.3333333333333333703, 0.3333333333333333703, 0.3333333333333333703, 0.3333333333333333703, 0.3333333333333333703, 0.3333333333333333703, 0.3333333333333333703, 0.3333333333333333703, 0.3333333333333333703, 0.3333333333333333703, 0.3333333333333333703, 0.3333333333333333703, 0.3333333333333333703, 0.3333333333333333703, 0.3333333333333333703, 0.3333333333333333703, 0.3333333333333333703, 0.3333333333333333703, 0.3333333333333333703, 0.3333333333333333703, 0.3333333333333333703, 0.3333333333333333703, 0.3333333333333333703, 0.3333333333333333703, 0.3333333333333333703, 0.3333333333333333703, 0.3333333333333333703, 0.3333333333333333703, 0.3333333333333333703, 0.3333333333333333703, 0.3333333333333333703, 0.3333333333333333703, 0.3333333333333333703, 0.3333333333333333703, 0.3333333333333333703, 0.3333333333333333703, 0.3333333333333333703, 0.3333333333333333703, 0.3333333333333333703, 0.3333333333333333703, 0.3333333333333333703, 0.3333333333333333703, 0.3333333333333333703, 0.3333333333333333703, 0.3333333333333333703, 0.3333333333333333703, 0.3333333333333333703, 0.3333333333333333703, 0.3333333333333333703, 0.3333333333333333703, 0.3333333333333333703, 0.3333333333333333703, 0.3333333333333333703, 0.3333333333333333703, 0.3333333333333333703, 0.3333333333333333703, 0.3333333333333333703, 0.3333333333333333703, 0.3333333333333333703, 0.3333333333333333703, 0.3333333333333333703, 0.3333333333333333703, 0.3333333333333333703, 0.3333333333333333703, 0.3333333333333333703, 0.3333333333333333703, 0.3333333333333333703, 0.3333333333333333703, 0.3333333333333333703, 0.3333333333333333703, 0.3333333333333333703, 0.3333333333333333703, 0.3333333333333333703, 0.3333333333333333703, 0.3333333333333333703, 0.3333333333333333703, 0.3333333333333333703, 0.3333333333333333703, 0.3333333333333333703, 0.3333333333333333703, 0.3333333333333333703, 0.3333333333333333703, 0.3333333333333333703, 0.3333333333333333703, 0.3333333333333333703, 0.3333333333333333703, 0.3333333333333333703, 0.3333333333333333703, 0.3333333333333333703, 0.3333333333333333703, 0.3333333333333333703, 0.3333333333333333703, 0.3333333333333333703, 0.3333333333333333703, 0.3333333333333333703, 0.3333333333333333703, 0.3333333333333333703, 0.3333333333333333703, 0.3333333333333333703, 0.3333333333333333703, 0.3333333333333333703, 0.3333333333333333703, 0.3333333333333333703, 0.3333333333333333703, 0.3333333333333333703, 0.3333333333333333703, 0.3333333333333333703, 0.3333333333333333703, 0.3333333333333333703, 0.3333333333333333703, 0.3333333333333333703, 0.3333333333333333703, 0.3333333333333333703, 0.3333333333333333703, 0.3333333333333333703, 0.3333333333333333703, 0.3333333333333333703, 0.3333333333333333703, 0.3333333333333333703, 0.3333333333333333703, 0.3333333333333333703, 0.3333333333333333703, 0.3333333333333333703, 0.3333333333333333703, 0.3333333333333333703, 0.3333333333333333703, 0.3333333333333333703, 0.3333333333333333703, 0.3333333333333333703, 0.3333333333333333703, 0.3333333333333333703, 0.3333333333333333703, 0.3333333333333333703, 0.3333333333333333703, 0.3333333333333333703, 0.3333333333333333703, 0.3333333333333333703, 0.3333333333333333703, 0.3333333333333333703, 0.3333333333333333703, 0.3333333333333333703, 0.3333333333333333703, 0.3333333333333333703, 0.3333333333333333703, 0.3333333333333333703, 0.3333333333333333703, 0.3333333333333333703, 0.3333333333333333703, 0.3333333333333333703, 0.3333333333333333703, 0.3333333333333333703, 0.3333333333333333703, 0.3333333333333333703, 0.3333333333333333703, 0.3333333333333333703, 0.3333333333333333703, 0.3333333333333333703, 0.3333333333333333703, 0.3333333333333333703, 0.3333333333333333703, 0.3333333333333333703, 0.3333333333333333703, 0.3333333333333333703, 0.3333333333333333703, 0.3333333333333333703, 0.3333333333333333703, 0.3333333333333333703, 0.3333333333333333703, 0.3333333333333333703, 0.3333333333333333703, 0.3333333333333333703, 0.3333333333333333703, 0.3333333333333333703, 0.3333333333333333703, 0.3333333333333333703, 0.3333333333333333703, 0.3333333333333333703, 0.3333333333333333703, 0.3333333333333333703, 0.3333333333333333703, 0.3333333333333333703, 0.3333333333333333703, 0.3333333333333333703, 0.3333333333333333703, 0.3333333333333333703, 0.3333333333333333703, 0.3333333333333333703, 0.3333333333333333703, 0.3333333333333333703, 0.3333333333333333703, 0.3333333333333333703, 0.3333333333333333703, 0.3333333333333333703, 0.3333333333333333703, 0.3333333333333333703, 0.3333333333333333703, 0.3333333333333333703, 0.3333333333333333703, 0.3333333333333333703, 0.3333333333333333703, 0.3333333333333333703, 0.3333333333333333703, 0.3333333333333333703, 0.3333333333333333703, 0.3333333333333333703, 0.3333333333333333703, 0.3333333333333333703, 0.3333333333333333703, 0.3333333333333333703, 0.3333333333333333703, 0.3333333333333333703, 0.3333333333333333703, 0.3333333333333333703, 0.3333333333333333703, 0.3333333333333333703, 0.3333333333333333703, 0.3333333333333333703, 0.3333333333333333703, 0.3333333333333333703, 0.3333333333333333703, 0.3333333333333333703, 0.3333333333333333703),
 ( 1.000000000000000000, 1.000000000000000000, 1.000000000000000000, 1.000000000000000000, 1.000000000000000000, 1.000000000000000000, 1.000000000000000000, 1.000000000000000000, 1.000000000000000000, 1.000000000000000000, 1.000000000000000000, 1.000000000000000000, 1.000000000000000000, 1.000000000000000000, 1.000000000000000000, 1.000000000000000000, 1.000000000000000000, 1.000000000000000000, 1.000000000000000000, 1.000000000000000000, 1.000000000000000000, 1.000000000000000000, 1.000000000000000000, 1.000000000000000000, 1.000000000000000000, 1.000000000000000000, 1.000000000000000000, 1.000000000000000000, 1.000000000000000000, 1.000000000000000000, 1.000000000000000000, 1.000000000000000000, 1.000000000000000000, 1.000000000000000000, 1.000000000000000000, 1.000000000000000000, 1.000000000000000000, 1.000000000000000000, 1.000000000000000000, 1.000000000000000000, 1.000000000000000000, 1.000000000000000000, 1.000000000000000000, 1.000000000000000000, 1.000000000000000000, 1.000000000000000000, 1.000000000000000000, 1.000000000000000000, 1.000000000000000000, 1.000000000000000000, 1.000000000000000000, 1.000000000000000000, 1.000000000000000000, 1.000000000000000000, 1.000000000000000000, 1.000000000000000000, 1.000000000000000000, 1.000000000000000000, 1.000000000000000000, 1.000000000000000000, 1.000000000000000000, 1.000000000000000000, 1.000000000000000000, 1.000000000000000000, 1.000000000000000000, 1.000000000000000000, 1.000000000000000000, 1.000000000000000000, 1.000000000000000000, 1.000000000000000000, 1.000000000000000000, 1.000000000000000000, 1.000000000000000000, 1.000000000000000000, 1.000000000000000000, 1.000000000000000000, 1.000000000000000000, 1.000000000000000000, 1.000000000000000000, 1.000000000000000000, 1.000000000000000000, 1.000000000000000000, 1.000000000000000000, 1.000000000000000000, 1.000000000000000000, 1.000000000000000000, 1.000000000000000000, 1.000000000000000000, 1.000000000000000000, 1.000000000000000000, 1.000000000000000000, 1.000000000000000000, 1.000000000000000000, 1.000000000000000000, 1.000000000000000000, 1.000000000000000000, 1.000000000000000000, 1.000000000000000000, 1.000000000000000000, 1.000000000000000000, 1.000000000000000000, 1.000000000000000000, 1.000000000000000000, 1.000000000000000000, 1.000000000000000000, 1.000000000000000000, 1.000000000000000000, 1.000000000000000000, 1.000000000000000000, 1.000000000000000000, 1.000000000000000000, 1.000000000000000000, 1.000000000000000000, 1.000000000000000000, 1.000000000000000000, 1.000000000000000000, 1.000000000000000000, 1.000000000000000000, 1.000000000000000000, 1.000000000000000000, 1.000000000000000000, 1.000000000000000000, 1.000000000000000000, 1.000000000000000000, 1.000000000000000000, 1.000000000000000000, 1.000000000000000000, 1.000000000000000000, 1.000000000000000000, 1.000000000000000000, 1.000000000000000000, 1.000000000000000000, 1.000000000000000000, 1.000000000000000000, 1.000000000000000000, 1.000000000000000000, 1.000000000000000000, 1.000000000000000000, 1.000000000000000000, 1.000000000000000000, 1.000000000000000000, 1.000000000000000000, 1.000000000000000000, 1.000000000000000000, 1.000000000000000000, 1.000000000000000000, 1.000000000000000000, 1.000000000000000000, 1.000000000000000000, 1.000000000000000000, 1.000000000000000000, 1.000000000000000000, 1.000000000000000000, 1.000000000000000000, 1.000000000000000000, 1.000000000000000000, 1.000000000000000000, 1.000000000000000000, 1.000000000000000000, 1.000000000000000000, 1.000000000000000000, 1.000000000000000000, 1.000000000000000000, 1.000000000000000000, 1.000000000000000000, 1.000000000000000000, 1.000000000000000000, 1.000000000000000000, 1.000000000000000000, 1.000000000000000000, 1.000000000000000000, 1.000000000000000000, 1.000000000000000000, 1.000000000000000000, 1.000000000000000000, 1.000000000000000000, 1.000000000000000000, 1.000000000000000000, 1.000000000000000000, 1.000000000000000000, 1.000000000000000000, 1.000000000000000000, 1.000000000000000000, 1.000000000000000000, 1.000000000000000000, 1.000000000000000000, 1.000000000000000000, 1.000000000000000000, 1.000000000000000000, 1.000000000000000000, 1.000000000000000000, 1.000000000000000000, 1.000000000000000000, 1.000000000000000000, 1.000000000000000000, 1.000000000000000000, 1.000000000000000000, 1.000000000000000000, 1.000000000000000000, 1.000000000000000000, 1.000000000000000000, 1.000000000000000000, 1.000000000000000000, 1.000000000000000000, 1.000000000000000000, 1.000000000000000000, 1.000000000000000000, 1.000000000000000000, 1.000000000000000000, 1.000000000000000000, 1.000000000000000000, 1.000000000000000000, 1.000000000000000000, 1.000000000000000000, 1.000000000000000000, 1.000000000000000000, 1.000000000000000000, 1.000000000000000000, 1.000000000000000000, 1.000000000000000000, 1.000000000000000000, 1.000000000000000000, 1.000000000000000000, 1.000000000000000000, 1.000000000000000000, 1.000000000000000000, 1.000000000000000000, 1.000000000000000000, 1.000000000000000000, 1.000000000000000000, 1.000000000000000000, 1.000000000000000000, 1.000000000000000000, 1.000000000000000000, 1.000000000000000000, 1.000000000000000000, 1.000000000000000000, 1.000000000000000000, 1.000000000000000000, 1.000000000000000000, 1.000000000000000000, 1.000000000000000000, 1.000000000000000000, 1.000000000000000000, 1.000000000000000000, 1.000000000000000000) ) ) 
 REPRESENTATION_ITEM ( '' )  SURFACE ( )  );
#20656=CARTESIAN_POINT ( 'NONE',  ( 25.50411877999659893, -13.63830170496968996, -16.08255890605547123 ) ) ;
#20657=CARTESIAN_POINT ( 'NONE',  ( 27.28133297882270014, -12.52022702279392874, -15.45456112525011427 ) ) ;
#20666=CARTESIAN_POINT ( 'NONE',  ( 23.76792026503975919, -8.198361753721227885, -14.67730844950409441 ) ) ;
#20667=CARTESIAN_POINT ( 'NONE',  ( 18.39996379557756256, 0.6904185378075045065, -15.43317298867526866 ) ) ;
#20670=CARTESIAN_POINT ( 'NONE',  ( 33.74345058881453241, -15.07496310474945922, -20.85461858825047798 ) ) ;
#20672=CARTESIAN_POINT ( 'NONE',  ( 11.46775782571576130, 9.292755756535285627, -15.86302895122203616 ) ) ;
#20676=CARTESIAN_POINT ( 'NONE',  ( 9.668378799564367299, 16.22503635135577227, -17.88486489230207965 ) ) ;
#20679=CARTESIAN_POINT ( 'NONE',  ( 12.51417009928267099, 8.576964204390579383, -15.11888119342340353 ) ) ;
#20687=CARTESIAN_POINT ( 'NONE',  ( 9.120682955242472190, 16.14398363876680520, -17.05135327743868245 ) ) ;
#20688=CARTESIAN_POINT ( 'NONE',  ( 32.00110207675911767, -10.95298233446834502, -16.54939777171900417 ) ) ;
#20690=CARTESIAN_POINT ( 'NONE',  ( 18.53087132295907935, 5.398958961476600038, -21.24745519132487459 ) ) ;
#20691=CARTESIAN_POINT ( 'NONE',  ( 17.40794641162625567, 9.636182090832996039, -14.27881468665684395 ) ) ;
#20693=CARTESIAN_POINT ( 'NONE',  ( 25.10166869626759123, -5.595937160916529152, -20.34551573546397307 ) ) ;
#20703=CARTESIAN_POINT ( 'NONE',  ( 35.54859390953724585, -21.18451583373416014, -18.06010107863414405 ) ) ;
#20704=CARTESIAN_POINT ( 'NONE',  ( 11.28991474634619863, 7.910464746135025926, -16.02350989558273753 ) ) ;
#20707=CARTESIAN_POINT ( 'NONE',  ( 28.01381056668970260, -10.10121741814351459, -18.82353034625045041 ) ) ;
#20709=CARTESIAN_POINT ( 'NONE',  ( 11.37973238226026318, 12.28930733048782642, -16.95943368139929319 ) ) ;
#20715=CARTESIAN_POINT ( 'NONE',  ( 12.51417009928267099, 8.576964204390579383, -15.11888119342340353 ) ) ;
#20720=CARTESIAN_POINT ( 'NONE',  ( 9.667809135389937580, 16.22764890387498227, -17.88510185254740747 ) ) ;
#20721=CARTESIAN_POINT ( 'NONE',  ( 22.74932893098897324, -1.793276863599028381, -13.92998459126509836 ) ) ;
#20722=CARTESIAN_POINT ( 'NONE',  ( 20.01442678821067034, -2.980627454636011198, -16.03144472681325183 ) ) ;
#20724=CARTESIAN_POINT ( 'NONE',  ( 17.40782953567980229, 3.270613820851801190, -14.52895612053623609 ) ) ;
#20728=CARTESIAN_POINT ( 'NONE',  ( 22.39939798857497877, 2.694615832958070722, -14.02792042734668065 ) ) ;
#20734=CARTESIAN_POINT ( 'NONE',  ( 10.35865474790814211, 16.97209951875106526, -17.91014213605047445 ) ) ;
#20744=CARTESIAN_POINT ( 'NONE',  ( 17.32873655921053313, 10.26331207550778579, -16.20725374984683143 ) ) ;
#20745=CARTESIAN_POINT ( 'NONE',  ( 11.05714535396004727, 17.68148921877153157, -17.77574279453144968 ) ) ;
#20746=CARTESIAN_POINT ( 'NONE',  ( 34.11209566957792561, -15.73109017586260272, -19.92372960426217787 ) ) ;
#20750=CARTESIAN_POINT ( 'NONE',  ( 9.641350810849047548, 17.66889113945805789, -17.91796598306941135 ) ) ;
#20752=CARTESIAN_POINT ( 'NONE',  ( 12.86487521014348623, 7.673917307032582791, -14.83936302970355037 ) ) ;
#20757=CARTESIAN_POINT ( 'NONE',  ( 10.47151541139924547, 16.45450612959241354, -17.33501744001014444 ) ) ;
#20759=CARTESIAN_POINT ( 'NONE',  ( 36.54859390953724585, -21.18451583373416014, -18.06010107863414405 ) ) ;
#20760=CARTESIAN_POINT ( 'NONE',  ( 28.16462234717350199, -5.661059359726887230, -16.30864077692347536 ) ) ;
#20765=CARTESIAN_POINT ( 'NONE',  ( 26.88053589187069292, -12.95240298029966119, -14.33176627689639382 ) ) ;
#20766=CARTESIAN_POINT ( 'NONE',  ( 23.87837110222071502, -4.315358902625421322, -12.52832693522684693 ) ) ;
#20782=CARTESIAN_POINT ( 'NONE',  ( 10.33811723165831786, 18.38618817278374706, -17.91339614244408907 ) ) ;
#20788=CARTESIAN_POINT ( 'NONE',  ( 11.45661370752365116, 9.343864103108954211, -15.86763743611193789 ) ) ;
#20790=CARTESIAN_POINT ( 'NONE',  ( 17.31141255128542511, 8.026854538702009378, -19.31233526832781777 ) ) ;
#20793=CARTESIAN_POINT ( 'NONE',  ( 24.60501232743784783, -9.531698448777172317, -16.22453333552994792 ) ) ;
#20797=CARTESIAN_POINT ( 'NONE',  ( 12.24518234991790955, 9.516123393600787850, -15.33326918312795328 ) ) ;
#20798=CARTESIAN_POINT ( 'NONE',  ( 34.75406370242679799, -18.61511248754081294, -20.11778113987843852 ) ) ;
#20802=CARTESIAN_POINT ( 'NONE',  ( 22.82249278870453679, 0.4072072893072278821, -18.57859108775207702 ) ) ;
#20805=CARTESIAN_POINT ( 'NONE',  ( 21.92441584138004984, 2.204866226087792924, -14.79409581392398110 ) ) ;
#20807=CARTESIAN_POINT ( 'NONE',  ( 28.29154804861901340, -7.753790107393749409, -19.00671289252072782 ) ) ;
#20818=CARTESIAN_POINT ( 'NONE',  ( 9.641351338355821810, 17.66888872024471624, -17.91303689663363130 ) ) ;
#20820=CARTESIAN_POINT ( 'NONE',  ( 24.28190956353967422, -4.127413435877471670, -12.52835809790152766 ) ) ;
#20821=CARTESIAN_POINT ( 'NONE',  ( 17.10097030076851610, 6.697663726599960121, -13.82760435466811089 ) ) ;
#20822=CARTESIAN_POINT ( 'NONE',  ( 34.59940796595157053, -18.92032618698594248, -21.11335396907232465 ) ) ;
#20828=CARTESIAN_POINT ( 'NONE',  ( 16.21960234321935701, 7.070186740785398882, -14.59618053200276044 ) ) ;
#20831=CARTESIAN_POINT ( 'NONE',  ( 12.50736435846123484, 8.573956625762026107, -15.12430548898761806 ) ) ;
#20835=CARTESIAN_POINT ( 'NONE',  ( 17.69365662292968366, 10.27476822432933545, -17.01437286930526227 ) ) ;
#20838=CARTESIAN_POINT ( 'NONE',  ( 9.110807846758516959, 16.18927214505777812, -17.05547580459120383 ) ) ;
#20839=CARTESIAN_POINT ( 'NONE',  ( 33.18306031693006730, -12.55741664378837896, -20.68523176094931415 ) ) ;
#20841=CARTESIAN_POINT ( 'NONE',  ( 19.48958755759471728, 3.937961857331544469, -13.19130291127160959 ) ) ;
#20842=CARTESIAN_POINT ( 'NONE',  ( 13.80032290073870449, 8.087308377618120048, -14.09379472307618641 ) ) ;
#20845=CARTESIAN_POINT ( 'NONE',  ( 19.75542110462093959, -4.861139154975066212, -17.07234110396024818 ) ) ;
#20856=CARTESIAN_POINT ( 'NONE',  ( 34.75280465199809043, -13.11698595563971459, -19.00481823564506101 ) ) ;
#20857=CARTESIAN_POINT ( 'NONE',  ( 12.72406076201818870, 7.612173793771704666, -14.95155764689848965 ) ) ;
#20862=CARTESIAN_POINT ( 'NONE',  ( 10.35900481074863322, 16.97049408594186914, -17.87076805301065363 ) ) ;
#20874=CARTESIAN_POINT ( 'NONE',  ( 9.829968513350019421, 15.48396532603707421, -17.81804186139787660 ) ) ;
#20876=CARTESIAN_POINT ( 'NONE',  ( 23.01595892079019379, -1.674233493421072305, -13.97569732891719241 ) ) ;
#20877=CARTESIAN_POINT ( 'NONE',  ( 23.17017814088865535, -4.132587038751921682, -14.65442522582375240 ) ) ;
#20878=CARTESIAN_POINT ( 'NONE',  ( 19.30972751531945519, 5.994221256738944348, -19.84686166629000326 ) ) ;
#20884=CARTESIAN_POINT ( 'NONE',  ( 23.60870351872479844, -7.222488552757559077, -14.83554404960226947 ) ) ;
#20892=CARTESIAN_POINT ( 'NONE',  ( 10.35864924400752862, 16.97212476034085782, -17.91519562840587199 ) ) ;
#20893=CARTESIAN_POINT ( 'NONE',  ( 35.54859390953724585, -22.18451583373416014, -18.19919658220850778 ) ) ;
#20894=CARTESIAN_POINT ( 'NONE',  ( 33.29928106196997817, -12.14339677642331772, -19.64090527578606427 ) ) ;
#20896=CARTESIAN_POINT ( 'NONE',  ( 11.29844335826449964, 8.819016302236921234, -17.20546268888528374 ) ) ;
#20899=CARTESIAN_POINT ( 'NONE',  ( 21.79935899731381710, -1.430375723040585356, -13.25318265510616733 ) ) ;
#20900=CARTESIAN_POINT ( 'NONE',  ( 11.06643561541932463, 17.63888289548684796, -17.56974948598543662 ) ) ;
#20901=CARTESIAN_POINT ( 'NONE',  ( 35.24964364652129234, -20.84149066036063047, -20.16262864730545346 ) ) ;
#20904=CARTESIAN_POINT ( 'NONE',  ( 9.916637298967875935, 16.40639221407973380, -16.50447193873893781 ) ) ;
#20906=CARTESIAN_POINT ( 'NONE',  ( 12.75441094417786658, 7.625102360211175601, -14.92740490885063309 ) ) ;
#20912=CARTESIAN_POINT ( 'NONE',  ( 10.35953768210033665, 16.96805026999784616, -17.84385765891457254 ) ) ;
#20914=CARTESIAN_POINT ( 'NONE',  ( 36.21530066971708095, -20.68720585756345187, -20.37220581101806971 ) ) ;
#20915=CARTESIAN_POINT ( 'NONE',  ( 25.26806593431409453, -8.821542497490490575, -18.05414547114721557 ) ) ;
#20923=CARTESIAN_POINT ( 'NONE',  ( 19.59003110916602708, 6.792398362604423312, -16.15450529561476500 ) ) ;
#20925=CARTESIAN_POINT ( 'NONE',  ( 30.71753525214919378, -10.10955902127019179, -14.92479911117869484 ) ) ;
#20936=CARTESIAN_POINT ( 'NONE',  ( 10.72284644870490489, 16.62177094183959980, -15.95334970537801134 ) ) ;
#20940=CARTESIAN_POINT ( 'NONE',  ( 11.14863080475985591, 10.75631295387255548, -15.99499920034263489 ) ) ;
#20942=CARTESIAN_POINT ( 'NONE',  ( 17.65840769916877662, 9.384080434346836697, -15.74689851229248738 ) ) ;
#20946=CARTESIAN_POINT ( 'NONE',  ( 28.75197783424699693, -9.407057218516385433, -18.70835418409691542 ) ) ;
#20950=CARTESIAN_POINT ( 'NONE',  ( 11.27582353004791216, 16.67860322824865449, -16.78467813988110890 ) ) ;
#20951=CARTESIAN_POINT ( 'NONE',  ( 32.73840480032550460, -11.71477781474665925, -16.63156947497440541 ) ) ;
#20952=CARTESIAN_POINT ( 'NONE',  ( 13.77718166750866224, 8.859676595473322536, -15.39100258941132715 ) ) ;
#20955=CARTESIAN_POINT ( 'NONE',  ( 25.21061150575720333, -3.342243121390650717, -18.67481654970342930 ) ) ;
#20961=CARTESIAN_POINT ( 'NONE',  ( 21.44014932938603835, 4.813297736510089742, -15.98289606589226075 ) ) ;
#20962=CARTESIAN_POINT ( 'NONE',  ( 16.24840684054896656, 4.149509756678782857, -16.79736725456322688 ) ) ;
#20974=CARTESIAN_POINT ( 'NONE',  ( 9.915248083523094280, 16.41276333319327918, -16.50506225043874409 ) ) ;
#20975=CARTESIAN_POINT ( 'NONE',  ( 22.27366892561238387, -0.4200048385588530664, -12.54648181008633934 ) ) ;
#20976=CARTESIAN_POINT ( 'NONE',  ( 23.76385019584477831, -1.264968635605209446, -19.12809044524397351 ) ) ;
#20977=CARTESIAN_POINT ( 'NONE',  ( 36.53927379715840829, -23.14264550581856739, -18.86160504153442830 ) ) ;
#20984=CARTESIAN_POINT ( 'NONE',  ( 15.78240017141095741, 4.038647184180326200, -18.77507866864583619 ) ) ;
#20988=CARTESIAN_POINT ( 'NONE',  ( 10.71678736308702362, 16.64955868083699997, -15.95594379117117434 ) ) ;
#20992=CARTESIAN_POINT ( 'NONE',  ( 16.53304876882650731, 8.555045913257369961, -19.77053526944897754 ) ) ;
#20994=CARTESIAN_POINT ( 'NONE',  ( 24.94601217299843654, -12.81575267032737742, -15.97323768315044035 ) ) ;
#20996=CARTESIAN_POINT ( 'NONE',  ( 34.99076264053043417, -20.67847543353016349, -21.19169145379677488 ) ) ;
#20998=CARTESIAN_POINT ( 'NONE',  ( 20.43449928165676965, -1.849542096390112356, -17.64764676960594869 ) ) ;
#21001=CARTESIAN_POINT ( 'NONE',  ( 18.18682981270212196, 6.389142113859191952, -14.72334701657588063 ) ) ;
#21005=CARTESIAN_POINT ( 'NONE',  ( 30.09709056228524204, -9.598102759715754217, -17.07777997130633807 ) ) ;
#21015=CARTESIAN_POINT ( 'NONE',  ( 36.54859390953724585, -21.18451583373416014, -17.22552805718784441 ) ) ;
#21017=CARTESIAN_POINT ( 'NONE',  ( 9.641485839925177714, 17.66827187890266160, -17.87200850766020110 ) ) ;
#21021=CARTESIAN_POINT ( 'NONE',  ( 10.46722255365007115, 16.47419372244215197, -17.33720764016775462 ) ) ;
#21033=CARTESIAN_POINT ( 'NONE',  ( 10.57561133056755942, 12.06435231892607618, -17.50969232694400546 ) ) ;
#21034=CARTESIAN_POINT ( 'NONE',  ( 25.51539342332723947, -8.447981945391376257, -12.99903862581394876 ) ) ;
#21035=CARTESIAN_POINT ( 'NONE',  ( 23.43490106394649430, 0.5024168867186777909, -19.39616715318824802 ) ) ;
#21037=CARTESIAN_POINT ( 'NONE',  ( 18.12654306171327079, 0.8625984663607378922, -18.09208126113620452 ) ) ;
#21043=CARTESIAN_POINT ( 'NONE',  ( 21.57856661146780652, -4.666631351218505586, -18.28211233923166645 ) ) ;
#21050=CARTESIAN_POINT ( 'NONE',  ( 10.43477690885096720, 16.62299358534909288, -17.37687480348504820 ) ) ;
#21052=CARTESIAN_POINT ( 'NONE',  ( 33.27037009343090546, -12.05169513820189309, -19.60996450177851713 ) ) ;
#21054=CARTESIAN_POINT ( 'NONE',  ( 8.944584764616054784, 16.95159238827779546, -17.91493351301869552 ) ) ;
#21058=CARTESIAN_POINT ( 'NONE',  ( 16.89369580670022941, 0.5033910033923695293, -17.32063897790030893 ) ) ;
#21059=CARTESIAN_POINT ( 'NONE',  ( 11.35716248442908061, 16.30557241515140277, -16.75104082405111683 ) ) ;
#21064=CARTESIAN_POINT ( 'NONE',  ( 9.918725397012197575, 16.39681593027784956, -16.50360835092378409 ) ) ;
#21066=CARTESIAN_POINT ( 'NONE',  ( 10.56508425215480074, 13.43253182900300402, -16.23631622730588830 ) ) ;
#21072=CARTESIAN_POINT ( 'NONE',  ( 10.55304143273637330, 16.08061740358965253, -17.30129946959702281 ) ) ;
#21074=CARTESIAN_POINT ( 'NONE',  ( 32.63927297112797277, -9.624974391992262568, -18.12286679007055312 ) ) ;
#21075=CARTESIAN_POINT ( 'NONE',  ( 27.78884322698630882, -6.380937659459246625, -17.89340433249687834 ) ) ;
#21080=CARTESIAN_POINT ( 'NONE',  ( 33.36027191889437660, -10.38700102556154903, -18.15738432823107473 ) ) ;
#21082=CARTESIAN_POINT ( 'NONE',  ( 19.63213555404020383, 6.204410169219986670, -18.27402551702938638 ) ) ;
#21083=CARTESIAN_POINT ( 'NONE',  ( 27.16844481176636350, -11.11852963900163438, -17.34443814838110143 ) ) ;
#21091=CARTESIAN_POINT ( 'NONE',  ( 10.61946839964472034, 17.09587585246520902, -16.05247762654136068 ) ) ;
#21097=CARTESIAN_POINT ( 'NONE',  ( 11.31072706937237982, 10.01291882189198112, -15.92796669285280764 ) ) ;
#21101=CARTESIAN_POINT ( 'NONE',  ( 17.82019932507133930, 1.781282266713458240, -14.47200660618688417 ) ) ;
#21104=CARTESIAN_POINT ( 'NONE',  ( 25.97851742199650005, -11.98992670343847244, -16.97112261376066655 ) ) ;
#21107=CARTESIAN_POINT ( 'NONE',  ( 11.27605965875426541, 16.67752031190189399, -16.78457976421582742 ) ) ;
#21109=CARTESIAN_POINT ( 'NONE',  ( 33.64261581855389949, -12.62196589562294591, -18.73949555988700055 ) ) ;
#21113=CARTESIAN_POINT ( 'NONE',  ( 24.25137658470242386, -8.936440734373054084, -19.04774169986686161 ) ) ;
#21116=CARTESIAN_POINT ( 'NONE',  ( 21.63689124574611711, 4.661388338709377521, -16.95871344450652174 ) ) ;
#21117=CARTESIAN_POINT ( 'NONE',  ( 16.52347908691095668, 7.282719431485021211, -19.45954596032283845 ) ) ;
#21126=CARTESIAN_POINT ( 'NONE',  ( 9.918725397012197575, 16.39681593027784956, -16.50360835092378409 ) ) ;
#21127=CARTESIAN_POINT ( 'NONE',  ( 21.03482577225312156, -5.582666113748667058, -14.36824825895596014 ) ) ;
#21128=CARTESIAN_POINT ( 'NONE',  ( 20.97149233804390533, -0.06858483505933390956, -19.21322127741759189 ) ) ;
#21130=CARTESIAN_POINT ( 'NONE',  ( 31.86596522828317291, -10.28264332119880820, -18.16914504201997360 ) ) ;
#21133=CARTESIAN_POINT ( 'NONE',  ( 12.50481220565295004, 8.572828783776230921, -15.12633959982445653 ) ) ;
#21138=CARTESIAN_POINT ( 'NONE',  ( 19.20291185354690811, 8.143073066566493878, -16.32372945079811188 ) ) ;
#21140=CARTESIAN_POINT ( 'NONE',  ( 10.35008142444812052, 18.33131885956999696, -17.43324812465761653 ) ) ;
#21144=CARTESIAN_POINT ( 'NONE',  ( 21.66440995182641416, 5.535554982823286174, -17.57621636221614025 ) ) ;
#21145=CARTESIAN_POINT ( 'NONE',  ( 14.69524703049083492, 10.61837011038446654, -14.15659040230468690 ) ) ;
#21147=CARTESIAN_POINT ( 'NONE',  ( 35.54859661768235668, -23.18452799999607805, -18.25366188177437365 ) ) ;
#21148=CARTESIAN_POINT ( 'NONE',  ( 21.08246358516588259, -1.232126404925322438, -18.58940169363586037 ) ) ;
#21149=CARTESIAN_POINT ( 'NONE',  ( 17.81405000127377747, 1.596365152898254980, -17.08637312321770096 ) ) ;
#21150=CARTESIAN_POINT ( 'NONE',  ( 28.29154804861901340, -7.753790107393749409, -19.00671289252072782 ) ) ;
#21158=CARTESIAN_POINT ( 'NONE',  ( 33.19592593216645326, -10.35933293216661610, -17.69446280125821147 ) ) ;
#21159=CARTESIAN_POINT ( 'NONE',  ( 13.19155076956097083, 7.818281081198240834, -14.57899684263624351 ) ) ;
#21167=CARTESIAN_POINT ( 'NONE',  ( 10.53683180627515981, 16.15495681678771689, -17.30800272034635867 ) ) ;
#21177=CARTESIAN_POINT ( 'NONE',  ( 9.667369220937283458, 16.22966640763102220, -17.88537093449073012 ) ) ;
#21179=CARTESIAN_POINT ( 'NONE',  ( 26.12748305362656254, -5.066878407431925524, -14.17679521427828071 ) ) ;
#21180=CARTESIAN_POINT ( 'NONE',  ( 21.81760893248375766, -3.923850722439390815, -13.93537712798182682 ) ) ;
#21185=CARTESIAN_POINT ( 'NONE',  ( 25.73595588610537277, -4.826321120321507507, -18.84379041344559269 ) ) ;
#21192=CARTESIAN_POINT ( 'NONE',  ( 11.86602117609799301, 10.05912493454434120, -16.75833615892761586 ) ) ;
#21194=CARTESIAN_POINT ( 'NONE',  ( 32.57315965809380742, -11.03986597812349935, -18.16622079659612510 ) ) ;
#21195=CARTESIAN_POINT ( 'NONE',  ( 13.37966566800644763, 7.625977406171305262, -15.70782985742499527 ) ) ;
#21200=CARTESIAN_POINT ( 'NONE',  ( 23.16390915794477223, 2.882539813099532555, -14.99485278278146438 ) ) ;
#21202=CARTESIAN_POINT ( 'NONE',  ( 11.27643094638968613, 16.67581753947769130, -16.78442615493024803 ) ) ;
#21207=CARTESIAN_POINT ( 'NONE',  ( 9.641351654859628084, 17.66888726871794191, -17.91235298298990841 ) ) ;
#21209=CARTESIAN_POINT ( 'NONE',  ( 9.916411867603999397, 16.40742607105030260, -16.50456570466356965 ) ) ;
#21216=CARTESIAN_POINT ( 'NONE',  ( 10.47249985125707106, 16.44999136291752251, -17.33460624675630513 ) ) ;
#21218=CARTESIAN_POINT ( 'NONE',  ( 32.68023997084922883, -9.631188006280016367, -18.23865791264771730 ) ) ;
#21219=CARTESIAN_POINT ( 'NONE',  ( 16.68567729567724456, 11.07888045854852876, -16.17353378320854418 ) ) ;
#21220=CARTESIAN_POINT ( 'NONE',  ( 24.36497833745277930, -6.082191617938494055, -18.74521747929614435 ) ) ;
#21223=CARTESIAN_POINT ( 'NONE',  ( 34.49115424338278046, -12.94152926980570939, -19.96804914223585925 ) ) ;
#21225=CARTESIAN_POINT ( 'NONE',  ( 31.88113401528661939, -11.03952345999570639, -14.96145667752709585 ) ) ;
#21226=CARTESIAN_POINT ( 'NONE',  ( 16.53342136567307108, 10.04554801986687629, -15.32032680638607047 ) ) ;
#21238=CARTESIAN_POINT ( 'NONE',  ( 10.70471194873291410, 16.70493807032227451, -15.96226385378574264 ) ) ;
#21244=CARTESIAN_POINT ( 'NONE',  ( 9.916336358462064737, 16.40777236560037622, -16.50459729666445696 ) ) ;
#21245=ORIENTED_EDGE ( 'NONE', *, *, #2895, .F. ) ;
#21246=CARTESIAN_POINT ( 'NONE',  ( 9.667821753224751902, 16.22759103687616999, -17.88509611560606061 ) ) ;
#21248=CARTESIAN_POINT ( 'NONE',  ( 21.18694592818775746, 3.276320881159561438, -13.81383015674761339 ) ) ;
#21251=CARTESIAN_POINT ( 'NONE',  ( 29.46565128511723586, -7.689737916804423534, -14.82739468409561567 ) ) ;
#21254=CARTESIAN_POINT ( 'NONE',  ( 11.27378865171844602, 16.68793543965420767, -16.78556983912737621 ) ) ;
#21256=CARTESIAN_POINT ( 'NONE',  ( 35.54859390953724585, -21.18451583373416014, -17.22552805718784441 ) ) ;
#21257=CARTESIAN_POINT ( 'NONE',  ( 17.54642605795894994, 9.676486402519270058, -18.74681543856335608 ) ) ;
#21259=CARTESIAN_POINT ( 'NONE',  ( 22.23398510282979146, -6.138177547518383292, -17.55864386164050472 ) ) ;
#21262=CARTESIAN_POINT ( 'NONE',  ( 20.29352232415978463, 1.537418251635638944, -14.27211978419980021 ) ) ;
#21263=CARTESIAN_POINT ( 'NONE',  ( 15.22094575638775282, 5.866722348926807662, -16.67377462076821715 ) ) ;
#21275=CARTESIAN_POINT ( 'NONE',  ( 9.924804006935172396, 16.36893865032855899, -16.50109463189289016 ) ) ;
#21276=CARTESIAN_POINT ( 'NONE',  ( 20.97462796522363959, -1.010871063906457534, -12.65628865346789134 ) ) ;
#21277=CARTESIAN_POINT ( 'NONE',  ( 22.98323032518889519, 2.094654362561221284, -17.51695658672324640 ) ) ;
#21279=CARTESIAN_POINT ( 'NONE',  ( 31.96909791962396596, -10.29830001063286460, -18.46063605759182735 ) ) ;
#21286=CARTESIAN_POINT ( 'NONE',  ( 16.01392728624657025, 9.853228751548474662, -15.03783782146776105 ) ) ;
#21289=CARTESIAN_POINT ( 'NONE',  ( 10.71920666609040573, 16.63846344887410922, -15.95486870256106648 ) ) ;
#21296=CARTESIAN_POINT ( 'NONE',  ( 21.48529164538665981, 5.106035544247377267, -18.65531623833433628 ) ) ;
#21298=CARTESIAN_POINT ( 'NONE',  ( 15.41439956623108642, 10.93483300904300215, -14.25553973300288568 ) ) ;
#21300=CARTESIAN_POINT ( 'NONE',  ( 32.57315965809380742, -11.03986597812349935, -18.16622079659612510 ) ) ;
#21301=CARTESIAN_POINT ( 'NONE',  ( 21.34664435287406903, -1.670712410592182895, -14.88600020661825063 ) ) ;
#21302=CARTESIAN_POINT ( 'NONE',  ( 18.08386662754633534, 1.890959213400748684, -17.98613275626550134 ) ) ;
#21303=CARTESIAN_POINT ( 'NONE',  ( 27.67597367917761630, -6.185689562215541670, -12.94745500973225383 ) ) ;
#21313=CARTESIAN_POINT ( 'NONE',  ( 35.14511844984765787, -14.87944403499761670, -19.12340528518704730 ) ) ;
#21314=CARTESIAN_POINT ( 'NONE',  ( 9.641351654859628084, 17.66888726871794191, -17.91235298298990841 ) ) ;
#21318=CARTESIAN_POINT ( 'NONE',  ( 12.02786405831828986, 9.316892843345049968, -16.69140843421181231 ) ) ;
#21330=CARTESIAN_POINT ( 'NONE',  ( 9.667746079407143256, 16.22793808664985704, -17.88513208046981617 ) ) ;
#21334=CARTESIAN_POINT ( 'NONE',  ( 26.63310354640557520, -6.268104337495945977, -18.78393408973622769 ) ) ;
#21335=CARTESIAN_POINT ( 'NONE',  ( 19.55718041265476970, -1.390565517676688900, -17.79492730709450754 ) ) ;
#21339=CARTESIAN_POINT ( 'NONE',  ( 26.47492910780048447, -3.130564378024159211, -15.09640780237150892 ) ) ;
#21350=CARTESIAN_POINT ( 'NONE',  ( 10.47187086816178159, 16.45287595956923354, -17.33486661187913214 ) ) ;
#21352=CARTESIAN_POINT ( 'NONE',  ( 34.82539348385352440, -18.93555941106099993, -20.13934242161363741 ) ) ;
#21355=CARTESIAN_POINT ( 'NONE',  ( 13.37103985619203783, 7.622196798368539028, -15.71470239503888422 ) ) ;
#21358=CARTESIAN_POINT ( 'NONE',  ( 19.02541433733466647, 1.263421280649871248, -13.57496312174407826 ) ) ;
#21359=CARTESIAN_POINT ( 'NONE',  ( 12.83227841057820484, 9.540504573332061256, -16.14102835882348330 ) ) ;
#21362=CARTESIAN_POINT ( 'NONE',  ( 11.47250673971808688, 9.270976631574885829, -15.86106510822916249 ) ) ;
#21364=CARTESIAN_POINT ( 'NONE',  ( 10.17605321708455257, 15.21667774575863419, -16.39719424528293246 ) ) ;
#21369=CARTESIAN_POINT ( 'NONE',  ( 10.35873811938078504, 16.97171716655003593, -17.89325570535168453 ) ) ;
#21371=CARTESIAN_POINT ( 'NONE',  ( 34.01601630636088913, -11.85276864474937852, -20.84012540857256823 ) ) ;
#21372=CARTESIAN_POINT ( 'NONE',  ( 27.11191462667604313, -11.78482644060662743, -13.28705938033944989 ) ) ;
#21373=CARTESIAN_POINT ( 'NONE',  ( 31.59793210864275537, -10.01186915388335485, -14.42687813506083039 ) ) ;
#21380=CARTESIAN_POINT ( 'NONE',  ( 28.35369828010231785, -12.30166555976806464, -13.00196782638265169 ) ) ;
#21382=CARTESIAN_POINT ( 'NONE',  ( 15.73644607668725826, 9.740111719757674535, -14.94734896276200153 ) ) ;
#21396=CARTESIAN_POINT ( 'NONE',  ( 10.72145343393089512, 16.62815948516130504, -15.95392576598924350 ) ) ;
#21402=CARTESIAN_POINT ( 'NONE',  ( 9.924804006935172396, 16.36893865032855899, -16.50109463189289016 ) ) ;
#21404=CARTESIAN_POINT ( 'NONE',  ( 18.10326352236751646, 1.905885860032081158, -14.21403189877281825 ) ) ;
#21407=CARTESIAN_POINT ( 'NONE',  ( 26.08768104250457753, -11.87935956797728210, -17.28510650846989805 ) ) ;
#21410=CARTESIAN_POINT ( 'NONE',  ( 11.27814055543051630, 16.66797705449195988, -16.78371917145281955 ) ) ;
#21412=CARTESIAN_POINT ( 'NONE',  ( 35.19403856461168090, -19.59168648217519504, -19.20845343762490032 ) ) ;
#21413=CARTESIAN_POINT ( 'NONE',  ( 17.96884874826282186, 1.586046385177752871, -19.67104016136476119 ) ) ;
#21416=CARTESIAN_POINT ( 'NONE',  ( 9.068088202150136112, 16.38518988071972871, -17.09785080524718381 ) ) ;
#21417=CARTESIAN_POINT ( 'NONE',  ( 25.72734949418555317, -2.696321649843969936, -17.76569039084671786 ) ) ;
#21420=CARTESIAN_POINT ( 'NONE',  ( 19.23896461120675383, 4.098237937441782996, -14.15247350351863886 ) ) ;
#21421=CARTESIAN_POINT ( 'NONE',  ( 18.03247465133560468, 8.846858265128714649, -18.47062581007826410 ) ) ;
#21434=CARTESIAN_POINT ( 'NONE',  ( 9.641890818133653340, 17.66641459721583374, -17.82828029666912073 ) ) ;
#21435=CARTESIAN_POINT ( 'NONE',  ( 26.86129341093661793, -9.458291044957649163, -14.14057404834478682 ) ) ;
#21436=CARTESIAN_POINT ( 'NONE',  ( 21.34960977245966873, -3.524359730468174412, -18.69795900347392248 ) ) ;
#21437=CARTESIAN_POINT ( 'NONE',  ( 34.86302720852563652, -20.10462780087231138, -21.19305451400748552 ) ) ;
#21443=CARTESIAN_POINT ( 'NONE',  ( 18.69974902744413470, 8.051839821468062652, -15.50866580261103955 ) ) ;
#21444=PRODUCT_DEFINITION_FORMATION_WITH_SPECIFIED_SOURCE ( 'ANY', '', #8864, .NOT_KNOWN. ) ;
#21447=CARTESIAN_POINT ( 'NONE',  ( 10.33816386007038268, 18.38597432894226458, -17.88535571907410571 ) ) ;
#21453=CARTESIAN_POINT ( 'NONE',  ( 17.66155849027303049, 7.702290371990539342, -14.74052880078125760 ) ) ;
#21454=CARTESIAN_POINT ( 'NONE',  ( 18.07402036735202699, 11.65617268414930940, -17.08825885362000108 ) ) ;
#21456=CARTESIAN_POINT ( 'NONE',  ( 33.29928106196997817, -12.14339677642331772, -19.64090527578606427 ) ) ;
#21457=CARTESIAN_POINT ( 'NONE',  ( 21.70429774405079115, -3.429840324723197664, -17.59459576866303365 ) ) ;
#21458=CARTESIAN_POINT ( 'NONE',  ( 18.78845540754137744, 2.550960650414936914, -18.75190108346638951 ) ) ;
#21459=CARTESIAN_POINT ( 'NONE',  ( 25.78329585330208218, -10.67969159757694086, -14.14496057932236361 ) ) ;
#21465=( GEOMETRIC_REPRESENTATION_CONTEXT ( 3 ) GLOBAL_UNCERTAINTY_ASSIGNED_CONTEXT ( ( #29719 ) ) GLOBAL_UNIT_ASSIGNED_CONTEXT ( ( #12587, #857, #4046 ) ) REPRESENTATION_CONTEXT ( 'NONE', 'WORKASPACE' ) );
#21469=CARTESIAN_POINT ( 'NONE',  ( 36.54859390953723874, -21.18451583373416014, -14.99999999999999822 ) ) ;
#21470=CARTESIAN_POINT ( 'NONE',  ( 13.30044262271030142, 7.866402339252101861, -14.49220811360527605 ) ) ;
#21473=CARTESIAN_POINT ( 'NONE',  ( 13.06976498004312326, 8.549601185932660385, -15.95463209657921055 ) ) ;
#21488=CARTESIAN_POINT ( 'NONE',  ( 11.22782251818125232, 9.073501160497098539, -17.23995927586370769 ) ) ;
#21490=CARTESIAN_POINT ( 'NONE',  ( 26.37829838608531219, -4.974601419860719353, -14.31557877768424092 ) ) ;
#21491=CARTESIAN_POINT ( 'NONE',  ( 25.47985489653468605, -2.350970512090694520, -13.88367939857760014 ) ) ;
#21503=CARTESIAN_POINT ( 'NONE',  ( 12.02761088988360783, 9.318053909225662679, -16.69151312802368636 ) ) ;
#21505=FACE_OUTER_BOUND ( 'NONE', #516, .T. ) ;
#21507=CARTESIAN_POINT ( 'NONE',  ( 8.944584683310379702, 16.95159276115599667, -19.66666666666843000 ) ) ;
#21509=CARTESIAN_POINT ( 'NONE',  ( 23.76365953361780470, 2.837943588559999508, -16.54419024451982168 ) ) ;
#21510=CARTESIAN_POINT ( 'NONE',  ( 12.81197645932666163, 9.633610080622574401, -16.14942406932820163 ) ) ;
#21514=CARTESIAN_POINT ( 'NONE',  ( 11.39177520167864266, 9.641221755901229429, -15.89445043910815336 ) ) ;
#21518=CARTESIAN_POINT ( 'NONE',  ( 10.95411528722473626, 11.64838591225006859, -16.07543820933196699 ) ) ;
#21525=CARTESIAN_POINT ( 'NONE',  ( 13.11043623405165448, 8.565188957795726310, -15.92239833454181230 ) ) ;
#21527=CARTESIAN_POINT ( 'NONE',  ( 36.54779501103016770, -22.18092680593016652, -18.48200341583098449 ) ) ;
#21529=CARTESIAN_POINT ( 'NONE',  ( 28.67486520862709654, -7.888541471525570614, -13.83454100519475105 ) ) ;
#21530=CARTESIAN_POINT ( 'NONE',  ( 26.32595758385100382, -12.12905223104374386, -14.21117607008287642 ) ) ;
#21535=CARTESIAN_POINT ( 'NONE',  ( 16.83868323617221208, 3.350830693655540315, -16.91447790370928672 ) ) ;
#21536=CARTESIAN_POINT ( 'NONE',  ( 27.97039215263694345, -10.38370070276099710, -17.82092013489567606 ) ) ;
#21545=CARTESIAN_POINT ( 'NONE',  ( 12.25668235260104844, 9.587403967970216101, -15.31905460325341117 ) ) ;
#21550=CARTESIAN_POINT ( 'NONE',  ( 11.47395765415086188, 9.264374527449886543, -15.86046114005151075 ) ) ;
#21555=CARTESIAN_POINT ( 'NONE',  ( 19.10622122644073428, 3.678778577015775042, -19.67015202264490625 ) ) ;
#21556=DIRECTION ( 'NONE',  ( 0.3331260486002958765, -0.05059491534325381845, -0.9415238660200613285 ) ) ;
#21562=CARTESIAN_POINT ( 'NONE',  ( 11.27239417409149880, 16.69433069180593776, -16.78622300611779750 ) ) ;
#21564=CARTESIAN_POINT ( 'NONE',  ( 33.20927704557755789, -11.78629111679139996, -17.96241082601573424 ) ) ;
#21565=CARTESIAN_POINT ( 'NONE',  ( 14.17177033308128031, 6.273687421093853800, -17.36430109743762173 ) ) ;
#21568=CARTESIAN_POINT ( 'NONE',  ( 23.14387462191455214, -5.292040767005758539, -18.71731562455695297 ) ) ;
#21572=CARTESIAN_POINT ( 'NONE',  ( 19.50876870223950377, -1.661710298099399630, -15.95382585723518432 ) ) ;
#21573=CARTESIAN_POINT ( 'NONE',  ( 15.15242361522499692, 5.855521407460130057, -16.92275779674541170 ) ) ;
#21586=CARTESIAN_POINT ( 'NONE',  ( 11.47181023233108021, 9.274170903235749108, -15.86135313853478657 ) ) ;
#21587=CARTESIAN_POINT ( 'NONE',  ( 27.11308663627701776, -11.54974243744149653, -14.54931088138702933 ) ) ;
#21588=CARTESIAN_POINT ( 'NONE',  ( 21.19231167106929803, 0.1271100694386541607, -19.24388053421374778 ) ) ;
#21589=CARTESIAN_POINT ( 'NONE',  ( 32.77977724007769211, -11.13765286058784554, -18.71157503069099448 ) ) ;
#21597=CARTESIAN_POINT ( 'NONE',  ( 21.66440995182641416, 5.535554982823286174, -17.57621636221614025 ) ) ;
#21601=CARTESIAN_POINT ( 'NONE',  ( 10.71436926824426550, 16.66064837202128501, -15.95707641581892133 ) ) ;
#21605=CARTESIAN_POINT ( 'NONE',  ( 24.66978787416869068, -0.3063955544261361963, -14.42797892638687784 ) ) ;
#21606=CARTESIAN_POINT ( 'NONE',  ( 14.42366234001531922, 7.375548675892134476, -20.85295579936483179 ) ) ;
#21608=CARTESIAN_POINT ( 'NONE',  ( 33.33926371295168423, -12.28475995124076903, -19.67523791759492013 ) ) ;
#21609=CARTESIAN_POINT ( 'NONE',  ( 21.79248024726475563, -3.676524810334697246, -15.28166220873658077 ) ) ;
#21610=CARTESIAN_POINT ( 'NONE',  ( 20.37262416712335167, 4.106476634890254829, -18.27772908839511246 ) ) ;
#21618=CARTESIAN_POINT ( 'NONE',  ( 34.21937970685856101, -11.80343312934236089, -19.83772509046166732 ) ) ;
#21619=CARTESIAN_POINT ( 'NONE',  ( 9.641350810849047548, 17.66889113945805789, -17.92454625180715766 ) ) ;
#21623=CARTESIAN_POINT ( 'NONE',  ( 13.11965390131543430, 8.569119222385459977, -15.91506261175275760 ) ) ;
#21631=CARTESIAN_POINT ( 'NONE',  ( 12.16405474897817207, 7.700086518927777846, -16.63006945039463247 ) ) ;
#21632=CARTESIAN_POINT ( 'NONE',  ( 25.82086518536678454, -3.233603117969178875, -16.21460360555060021 ) ) ;
#21633=CARTESIAN_POINT ( 'NONE',  ( 21.30888034401541731, -0.8953576338359930942, -14.03585182699830369 ) ) ;
#21645=CARTESIAN_POINT ( 'NONE',  ( 10.48820292689142519, 16.37797505638186735, -17.32811247259324716 ) ) ;
#21647=CARTESIAN_POINT ( 'NONE',  ( 33.69611315462438483, -12.86230108826256924, -18.75566652118837752 ) ) ;
#21649=CARTESIAN_POINT ( 'NONE',  ( 13.38606102883407445, 7.628803627606831839, -15.70273264218319120 ) ) ;
#21651=CARTESIAN_POINT ( 'NONE',  ( 25.45462155318426767, -0.2439708902934435431, -15.99927030562601438 ) ) ;
#21652=CARTESIAN_POINT ( 'NONE',  ( 12.79171442625009547, 9.726534347120292523, -16.15780313276466273 ) ) ;
#21656=CARTESIAN_POINT ( 'NONE',  ( 9.919231947839115549, 16.39449282361540483, -16.50339887433786501 ) ) ;
#21659=CARTESIAN_POINT ( 'NONE',  ( 9.919231947839115549, 16.39449282361540483, -16.50339887433786501 ) ) ;
#21664=CARTESIAN_POINT ( 'NONE',  ( 12.26413032053702779, 8.815164712426300397, -16.54932944099246228 ) ) ;
#21666=CARTESIAN_POINT ( 'NONE',  ( 35.12112610261377910, -16.77165912796762726, -21.20079607051596327 ) ) ;
#21667=CARTESIAN_POINT ( 'NONE',  ( 29.30346499805017757, -7.722527705200430859, -14.56292402596598556 ) ) ;
#21668=CARTESIAN_POINT ( 'NONE',  ( 28.75197783424699693, -9.407057218516385433, -18.70835418409691542 ) ) ;
#21672=CARTESIAN_POINT ( 'NONE',  ( 34.28781561389841670, -12.04879923890588422, -19.89451123369701691 ) ) ;
#21675=CARTESIAN_POINT ( 'NONE',  ( 20.54317392443767076, 4.330699614500605144, -17.92201748610454715 ) ) ;
#21676=CARTESIAN_POINT ( 'NONE',  ( 14.33367420948735393, 6.252843122977492563, -16.41390433006782956 ) ) ;
#21689=CARTESIAN_POINT ( 'NONE',  ( 12.26747700539757346, 9.511763647452495363, -15.31658389161178668 ) ) ;
#21694=CARTESIAN_POINT ( 'NONE',  ( 11.47310491742633687, 9.268236560789974376, -15.86081749295074594 ) ) ;
#21696=CARTESIAN_POINT ( 'NONE',  ( 19.61234978942155038, 5.539603999143367652, -15.30853080630118512 ) ) ;
#21702=CARTESIAN_POINT ( 'NONE',  ( 12.83231907764629476, 9.540323555994485005, -16.14101112307237074 ) ) ;
#21704=CARTESIAN_POINT ( 'NONE',  ( 35.46586886002400263, -20.81287600694606610, -19.09165458252410374 ) ) ;
#21705=CARTESIAN_POINT ( 'NONE',  ( 19.05868480923028940, 8.129737193291200370, -16.02886444249750042 ) ) ;
#21708=CARTESIAN_POINT ( 'NONE',  ( 18.35279563442798079, 9.979516425631709708, -19.26739628155305439 ) ) ;
#21712=CARTESIAN_POINT ( 'NONE',  ( 24.68325608809179528, -0.07379305852225118145, -17.41420097001153167 ) ) ;
#21713=CARTESIAN_POINT ( 'NONE',  ( 18.15277384750198308, 2.816914934748806054, -19.48283598520044180 ) ) ;
#21730=CARTESIAN_POINT ( 'NONE',  ( 11.47338783222600789, 9.266948822715743717, -15.86069975447064806 ) ) ;
#21731=CARTESIAN_POINT ( 'NONE',  ( 26.77273401934504093, -11.50074486517209138, -16.59227217106661101 ) ) ;
#21732=CARTESIAN_POINT ( 'NONE',  ( 26.55721583451634160, -2.971036115494387175, -18.36415422809029607 ) ) ;
#21733=CARTESIAN_POINT ( 'NONE',  ( 33.40713826534622655, -12.56408340279653757, -19.71064172033093698 ) ) ;
#21743=CARTESIAN_POINT ( 'NONE',  ( 18.98200677837107264, -2.562081333921657933, -16.63161468174866187 ) ) ;
#21746=CARTESIAN_POINT ( 'NONE',  ( 12.11484812106508713, 10.23787383345373136, -15.37770804730690166 ) ) ;
#21750=CARTESIAN_POINT ( 'NONE',  ( 21.10023079691774228, -0.4353598523292347422, -20.14113737667230097 ) ) ;
#21751=CARTESIAN_POINT ( 'NONE',  ( 19.35412429307980986, 8.340480409601783052, -14.20924892776020343 ) ) ;
#21753=CARTESIAN_POINT ( 'NONE',  ( 34.82539348385352440, -18.93555941106099993, -20.13934242161363741 ) ) ;
#21757=CARTESIAN_POINT ( 'NONE',  ( 28.21504805113574221, -4.147720155524260655, -15.34900075604336500 ) ) ;
#21759=CARTESIAN_POINT ( 'NONE',  ( 18.31666763169264911, 2.112308299563359970, -18.35152529819803746 ) ) ;
#21773=CARTESIAN_POINT ( 'NONE',  ( 36.54859390953724585, -22.18451583373416014, -17.64281456791166036 ) ) ;
#21775=CARTESIAN_POINT ( 'NONE',  ( 9.655099948573186097, 17.60583584124798051, -17.48406748397995614 ) ) ;
#21779=CARTESIAN_POINT ( 'NONE',  ( 13.09695832212169364, 8.559710067821024282, -15.93310406974445392 ) ) ;
#21789=CARTESIAN_POINT ( 'NONE',  ( 11.68823183152383471, 8.106166304734948369, -16.96230016324342671 ) ) ;
#21792=CARTESIAN_POINT ( 'NONE',  ( 30.07451494818246474, -7.670792865742884992, -18.22619146169064663 ) ) ;
#21793=CARTESIAN_POINT ( 'NONE',  ( 24.77705064808911217, -2.604154092221317551, -13.46095375842554098 ) ) ;
#21807=CARTESIAN_POINT ( 'NONE',  ( 10.47249985125707106, 16.44999136291752251, -17.33460624675630513 ) ) ;
#21808=CARTESIAN_POINT ( 'NONE',  ( 33.09970432537804896, -11.76965169494800989, -17.65272085910585886 ) ) ;
#21810=CARTESIAN_POINT ( 'NONE',  ( 9.242255153701981030, 15.58643803978083753, -17.00107889682120899 ) ) ;
#21811=CARTESIAN_POINT ( 'NONE',  ( 23.63863231746517712, -2.790269051896475450, -19.68844555248840678 ) ) ;
#21812=CARTESIAN_POINT ( 'NONE',  ( 12.85347977544317111, 9.515020184875311315, -16.12678873937763413 ) ) ;
#21817=CARTESIAN_POINT ( 'NONE',  ( 11.46775782571576130, 9.292755756535285627, -15.86302895122203616 ) ) ;
#21822=CARTESIAN_POINT ( 'NONE',  ( 12.02908293258818517, 9.311337566433326884, -16.69090174519279657 ) ) ;
#21825=CARTESIAN_POINT ( 'NONE',  ( 35.54910479118309041, -18.69434066908399217, -21.33016376092627553 ) ) ;
#21826=CARTESIAN_POINT ( 'NONE',  ( 28.47856004806874353, -11.16640101040803401, -12.66155532224275149 ) ) ;
#21827=CARTESIAN_POINT ( 'NONE',  ( 13.97862894411929879, 7.467096638697104716, -19.56757695884047621 ) ) ;
#21832=CARTESIAN_POINT ( 'NONE',  ( 35.34711162051457478, -16.78689235204268115, -20.22678452305727603 ) ) ;
#21833=CARTESIAN_POINT ( 'NONE',  ( 20.64697163712990857, 4.580154932681155699, -17.29389188279686707 ) ) ;
#21834=CARTESIAN_POINT ( 'NONE',  ( 16.34386185847872142, 4.569898679961749366, -19.52586945278800812 ) ) ;
#21842=CARTESIAN_POINT ( 'NONE',  ( 12.25826188308600351, 9.517053581970603915, -15.32321445922237224 ) ) ;
#21846=CARTESIAN_POINT ( 'NONE',  ( 12.48484057295006977, 8.564241722236854315, -15.14223913367768759 ) ) ;
#21849=CARTESIAN_POINT ( 'NONE',  ( 10.53902527060216343, 9.639284983934057749, -16.46481883690060144 ) ) ;
#21855=CARTESIAN_POINT ( 'NONE',  ( 12.83225835781710344, 9.540595166069421040, -16.14103675596956933 ) ) ;
#21859=CARTESIAN_POINT ( 'NONE',  ( 34.16485483951214519, -11.28898102658429536, -18.35413676833350038 ) ) ;
#21860=CARTESIAN_POINT ( 'NONE',  ( 17.08157517049449581, 7.460725202527481947, -14.57009041681831896 ) ) ;
#21865=CARTESIAN_POINT ( 'NONE',  ( 18.16551323082808267, 7.152368624112494189, -14.07085781252208712 ) ) ;
#21870=CARTESIAN_POINT ( 'NONE',  ( 19.95076809599375878, -1.008983920988137495, -18.52968236344498720 ) ) ;
#21871=CARTESIAN_POINT ( 'NONE',  ( 21.92347772697934261, 3.537472258236324052, -14.28107661384214211 ) ) ;
#21880=CARTESIAN_POINT ( 'NONE',  ( 10.04637620539468124, 15.81139305134258599, -16.45082025127570091 ) ) ;
#21882=CARTESIAN_POINT ( 'NONE',  ( 25.52642221012979462, -9.988304178644780151, -15.98026830291908773 ) ) ;
#21883=CARTESIAN_POINT ( 'NONE',  ( 24.79209089726652948, -9.725099617967893906, -18.44766554224525734 ) ) ;
#21884=CARTESIAN_POINT ( 'NONE',  ( 32.63711423693117553, -11.05166607373017484, -18.34576405707344549 ) ) ;
#21893=CARTESIAN_POINT ( 'NONE',  ( 15.41431293496917121, 3.575304669039410133, -17.09800041271234150 ) ) ;
#21897=CARTESIAN_POINT ( 'NONE',  ( 11.95275185645256322, 10.98126796543430572, -15.44474055479659569 ) ) ;
#21898=CARTESIAN_POINT ( 'NONE',  ( 33.29928106196997817, -12.14339677642331772, -19.64090527578606427 ) ) ;
#21901=CARTESIAN_POINT ( 'NONE',  ( 24.79644250101478065, -1.608028467720058918, -19.02763285027648976 ) ) ;
#21903=CARTESIAN_POINT ( 'NONE',  ( 17.99875044999096119, -0.3805832805143671838, -17.40611996466761369 ) ) ;
#21905=CARTESIAN_POINT ( 'NONE',  ( 35.13870703111577143, -20.34311121210408757, -20.23074448643712486 ) ) ;
#21908=CARTESIAN_POINT ( 'NONE',  ( 29.43474752111978177, -7.508961153211615169, -12.65842848261850229 ) ) ;
#21909=CARTESIAN_POINT ( 'NONE',  ( 21.04533358917985808, -3.575919577149618167, -19.74844908412899969 ) ) ;
#21911=CARTESIAN_POINT ( 'NONE',  ( 26.32595758385100382, -12.12905223104374386, -14.21117607008287642 ) ) ;
#21918=CARTESIAN_POINT ( 'NONE',  ( 27.31974442496251143, -5.660127319198639206, -14.41990313654811651 ) ) ;
#21920=CARTESIAN_POINT ( 'NONE',  ( 36.02474454408307736, -19.83113812547715682, -20.43161669954002591 ) ) ;
#21922=CARTESIAN_POINT ( 'NONE',  ( 10.95411528722473626, 11.64838591225006859, -16.07543820933196699 ) ) ;
#21925=CARTESIAN_POINT ( 'NONE',  ( 12.35422140817580683, 8.720385185214494683, -16.48779044034850116 ) ) ;
#21939=CARTESIAN_POINT ( 'NONE',  ( 12.82830918206423121, 7.509569466653498004, -16.13756579491948173 ) ) ;
#21941=CARTESIAN_POINT ( 'NONE',  ( 14.35528768574272895, 10.45889919667044410, -14.17515447063821910 ) ) ;
#21943=CARTESIAN_POINT ( 'NONE',  ( 26.64416741123070054, -12.70369174447049332, -17.39020166599120643 ) ) ;
#21946=( BOUNDED_SURFACE ( )  B_SPLINE_SURFACE ( 3, 3, ( 
 ( #20540, #17795, #4226, #29929, #30070, #13675, #23001, #9082, #13075, #22396, #1500, #20835, #19012, #23753, #9846, #9533, #9688, #2250, #20992, #14262, #28219, #2850, #18556, #12136, #5120, #100, #2558, #30218, #28369, #9228, #7424, #403, #16724, #16868, #26044, #4971, #27912, #21453, #16417, #13961, #6971, #19159, #255, #18856, #28515, #7564, #23594, #14413, #4818, #4524, #561, #7268, #9385, #16258, #18711, #13811, #28059, #7112, #16572, #11676, #25571, #25894, #25736, #23141, #11523, #2402, #14114, #4669, #23291, #2693, #23445, #11829, #21144, #11976, #21296, #12431, #15167, #8308, #17172, #8007, #10293, #9988, #3591, #3008, #1159, #14716, #5429, #12583, #3446, #26199, #29117, #24058, #853, #17463, #26812, #5887, #5277, #3158, #24503, #10439, #12882, #22057, #5734, #19601, #22197, #26350, #702, #8158, #21750, #15017, #12736, #19304, #1309, #24347, #28664, #10142, #19455, #10597, #7715, #1016, #17024, #19908, #28825, #29272, #12285, #19748, #14564, #23913, #28971, #21605, #7862, #26501, #5581, #17314, #14864, #24204, #3307, #21901, #26655, #15627, #13041, #11195, #22357, #20506, #13484, #22813, #182, #1917, #18067, #1462, #6627, #29585, #27117, #10753, #2065, #13337, #1763, #11345, #20648, #6483, #29891, #17903, #17613, #8899, #22659, #13193, #20060, #3894, #22964, #22515, #20205, #29742, #24807, #29435, #11050, #8603, #18216, #25252, #15474, #27282, #27571, #6179, #20352, #8457, #26972, #1615, #6030, #10893, #6332, #15920, #15314, #24961, #8748, #27428, #17761, #4337, #24647, #13635, #4041, #15772, #25097, #4188, #3741, #12354, #18937, #14337, #769, #10066, #19378, #18785, #7347, #28742, #3085, #16795, #21529, #21667, #23673, #14787, #7788, #16490, #24127, #12059, #5502, #334, #19087, #26122, #28293, #17097, #16648, #9769, #14641, #25965, #23831, #14193, #3225, #2777, #12503, #5046, #21372, #26422, #21826, #480, #630, #2929, #23519, #9461 ),
 ( #28139, #28438, #7490, #7196, #25816, #4897, #2628, #5200, #11903, #21219, #14494, #9915, #9619, #12209, #19226, #28583, #7637, #16944, #26273, #5355, #23988, #10514, #8228, #19673, #15397, #1539, #27048, #10677, #24578, #22439, #1091, #5657, #13113, #8078, #19986, #8383, #14939, #20133, #29357, #24274, #10368, #17387, #29511, #3373, #5958, #12660, #10822, #21978, #8532, #17242, #24731, #17833, #6256, #15246, #6103, #28900, #26732, #17689, #3666, #27205, #29038, #15551, #24886, #5804, #29191, #26573, #3819, #15089, #3971, #13270, #926, #10218, #19529, #1386, #24425, #7931, #12813, #3520, #22126, #1230, #26894, #12962, #19828, #17538, #22277, #27798, #22894, #16295, #16152, #27644, #18143, #15703, #8830, #27949, #27505, #25177, #4420, #29822, #25032, #6712, #4268, #13850, #2142, #20580, #18598, #25608, #27358, #4118, #6414, #23040, #13568, #25470, #20430, #16000, #13413, #22738, #4704, #29965, #30258, #6556, #1996, #11559, #7006, #11416, #4561, #20721, #20876, #9270, #8972, #23176, #15847, #1851, #11275, #22587, #17986, #11129, #1688, #18287, #25329, #10969, #13714, #2288, #30108, #9118, #20278, #29665, #8680, #6865, #18449, #19191, #23792, #11717, #9879, #14155, #19048, #23634, #19339, #5011, #23483, #13997, #21632, #4854, #14453, #28403, #14300, #2889, #441, #9573, #28704, #12171, #7752, #7457, #28547, #2590, #18896, #28253, #16453, #25776, #7598, #729, #7303, #11866, #23326, #21179, #21490, #290, #12016, #2733, #16760, #16904, #26082, #594, #16608, #25929, #9420, #18745, #21334, #26235, #5315, #14599, #23953, #3044, #17061, #9726, #12316, #5163, #10026, #26389, #2439, #21034, #140, #28093, #7154, #12622, #10640, #19950, #24240, #8351, #5772, #12923, #27015, #3784, #21792, #28865, #15053, #12776, #3341, #3488, #29318, #17653, #26539, #14753, #24091, #3192, #6070, #13080, #15356, #15210, #12469, #1351, #5619, #10479, #24387, #10795, #26697, #14899 ),
 ( #20102, #8043, #1506, #21941, #22093, #1198, #1055, #24695, #22402, #29480, #24543, #29153, #8500, #10331, #10183, #17799, #19639, #3630, #22241, #19494, #5467, #891, #7900, #29005, #17352, #17210, #19788, #8194, #17504, #26857, #5924, #16118, #13238, #11385, #25438, #2255, #1959, #2110, #24849, #13378, #6674, #20546, #4529, #10934, #13819, #27763, #22702, #25139, #22558, #20690, #1657, #30075, #23006, #9088, #9233, #18412, #27611, #20245, #23145, #8794, #6379, #29632, #11528, #22857, #11240, #20841, #30224, #15964, #6829, #27470, #27162, #6221, #29933, #1810, #8644, #11091, #15517, #20393, #29783, #8940, #4085, #17948, #18256, #18108, #3935, #27324, #25002, #6524, #15669, #15814, #25294, #4231, #13531, #4382, #13681, #28064, #4825, #7568, #707, #9537, #410, #2698, #2408, #26203, #23602, #14121, #11683, #23451, #23919, #2562, #21148, #9694, #25741, #20998, #11981, #259, #9850, #5281, #16422, #18864, #23757, #7119, #21301, #23295, #3013, #11836, #12289, #28223, #7274, #16874, #18564, #16576, #19019, #28374, #108, #14569, #25577, #2854, #25900, #4976, #14267, #26049, #27916, #21457, #7428, #16729, #19163, #28520, #21609, #6975, #5128, #16263, #12142, #14417, #566, #4673, #13965, #9390, #18716, #17029, #15322, #12588, #6037, #858, #19607, #17321, #28829, #24508, #10604, #5892, #19754, #3452, #1314, #10148, #14720, #22204, #17178, #29123, #17469, #24063, #29278, #8163, #3164, #19461, #26506, #8314, #12435, #15022, #21757, #19915, #7867, #17619, #26355, #3596, #26978, #24654, #24354, #15173, #7719, #5588, #26819, #12743, #3748, #14869, #13046, #22365, #24209, #8013, #5436, #12889, #3311, #9993, #19308, #28671, #21908, #1022, #10447, #10300, #28978, #26661, #5739, #22062, #1164, #27435, #15778, #25404, #4496, #20512, #6632, #1770, #13787, #25258, #17909, #20656, #1468, #22666, #13491, #25103, #15482, #9047, #8466, #15925, #20212, #10899, #18073, #8906 ),
 ( #6790, #11055, #1620, #10758, #18371, #22523, #1923, #6488, #20357, #11202, #4193, #27288, #16079, #29897, #20066, #22820, #4343, #29593, #6338, #15635, #3901, #13200, #13642, #27728, #24969, #8609, #29442, #4047, #18223, #13342, #29748, #8757, #27577, #22970, #2073, #11350, #30041, #17768, #27124, #6185, #24812, #5093, #9662, #18985, #28341, #7394, #7532, #4641, #23566, #2373, #9354, #18825, #7242, #16692, #23263, #16539, #25863, #73, #26016, #14381, #11646, #23718, #23412, #375, #2820, #21420, #9200, #16233, #2528, #223, #20961, #21116, #12106, #530, #2664, #9501, #19127, #26167, #27884, #25547, #6941, #11943, #14081, #9815, #18680, #4941, #13932, #28028, #5242, #28184, #28484, #7086, #11799, #16837, #23113, #21262, #2222, #11492, #20805, #30191, #14233, #18530, #16381, #25706, #4791, #29237, #9955, #23880, #12399, #3563, #8126, #21870, #26622, #17430, #19423, #19871, #12854, #21572, #8272, #17142, #10567, #5400, #24170, #978, #3126, #29088, #15137, #10412, #24319, #7977, #5849, #14686, #19271, #26780, #21712, #3413, #22025, #28627, #22168, #12704, #7682, #24030, #816, #1275, #16990, #19574, #26315, #24467, #10111, #17584, #670, #26940, #14535, #2979, #28941, #19717, #12255, #28789, #1131, #17287, #7833, #26470, #5554, #14832, #3272, #12548, #10261, #5700, #14982, #29862, #1887, #11168, #18332, #20474, #6451, #20028, #25222, #17869, #15443, #29402, #20625, #1730, #20317, #30004, #9010, #25067, #8872, #6297, #5996, #18186, #11013, #1582, #8426, #22482, #11313, #10862, #8570, #18032, #13158, #17727, #29706, #27248, #27543, #13606, #3864, #15595, #6596, #24772, #8719, #10717, #15284, #20172, #24615, #29553, #24928, #4307, #3710, #4008, #27401, #15742, #27086, #22936, #13006, #15890, #13306, #22627, #4155, #13452, #22325, #2038, #22780, #1429, #6146, #18946, #7354, #20765, #12065, #23373, #11765, #21380, #492, #16497, #2633, #27993, #9777, #21225 ),
 ( #5054, #25516, #7053, #16654, #2783, #7205, #9624, #25823, #25975, #14343, #14044, #28299, #4607, #30154, #23223, #27692, #23082, #9163, #23679, #18492, #13898, #6751, #18791, #16042, #16342, #27846, #25368, #4461, #13752, #11908, #2186, #340, #4903, #11454, #23528, #6908, #2493, #25666, #16199, #18647, #2337, #11607, #20923, #37, #28147, #21082, #4754, #14202, #189, #9322, #9469, #17252, #13243, #3233, #3378, #19235, #23998, #3093, #21535, #636, #12668, #6227, #12363, #7647, #28445, #16951, #19538, #26279, #17104, #28753, #12512, #24282, #21833, #7938, #21675, #9923, #14500, #23838, #7798, #1098, #5664, #14945, #21986, #10375, #3941, #28592, #28907, #5364, #14647, #14795, #938, #19681, #777, #10225, #26581, #10071, #29048, #8084, #19385, #17805, #26430, #27167, #15525, #24854, #5208, #12220, #5515, #24134, #22565, #1663, #19092, #7499, #16800, #26130, #2935, #8801, #11244, #16122, #20398, #25298, #15673, #16266, #25144, #25581, #29787, #27474, #30228, #23298, #1962, #23009, #4386, #25007, #18569, #17953, #25441, #18111, #6527, #27616, #18416, #10942, #13825, #15817, #4237, #2260, #11531, #20845, #20249, #13535, #9239, #4533, #18259, #2116, #23148, #22860, #4676, #27918, #27330, #13967, #20551, #6978, #1814, #29937, #6677, #8943, #29636, #8649, #6832, #20693, #13685, #6384, #11096, #4089, #13382, #15972, #30080, #27771, #22711, #11388, #9091, #28066, #14124, #11839, #28523, #16425, #21303, #25745, #569, #7124, #7574, #9393, #2857, #16878, #5285, #11985, #23760, #111, #21150, #7431, #414, #26205, #4828, #14572, #9854, #262, #14274, #18718, #12147, #23455, #21459, #19167, #23923, #12293, #3016, #16732, #2567, #2412, #16579, #9542, #18867, #11685, #9697, #19021, #21005, #28226, #7277, #25903, #4979, #23605, #2701, #28378, #26055, #5131, #14422, #4774, #25238, #2053, #11473, #28011, #16061, #56, #6615, #1905, #4324, #14066, #25086, #11185 ),
 ( #4623, #18202, #8888, #25388, #6924, #11780, #2358, #27562, #13622, #20942, #9338, #18666, #8738, #15908, #7070, #23244, #6768, #20790, #11629, #22953, #23396, #16365, #6471, #2513, #11333, #25686, #20494, #9031, #4479, #20638, #13915, #29730, #25531, #9183, #23098, #18055, #29880, #4176, #27418, #30021, #18509, #16217, #13470, #15762, #27868, #22800, #18354, #27711, #13770, #2201, #30175, #23548, #3110, #25847, #10090, #7224, #5382, #19404, #26450, #26150, #26298, #18810, #7379, #656, #14518, #28773, #4926, #7816, #21696, #16674, #19112, #16520, #14668, #14218, #24014, #16973, #12384, #3257, #801, #21555, #2651, #17124, #2805, #360, #11926, #5531, #16816, #5225, #14812, #24153, #9940, #21101, #21404, #206, #9486, #23861, #25997, #21248, #5073, #28167, #14366, #23701, #2959, #28320, #9645, #12238, #12086, #18964, #508, #9797, #28467, #7515, #19252, #28609, #7666, #30053, #14247, #25419, #23123, #23578, #18388, #4508, #28199, #21276, #30204, #20975, #23273, #22983, #16554, #15943, #14096, #27743, #6803, #25556, #16397, #8917, #11812, #16092, #13797, #239, #9516, #18838, #18233, #2232, #7255, #2542, #16244, #84, #21127, #11504, #2674, #25878, #25270, #11960, #20820, #4957, #9063, #18540, #4651, #9213, #23429, #27591, #4803, #18696, #2388, #6649, #27894, #13659, #4356, #6956, #28041, #25720, #2086, #11362, #7097, #20666, #13943, #11661, #9365, #2834, #5414, #12120, #12563, #5105, #19585, #16710, #14844, #28954, #5719, #14699, #5564, #28354, #16853, #10125, #24041, #7990, #14395, #17298, #993, #26180, #28644, #26031, #24187, #23737, #3288, #26484, #21882, #12717, #10276, #834, #21435, #26637, #12268, #9828, #546, #14999, #26331, #3140, #24333, #3426, #19435, #388, #686, #9674, #18996, #12415, #5261, #19144, #14549, #7410, #23896, #2993, #21731, #7549, #28501, #28808, #21587, #9973, #19288, #7695, #17008, #7846, #17155, #18010, #25051, #4287 ),
 ( #11434, #6431, #4138, #11147, #22180, #24480, #27379, #6887, #17447, #3578, #20744, #12867, #29684, #16176, #13589, #2160, #22757, #1705, #1143, #10423, #19732, #27666, #30133, #6729, #2016, #29100, #18310, #10988, #27524, #1869, #27820, #13430, #20296, #22039, #9140, #8699, #22913, #6579, #20450, #11295, #8848, #15723, #25497, #20599, #4586, #15867, #16020, #29843, #18163, #25197, #29982, #8992, #25345, #18468, #4437, #13734, #8139, #23061, #26796, #5867, #15149, #23502, #28274, #19071, #7331, #2757, #16472, #4728, #9297, #18622, #2611, #26104, #463, #9750, #28424, #7476, #28567, #25638, #14320, #23351, #163, #9600, #16629, #16779, #14022, #25949, #5029, #21058, #5182, #14476, #2465, #23815, #14175, #21358, #2913, #12193, #10, #7030, #11886, #21200, #11740, #316, #21509, #616, #23656, #18921, #9900, #16925, #27969, #16321, #9442, #12044, #4879, #19210, #18768, #7620, #28121, #26255, #13876, #7180, #23198, #2315, #25799, #11585, #20899, #24562, #7770, #10355, #17083, #17524, #10047, #3652, #21651, #19811, #12948, #10662, #19659, #10499, #3063, #21811, #15072, #29024, #22261, #19361, #1370, #5943, #909, #3358, #750, #29177, #28722, #8213, #1216, #26879, #17676, #15228, #5790, #26406, #19971, #17229, #14768, #5486, #29342, #1076, #8062, #8369, #5340, #24411, #14625, #5643, #23973, #12339, #17373, #10200, #24111, #19513, #3210, #28887, #7919, #26718, #12488, #26556, #3506, #14921, #24261, #12644, #21963, #12798, #22114, #8519, #17820, #2129, #13257, #10955, #11399, #6244, #22576, #15985, #9104, #17972, #8816, #11112, #10811, #4403, #3805, #1981, #15539, #24870, #13398, #4253, #27032, #29948, #3959, #1676, #18273, #27631, #6696, #6088, #20265, #25312, #20565, #4104, #18124, #8957, #29651, #20707, #13702, #13096, #30095, #8667, #23027, #27191, #6399, #22726, #27344, #11262, #15385, #22875, #6542, #20416, #24718, #15690, #25019, #22425, #1830, #29807 ) ),
 .UNSPECIFIED., .T., .F., .F. ) 
 B_SPLINE_SURFACE_WITH_KNOTS ( ( 4, 3, 4 ),
 ( 4, 2, 2, 2, 2, 2, 2, 2, 2, 2, 2, 2, 2, 2, 2, 2, 2, 2, 2, 2, 2, 2, 2, 2, 2, 2, 2, 2, 2, 2, 2, 2, 2, 2, 2, 2, 2, 2, 2, 2, 2, 2, 2, 2, 2, 2, 2, 2, 2, 2, 2, 2, 2, 2, 2, 2, 2, 2, 2, 2, 2, 2, 2, 2, 2, 2, 2, 2, 2, 2, 2, 2, 2, 2, 2, 2, 2, 2, 2, 2, 2, 2, 2, 2, 2, 2, 2, 2, 2, 2, 2, 2, 2, 2, 2, 2, 2, 2, 2, 2, 2, 2, 2, 2, 2, 2, 2, 2, 2, 2, 2, 2, 2, 2, 2, 2, 2, 2, 2, 2, 2, 2, 4 ),
 ( 0.000000000000000000, 0.5000000000000000000, 1.000000000000000000 ),
 ( 0.000000000000000000, 0.007812500000000000000, 0.01464843750000000000, 0.02148437500000000000, 0.02832031250000000000, 0.03515625000000000000, 0.04882812500000000000, 0.05566406250000000000, 0.06250000000000000000, 0.06933593750000000000, 0.07617187500000000000, 0.08984375000000000000, 0.09667968750000000000, 0.1035156250000000000, 0.1103515625000000000, 0.1171875000000000000, 0.1240234375000000000, 0.1308593750000000000, 0.1376953125000000000, 0.1445312500000000000, 0.1513671875000000000, 0.1582031250000000000, 0.1718750000000000000, 0.1787109375000000000, 0.1855468750000000000, 0.1992187500000000000, 0.2060546875000000000, 0.2128906250000000000, 0.2197265625000000000, 0.2265625000000000000, 0.2402343750000000000, 0.2470703125000000000, 0.2539062500000000000, 0.2607421875000000000, 0.2675781250000000000, 0.2812500000000000000, 0.2880859375000000000, 0.2949218750000000000, 0.3017578125000000000, 0.3085937500000000000, 0.3154296875000000000, 0.3222656250000000000, 0.3291015625000000000, 0.3359375000000000000, 0.3496093750000000000, 0.3564453125000000000, 0.3632812500000000000, 0.3701171875000000000, 0.3769531250000000000, 0.3906250000000000000, 0.3974609375000000000, 0.4042968750000000000, 0.4179687500000000000, 0.4316406250000000000, 0.4384765625000000000, 0.4453125000000000000, 0.4521484375000000000, 0.4589843750000000000, 0.4658203125000000000, 0.4726562500000000000, 0.4794921875000000000, 0.4863281250000000000, 0.4931640625000000000, 0.5000000000000000000, 0.5078125000000000000, 0.5156250000000000000, 0.5234375000000000000, 0.5312500000000000000, 0.5390625000000000000, 0.5468750000000000000, 0.5625000000000000000, 0.5693359375000000000, 0.5761718750000000000, 0.5898437500000000000, 0.5966796875000000000, 0.6035156250000000000, 0.6103515625000000000, 0.6171875000000000000, 0.6308593750000000000, 0.6376953125000000000, 0.6445312500000000000, 0.6513671875000000000, 0.6582031250000000000, 0.6718750000000000000, 0.6787109375000000000, 0.6855468750000000000, 0.6992187500000000000, 0.7128906250000000000, 0.7197265625000000000, 0.7265625000000000000, 0.7333984375000000000, 0.7402343750000000000, 0.7470703125000000000, 0.7539062500000000000, 0.7607421875000000000, 0.7675781250000000000, 0.7744140625000000000, 0.7812500000000000000, 0.7890625000000000000, 0.7968750000000000000, 0.8046875000000000000, 0.8125000000000000000, 0.8203125000000000000, 0.8281250000000000000, 0.8437500000000000000, 0.8505859375000000000, 0.8574218750000000000, 0.8710937500000000000, 0.8779296875000000000, 0.8847656250000000000, 0.8916015625000000000, 0.8984375000000000000, 0.9121093750000000000, 0.9189453125000000000, 0.9257812500000000000, 0.9326171875000000000, 0.9394531250000000000, 0.9531250000000000000, 0.9589843750000000000, 0.9648437500000000000, 0.9765625000000000000, 0.9882812500000000000, 1.000000000000000000 ),
 .UNSPECIFIED. ) 
 GEOMETRIC_REPRESENTATION_ITEM ( )  RATIONAL_B_SPLINE_SURFACE ( (
 ( 1.000000000000000000, 1.000000000000000000, 1.000000000000000000, 1.000000000000000000, 1.000000000000000000, 1.000000000000000000, 1.000000000000000000, 1.000000000000000000, 1.000000000000000000, 1.000000000000000000, 1.000000000000000000, 1.000000000000000000, 1.000000000000000000, 1.000000000000000000, 1.000000000000000000, 1.000000000000000000, 1.000000000000000000, 1.000000000000000000, 1.000000000000000000, 1.000000000000000000, 1.000000000000000000, 1.000000000000000000, 1.000000000000000000, 1.000000000000000000, 1.000000000000000000, 1.000000000000000000, 1.000000000000000000, 1.000000000000000000, 1.000000000000000000, 1.000000000000000000, 1.000000000000000000, 1.000000000000000000, 1.000000000000000000, 1.000000000000000000, 1.000000000000000000, 1.000000000000000000, 1.000000000000000000, 1.000000000000000000, 1.000000000000000000, 1.000000000000000000, 1.000000000000000000, 1.000000000000000000, 1.000000000000000000, 1.000000000000000000, 1.000000000000000000, 1.000000000000000000, 1.000000000000000000, 1.000000000000000000, 1.000000000000000000, 1.000000000000000000, 1.000000000000000000, 1.000000000000000000, 1.000000000000000000, 1.000000000000000000, 1.000000000000000000, 1.000000000000000000, 1.000000000000000000, 1.000000000000000000, 1.000000000000000000, 1.000000000000000000, 1.000000000000000000, 1.000000000000000000, 1.000000000000000000, 1.000000000000000000, 1.000000000000000000, 1.000000000000000000, 1.000000000000000000, 1.000000000000000000, 1.000000000000000000, 1.000000000000000000, 1.000000000000000000, 1.000000000000000000, 1.000000000000000000, 1.000000000000000000, 1.000000000000000000, 1.000000000000000000, 1.000000000000000000, 1.000000000000000000, 1.000000000000000000, 1.000000000000000000, 1.000000000000000000, 1.000000000000000000, 1.000000000000000000, 1.000000000000000000, 1.000000000000000000, 1.000000000000000000, 1.000000000000000000, 1.000000000000000000, 1.000000000000000000, 1.000000000000000000, 1.000000000000000000, 1.000000000000000000, 1.000000000000000000, 1.000000000000000000, 1.000000000000000000, 1.000000000000000000, 1.000000000000000000, 1.000000000000000000, 1.000000000000000000, 1.000000000000000000, 1.000000000000000000, 1.000000000000000000, 1.000000000000000000, 1.000000000000000000, 1.000000000000000000, 1.000000000000000000, 1.000000000000000000, 1.000000000000000000, 1.000000000000000000, 1.000000000000000000, 1.000000000000000000, 1.000000000000000000, 1.000000000000000000, 1.000000000000000000, 1.000000000000000000, 1.000000000000000000, 1.000000000000000000, 1.000000000000000000, 1.000000000000000000, 1.000000000000000000, 1.000000000000000000, 1.000000000000000000, 1.000000000000000000, 1.000000000000000000, 1.000000000000000000, 1.000000000000000000, 1.000000000000000000, 1.000000000000000000, 1.000000000000000000, 1.000000000000000000, 1.000000000000000000, 1.000000000000000000, 1.000000000000000000, 1.000000000000000000, 1.000000000000000000, 1.000000000000000000, 1.000000000000000000, 1.000000000000000000, 1.000000000000000000, 1.000000000000000000, 1.000000000000000000, 1.000000000000000000, 1.000000000000000000, 1.000000000000000000, 1.000000000000000000, 1.000000000000000000, 1.000000000000000000, 1.000000000000000000, 1.000000000000000000, 1.000000000000000000, 1.000000000000000000, 1.000000000000000000, 1.000000000000000000, 1.000000000000000000, 1.000000000000000000, 1.000000000000000000, 1.000000000000000000, 1.000000000000000000, 1.000000000000000000, 1.000000000000000000, 1.000000000000000000, 1.000000000000000000, 1.000000000000000000, 1.000000000000000000, 1.000000000000000000, 1.000000000000000000, 1.000000000000000000, 1.000000000000000000, 1.000000000000000000, 1.000000000000000000, 1.000000000000000000, 1.000000000000000000, 1.000000000000000000, 1.000000000000000000, 1.000000000000000000, 1.000000000000000000, 1.000000000000000000, 1.000000000000000000, 1.000000000000000000, 1.000000000000000000, 1.000000000000000000, 1.000000000000000000, 1.000000000000000000, 1.000000000000000000, 1.000000000000000000, 1.000000000000000000, 1.000000000000000000, 1.000000000000000000, 1.000000000000000000, 1.000000000000000000, 1.000000000000000000, 1.000000000000000000, 1.000000000000000000, 1.000000000000000000, 1.000000000000000000, 1.000000000000000000, 1.000000000000000000, 1.000000000000000000, 1.000000000000000000, 1.000000000000000000, 1.000000000000000000, 1.000000000000000000, 1.000000000000000000, 1.000000000000000000, 1.000000000000000000, 1.000000000000000000, 1.000000000000000000, 1.000000000000000000, 1.000000000000000000, 1.000000000000000000, 1.000000000000000000, 1.000000000000000000, 1.000000000000000000, 1.000000000000000000, 1.000000000000000000, 1.000000000000000000, 1.000000000000000000, 1.000000000000000000, 1.000000000000000000, 1.000000000000000000, 1.000000000000000000, 1.000000000000000000, 1.000000000000000000, 1.000000000000000000, 1.000000000000000000, 1.000000000000000000, 1.000000000000000000, 1.000000000000000000, 1.000000000000000000, 1.000000000000000000, 1.000000000000000000, 1.000000000000000000, 1.000000000000000000, 1.000000000000000000, 1.000000000000000000, 1.000000000000000000, 1.000000000000000000, 1.000000000000000000, 1.000000000000000000, 1.000000000000000000, 1.000000000000000000, 1.000000000000000000, 1.000000000000000000, 1.000000000000000000, 1.000000000000000000, 1.000000000000000000),
 ( 0.3333333333333333703, 0.3333333333333333703, 0.3333333333333333703, 0.3333333333333333703, 0.3333333333333333703, 0.3333333333333333703, 0.3333333333333333703, 0.3333333333333333703, 0.3333333333333333703, 0.3333333333333333703, 0.3333333333333333703, 0.3333333333333333703, 0.3333333333333333703, 0.3333333333333333703, 0.3333333333333333703, 0.3333333333333333703, 0.3333333333333333703, 0.3333333333333333703, 0.3333333333333333703, 0.3333333333333333703, 0.3333333333333333703, 0.3333333333333333703, 0.3333333333333333703, 0.3333333333333333703, 0.3333333333333333703, 0.3333333333333333703, 0.3333333333333333703, 0.3333333333333333703, 0.3333333333333333703, 0.3333333333333333703, 0.3333333333333333703, 0.3333333333333333703, 0.3333333333333333703, 0.3333333333333333703, 0.3333333333333333703, 0.3333333333333333703, 0.3333333333333333703, 0.3333333333333333703, 0.3333333333333333703, 0.3333333333333333703, 0.3333333333333333703, 0.3333333333333333703, 0.3333333333333333703, 0.3333333333333333703, 0.3333333333333333703, 0.3333333333333333703, 0.3333333333333333703, 0.3333333333333333703, 0.3333333333333333703, 0.3333333333333333703, 0.3333333333333333703, 0.3333333333333333703, 0.3333333333333333703, 0.3333333333333333703, 0.3333333333333333703, 0.3333333333333333703, 0.3333333333333333703, 0.3333333333333333703, 0.3333333333333333703, 0.3333333333333333703, 0.3333333333333333703, 0.3333333333333333703, 0.3333333333333333703, 0.3333333333333333703, 0.3333333333333333703, 0.3333333333333333703, 0.3333333333333333703, 0.3333333333333333703, 0.3333333333333333703, 0.3333333333333333703, 0.3333333333333333703, 0.3333333333333333703, 0.3333333333333333703, 0.3333333333333333703, 0.3333333333333333703, 0.3333333333333333703, 0.3333333333333333703, 0.3333333333333333703, 0.3333333333333333703, 0.3333333333333333703, 0.3333333333333333703, 0.3333333333333333703, 0.3333333333333333703, 0.3333333333333333703, 0.3333333333333333703, 0.3333333333333333703, 0.3333333333333333703, 0.3333333333333333703, 0.3333333333333333703, 0.3333333333333333703, 0.3333333333333333703, 0.3333333333333333703, 0.3333333333333333703, 0.3333333333333333703, 0.3333333333333333703, 0.3333333333333333703, 0.3333333333333333703, 0.3333333333333333703, 0.3333333333333333703, 0.3333333333333333703, 0.3333333333333333703, 0.3333333333333333703, 0.3333333333333333703, 0.3333333333333333703, 0.3333333333333333703, 0.3333333333333333703, 0.3333333333333333703, 0.3333333333333333703, 0.3333333333333333703, 0.3333333333333333703, 0.3333333333333333703, 0.3333333333333333703, 0.3333333333333333703, 0.3333333333333333703, 0.3333333333333333703, 0.3333333333333333703, 0.3333333333333333703, 0.3333333333333333703, 0.3333333333333333703, 0.3333333333333333703, 0.3333333333333333703, 0.3333333333333333703, 0.3333333333333333703, 0.3333333333333333703, 0.3333333333333333703, 0.3333333333333333703, 0.3333333333333333703, 0.3333333333333333703, 0.3333333333333333703, 0.3333333333333333703, 0.3333333333333333703, 0.3333333333333333703, 0.3333333333333333703, 0.3333333333333333703, 0.3333333333333333703, 0.3333333333333333703, 0.3333333333333333703, 0.3333333333333333703, 0.3333333333333333703, 0.3333333333333333703, 0.3333333333333333703, 0.3333333333333333703, 0.3333333333333333703, 0.3333333333333333703, 0.3333333333333333703, 0.3333333333333333703, 0.3333333333333333703, 0.3333333333333333703, 0.3333333333333333703, 0.3333333333333333703, 0.3333333333333333703, 0.3333333333333333703, 0.3333333333333333703, 0.3333333333333333703, 0.3333333333333333703, 0.3333333333333333703, 0.3333333333333333703, 0.3333333333333333703, 0.3333333333333333703, 0.3333333333333333703, 0.3333333333333333703, 0.3333333333333333703, 0.3333333333333333703, 0.3333333333333333703, 0.3333333333333333703, 0.3333333333333333703, 0.3333333333333333703, 0.3333333333333333703, 0.3333333333333333703, 0.3333333333333333703, 0.3333333333333333703, 0.3333333333333333703, 0.3333333333333333703, 0.3333333333333333703, 0.3333333333333333703, 0.3333333333333333703, 0.3333333333333333703, 0.3333333333333333703, 0.3333333333333333703, 0.3333333333333333703, 0.3333333333333333703, 0.3333333333333333703, 0.3333333333333333703, 0.3333333333333333703, 0.3333333333333333703, 0.3333333333333333703, 0.3333333333333333703, 0.3333333333333333703, 0.3333333333333333703, 0.3333333333333333703, 0.3333333333333333703, 0.3333333333333333703, 0.3333333333333333703, 0.3333333333333333703, 0.3333333333333333703, 0.3333333333333333703, 0.3333333333333333703, 0.3333333333333333703, 0.3333333333333333703, 0.3333333333333333703, 0.3333333333333333703, 0.3333333333333333703, 0.3333333333333333703, 0.3333333333333333703, 0.3333333333333333703, 0.3333333333333333703, 0.3333333333333333703, 0.3333333333333333703, 0.3333333333333333703, 0.3333333333333333703, 0.3333333333333333703, 0.3333333333333333703, 0.3333333333333333703, 0.3333333333333333703, 0.3333333333333333703, 0.3333333333333333703, 0.3333333333333333703, 0.3333333333333333703, 0.3333333333333333703, 0.3333333333333333703, 0.3333333333333333703, 0.3333333333333333703, 0.3333333333333333703, 0.3333333333333333703, 0.3333333333333333703, 0.3333333333333333703, 0.3333333333333333703, 0.3333333333333333703, 0.3333333333333333703, 0.3333333333333333703, 0.3333333333333333703, 0.3333333333333333703, 0.3333333333333333703, 0.3333333333333333703, 0.3333333333333333703, 0.3333333333333333703, 0.3333333333333333703, 0.3333333333333333703, 0.3333333333333333703, 0.3333333333333333703, 0.3333333333333333703, 0.3333333333333333703, 0.3333333333333333703, 0.3333333333333333703, 0.3333333333333333703, 0.3333333333333333703),
 ( 0.3333333333333333703, 0.3333333333333333703, 0.3333333333333333703, 0.3333333333333333703, 0.3333333333333333703, 0.3333333333333333703, 0.3333333333333333703, 0.3333333333333333703, 0.3333333333333333703, 0.3333333333333333703, 0.3333333333333333703, 0.3333333333333333703, 0.3333333333333333703, 0.3333333333333333703, 0.3333333333333333703, 0.3333333333333333703, 0.3333333333333333703, 0.3333333333333333703, 0.3333333333333333703, 0.3333333333333333703, 0.3333333333333333703, 0.3333333333333333703, 0.3333333333333333703, 0.3333333333333333703, 0.3333333333333333703, 0.3333333333333333703, 0.3333333333333333703, 0.3333333333333333703, 0.3333333333333333703, 0.3333333333333333703, 0.3333333333333333703, 0.3333333333333333703, 0.3333333333333333703, 0.3333333333333333703, 0.3333333333333333703, 0.3333333333333333703, 0.3333333333333333703, 0.3333333333333333703, 0.3333333333333333703, 0.3333333333333333703, 0.3333333333333333703, 0.3333333333333333703, 0.3333333333333333703, 0.3333333333333333703, 0.3333333333333333703, 0.3333333333333333703, 0.3333333333333333703, 0.3333333333333333703, 0.3333333333333333703, 0.3333333333333333703, 0.3333333333333333703, 0.3333333333333333703, 0.3333333333333333703, 0.3333333333333333703, 0.3333333333333333703, 0.3333333333333333703, 0.3333333333333333703, 0.3333333333333333703, 0.3333333333333333703, 0.3333333333333333703, 0.3333333333333333703, 0.3333333333333333703, 0.3333333333333333703, 0.3333333333333333703, 0.3333333333333333703, 0.3333333333333333703, 0.3333333333333333703, 0.3333333333333333703, 0.3333333333333333703, 0.3333333333333333703, 0.3333333333333333703, 0.3333333333333333703, 0.3333333333333333703, 0.3333333333333333703, 0.3333333333333333703, 0.3333333333333333703, 0.3333333333333333703, 0.3333333333333333703, 0.3333333333333333703, 0.3333333333333333703, 0.3333333333333333703, 0.3333333333333333703, 0.3333333333333333703, 0.3333333333333333703, 0.3333333333333333703, 0.3333333333333333703, 0.3333333333333333703, 0.3333333333333333703, 0.3333333333333333703, 0.3333333333333333703, 0.3333333333333333703, 0.3333333333333333703, 0.3333333333333333703, 0.3333333333333333703, 0.3333333333333333703, 0.3333333333333333703, 0.3333333333333333703, 0.3333333333333333703, 0.3333333333333333703, 0.3333333333333333703, 0.3333333333333333703, 0.3333333333333333703, 0.3333333333333333703, 0.3333333333333333703, 0.3333333333333333703, 0.3333333333333333703, 0.3333333333333333703, 0.3333333333333333703, 0.3333333333333333703, 0.3333333333333333703, 0.3333333333333333703, 0.3333333333333333703, 0.3333333333333333703, 0.3333333333333333703, 0.3333333333333333703, 0.3333333333333333703, 0.3333333333333333703, 0.3333333333333333703, 0.3333333333333333703, 0.3333333333333333703, 0.3333333333333333703, 0.3333333333333333703, 0.3333333333333333703, 0.3333333333333333703, 0.3333333333333333703, 0.3333333333333333703, 0.3333333333333333703, 0.3333333333333333703, 0.3333333333333333703, 0.3333333333333333703, 0.3333333333333333703, 0.3333333333333333703, 0.3333333333333333703, 0.3333333333333333703, 0.3333333333333333703, 0.3333333333333333703, 0.3333333333333333703, 0.3333333333333333703, 0.3333333333333333703, 0.3333333333333333703, 0.3333333333333333703, 0.3333333333333333703, 0.3333333333333333703, 0.3333333333333333703, 0.3333333333333333703, 0.3333333333333333703, 0.3333333333333333703, 0.3333333333333333703, 0.3333333333333333703, 0.3333333333333333703, 0.3333333333333333703, 0.3333333333333333703, 0.3333333333333333703, 0.3333333333333333703, 0.3333333333333333703, 0.3333333333333333703, 0.3333333333333333703, 0.3333333333333333703, 0.3333333333333333703, 0.3333333333333333703, 0.3333333333333333703, 0.3333333333333333703, 0.3333333333333333703, 0.3333333333333333703, 0.3333333333333333703, 0.3333333333333333703, 0.3333333333333333703, 0.3333333333333333703, 0.3333333333333333703, 0.3333333333333333703, 0.3333333333333333703, 0.3333333333333333703, 0.3333333333333333703, 0.3333333333333333703, 0.3333333333333333703, 0.3333333333333333703, 0.3333333333333333703, 0.3333333333333333703, 0.3333333333333333703, 0.3333333333333333703, 0.3333333333333333703, 0.3333333333333333703, 0.3333333333333333703, 0.3333333333333333703, 0.3333333333333333703, 0.3333333333333333703, 0.3333333333333333703, 0.3333333333333333703, 0.3333333333333333703, 0.3333333333333333703, 0.3333333333333333703, 0.3333333333333333703, 0.3333333333333333703, 0.3333333333333333703, 0.3333333333333333703, 0.3333333333333333703, 0.3333333333333333703, 0.3333333333333333703, 0.3333333333333333703, 0.3333333333333333703, 0.3333333333333333703, 0.3333333333333333703, 0.3333333333333333703, 0.3333333333333333703, 0.3333333333333333703, 0.3333333333333333703, 0.3333333333333333703, 0.3333333333333333703, 0.3333333333333333703, 0.3333333333333333703, 0.3333333333333333703, 0.3333333333333333703, 0.3333333333333333703, 0.3333333333333333703, 0.3333333333333333703, 0.3333333333333333703, 0.3333333333333333703, 0.3333333333333333703, 0.3333333333333333703, 0.3333333333333333703, 0.3333333333333333703, 0.3333333333333333703, 0.3333333333333333703, 0.3333333333333333703, 0.3333333333333333703, 0.3333333333333333703, 0.3333333333333333703, 0.3333333333333333703, 0.3333333333333333703, 0.3333333333333333703, 0.3333333333333333703, 0.3333333333333333703, 0.3333333333333333703, 0.3333333333333333703, 0.3333333333333333703, 0.3333333333333333703, 0.3333333333333333703, 0.3333333333333333703, 0.3333333333333333703, 0.3333333333333333703, 0.3333333333333333703, 0.3333333333333333703, 0.3333333333333333703, 0.3333333333333333703, 0.3333333333333333703, 0.3333333333333333703),
 ( 1.000000000000000000, 1.000000000000000000, 1.000000000000000000, 1.000000000000000000, 1.000000000000000000, 1.000000000000000000, 1.000000000000000000, 1.000000000000000000, 1.000000000000000000, 1.000000000000000000, 1.000000000000000000, 1.000000000000000000, 1.000000000000000000, 1.000000000000000000, 1.000000000000000000, 1.000000000000000000, 1.000000000000000000, 1.000000000000000000, 1.000000000000000000, 1.000000000000000000, 1.000000000000000000, 1.000000000000000000, 1.000000000000000000, 1.000000000000000000, 1.000000000000000000, 1.000000000000000000, 1.000000000000000000, 1.000000000000000000, 1.000000000000000000, 1.000000000000000000, 1.000000000000000000, 1.000000000000000000, 1.000000000000000000, 1.000000000000000000, 1.000000000000000000, 1.000000000000000000, 1.000000000000000000, 1.000000000000000000, 1.000000000000000000, 1.000000000000000000, 1.000000000000000000, 1.000000000000000000, 1.000000000000000000, 1.000000000000000000, 1.000000000000000000, 1.000000000000000000, 1.000000000000000000, 1.000000000000000000, 1.000000000000000000, 1.000000000000000000, 1.000000000000000000, 1.000000000000000000, 1.000000000000000000, 1.000000000000000000, 1.000000000000000000, 1.000000000000000000, 1.000000000000000000, 1.000000000000000000, 1.000000000000000000, 1.000000000000000000, 1.000000000000000000, 1.000000000000000000, 1.000000000000000000, 1.000000000000000000, 1.000000000000000000, 1.000000000000000000, 1.000000000000000000, 1.000000000000000000, 1.000000000000000000, 1.000000000000000000, 1.000000000000000000, 1.000000000000000000, 1.000000000000000000, 1.000000000000000000, 1.000000000000000000, 1.000000000000000000, 1.000000000000000000, 1.000000000000000000, 1.000000000000000000, 1.000000000000000000, 1.000000000000000000, 1.000000000000000000, 1.000000000000000000, 1.000000000000000000, 1.000000000000000000, 1.000000000000000000, 1.000000000000000000, 1.000000000000000000, 1.000000000000000000, 1.000000000000000000, 1.000000000000000000, 1.000000000000000000, 1.000000000000000000, 1.000000000000000000, 1.000000000000000000, 1.000000000000000000, 1.000000000000000000, 1.000000000000000000, 1.000000000000000000, 1.000000000000000000, 1.000000000000000000, 1.000000000000000000, 1.000000000000000000, 1.000000000000000000, 1.000000000000000000, 1.000000000000000000, 1.000000000000000000, 1.000000000000000000, 1.000000000000000000, 1.000000000000000000, 1.000000000000000000, 1.000000000000000000, 1.000000000000000000, 1.000000000000000000, 1.000000000000000000, 1.000000000000000000, 1.000000000000000000, 1.000000000000000000, 1.000000000000000000, 1.000000000000000000, 1.000000000000000000, 1.000000000000000000, 1.000000000000000000, 1.000000000000000000, 1.000000000000000000, 1.000000000000000000, 1.000000000000000000, 1.000000000000000000, 1.000000000000000000, 1.000000000000000000, 1.000000000000000000, 1.000000000000000000, 1.000000000000000000, 1.000000000000000000, 1.000000000000000000, 1.000000000000000000, 1.000000000000000000, 1.000000000000000000, 1.000000000000000000, 1.000000000000000000, 1.000000000000000000, 1.000000000000000000, 1.000000000000000000, 1.000000000000000000, 1.000000000000000000, 1.000000000000000000, 1.000000000000000000, 1.000000000000000000, 1.000000000000000000, 1.000000000000000000, 1.000000000000000000, 1.000000000000000000, 1.000000000000000000, 1.000000000000000000, 1.000000000000000000, 1.000000000000000000, 1.000000000000000000, 1.000000000000000000, 1.000000000000000000, 1.000000000000000000, 1.000000000000000000, 1.000000000000000000, 1.000000000000000000, 1.000000000000000000, 1.000000000000000000, 1.000000000000000000, 1.000000000000000000, 1.000000000000000000, 1.000000000000000000, 1.000000000000000000, 1.000000000000000000, 1.000000000000000000, 1.000000000000000000, 1.000000000000000000, 1.000000000000000000, 1.000000000000000000, 1.000000000000000000, 1.000000000000000000, 1.000000000000000000, 1.000000000000000000, 1.000000000000000000, 1.000000000000000000, 1.000000000000000000, 1.000000000000000000, 1.000000000000000000, 1.000000000000000000, 1.000000000000000000, 1.000000000000000000, 1.000000000000000000, 1.000000000000000000, 1.000000000000000000, 1.000000000000000000, 1.000000000000000000, 1.000000000000000000, 1.000000000000000000, 1.000000000000000000, 1.000000000000000000, 1.000000000000000000, 1.000000000000000000, 1.000000000000000000, 1.000000000000000000, 1.000000000000000000, 1.000000000000000000, 1.000000000000000000, 1.000000000000000000, 1.000000000000000000, 1.000000000000000000, 1.000000000000000000, 1.000000000000000000, 1.000000000000000000, 1.000000000000000000, 1.000000000000000000, 1.000000000000000000, 1.000000000000000000, 1.000000000000000000, 1.000000000000000000, 1.000000000000000000, 1.000000000000000000, 1.000000000000000000, 1.000000000000000000, 1.000000000000000000, 1.000000000000000000, 1.000000000000000000, 1.000000000000000000, 1.000000000000000000, 1.000000000000000000, 1.000000000000000000, 1.000000000000000000, 1.000000000000000000, 1.000000000000000000, 1.000000000000000000, 1.000000000000000000, 1.000000000000000000, 1.000000000000000000, 1.000000000000000000, 1.000000000000000000, 1.000000000000000000, 1.000000000000000000, 1.000000000000000000, 1.000000000000000000, 1.000000000000000000, 1.000000000000000000, 1.000000000000000000, 1.000000000000000000, 1.000000000000000000, 1.000000000000000000),
 ( 0.3333333333333333703, 0.3333333333333333703, 0.3333333333333333703, 0.3333333333333333703, 0.3333333333333333703, 0.3333333333333333703, 0.3333333333333333703, 0.3333333333333333703, 0.3333333333333333703, 0.3333333333333333703, 0.3333333333333333703, 0.3333333333333333703, 0.3333333333333333703, 0.3333333333333333703, 0.3333333333333333703, 0.3333333333333333703, 0.3333333333333333703, 0.3333333333333333703, 0.3333333333333333703, 0.3333333333333333703, 0.3333333333333333703, 0.3333333333333333703, 0.3333333333333333703, 0.3333333333333333703, 0.3333333333333333703, 0.3333333333333333703, 0.3333333333333333703, 0.3333333333333333703, 0.3333333333333333703, 0.3333333333333333703, 0.3333333333333333703, 0.3333333333333333703, 0.3333333333333333703, 0.3333333333333333703, 0.3333333333333333703, 0.3333333333333333703, 0.3333333333333333703, 0.3333333333333333703, 0.3333333333333333703, 0.3333333333333333703, 0.3333333333333333703, 0.3333333333333333703, 0.3333333333333333703, 0.3333333333333333703, 0.3333333333333333703, 0.3333333333333333703, 0.3333333333333333703, 0.3333333333333333703, 0.3333333333333333703, 0.3333333333333333703, 0.3333333333333333703, 0.3333333333333333703, 0.3333333333333333703, 0.3333333333333333703, 0.3333333333333333703, 0.3333333333333333703, 0.3333333333333333703, 0.3333333333333333703, 0.3333333333333333703, 0.3333333333333333703, 0.3333333333333333703, 0.3333333333333333703, 0.3333333333333333703, 0.3333333333333333703, 0.3333333333333333703, 0.3333333333333333703, 0.3333333333333333703, 0.3333333333333333703, 0.3333333333333333703, 0.3333333333333333703, 0.3333333333333333703, 0.3333333333333333703, 0.3333333333333333703, 0.3333333333333333703, 0.3333333333333333703, 0.3333333333333333703, 0.3333333333333333703, 0.3333333333333333703, 0.3333333333333333703, 0.3333333333333333703, 0.3333333333333333703, 0.3333333333333333703, 0.3333333333333333703, 0.3333333333333333703, 0.3333333333333333703, 0.3333333333333333703, 0.3333333333333333703, 0.3333333333333333703, 0.3333333333333333703, 0.3333333333333333703, 0.3333333333333333703, 0.3333333333333333703, 0.3333333333333333703, 0.3333333333333333703, 0.3333333333333333703, 0.3333333333333333703, 0.3333333333333333703, 0.3333333333333333703, 0.3333333333333333703, 0.3333333333333333703, 0.3333333333333333703, 0.3333333333333333703, 0.3333333333333333703, 0.3333333333333333703, 0.3333333333333333703, 0.3333333333333333703, 0.3333333333333333703, 0.3333333333333333703, 0.3333333333333333703, 0.3333333333333333703, 0.3333333333333333703, 0.3333333333333333703, 0.3333333333333333703, 0.3333333333333333703, 0.3333333333333333703, 0.3333333333333333703, 0.3333333333333333703, 0.3333333333333333703, 0.3333333333333333703, 0.3333333333333333703, 0.3333333333333333703, 0.3333333333333333703, 0.3333333333333333703, 0.3333333333333333703, 0.3333333333333333703, 0.3333333333333333703, 0.3333333333333333703, 0.3333333333333333703, 0.3333333333333333703, 0.3333333333333333703, 0.3333333333333333703, 0.3333333333333333703, 0.3333333333333333703, 0.3333333333333333703, 0.3333333333333333703, 0.3333333333333333703, 0.3333333333333333703, 0.3333333333333333703, 0.3333333333333333703, 0.3333333333333333703, 0.3333333333333333703, 0.3333333333333333703, 0.3333333333333333703, 0.3333333333333333703, 0.3333333333333333703, 0.3333333333333333703, 0.3333333333333333703, 0.3333333333333333703, 0.3333333333333333703, 0.3333333333333333703, 0.3333333333333333703, 0.3333333333333333703, 0.3333333333333333703, 0.3333333333333333703, 0.3333333333333333703, 0.3333333333333333703, 0.3333333333333333703, 0.3333333333333333703, 0.3333333333333333703, 0.3333333333333333703, 0.3333333333333333703, 0.3333333333333333703, 0.3333333333333333703, 0.3333333333333333703, 0.3333333333333333703, 0.3333333333333333703, 0.3333333333333333703, 0.3333333333333333703, 0.3333333333333333703, 0.3333333333333333703, 0.3333333333333333703, 0.3333333333333333703, 0.3333333333333333703, 0.3333333333333333703, 0.3333333333333333703, 0.3333333333333333703, 0.3333333333333333703, 0.3333333333333333703, 0.3333333333333333703, 0.3333333333333333703, 0.3333333333333333703, 0.3333333333333333703, 0.3333333333333333703, 0.3333333333333333703, 0.3333333333333333703, 0.3333333333333333703, 0.3333333333333333703, 0.3333333333333333703, 0.3333333333333333703, 0.3333333333333333703, 0.3333333333333333703, 0.3333333333333333703, 0.3333333333333333703, 0.3333333333333333703, 0.3333333333333333703, 0.3333333333333333703, 0.3333333333333333703, 0.3333333333333333703, 0.3333333333333333703, 0.3333333333333333703, 0.3333333333333333703, 0.3333333333333333703, 0.3333333333333333703, 0.3333333333333333703, 0.3333333333333333703, 0.3333333333333333703, 0.3333333333333333703, 0.3333333333333333703, 0.3333333333333333703, 0.3333333333333333703, 0.3333333333333333703, 0.3333333333333333703, 0.3333333333333333703, 0.3333333333333333703, 0.3333333333333333703, 0.3333333333333333703, 0.3333333333333333703, 0.3333333333333333703, 0.3333333333333333703, 0.3333333333333333703, 0.3333333333333333703, 0.3333333333333333703, 0.3333333333333333703, 0.3333333333333333703, 0.3333333333333333703, 0.3333333333333333703, 0.3333333333333333703, 0.3333333333333333703, 0.3333333333333333703, 0.3333333333333333703, 0.3333333333333333703, 0.3333333333333333703, 0.3333333333333333703, 0.3333333333333333703, 0.3333333333333333703, 0.3333333333333333703, 0.3333333333333333703, 0.3333333333333333703, 0.3333333333333333703, 0.3333333333333333703, 0.3333333333333333703, 0.3333333333333333703, 0.3333333333333333703, 0.3333333333333333703, 0.3333333333333333703, 0.3333333333333333703),
 ( 0.3333333333333333703, 0.3333333333333333703, 0.3333333333333333703, 0.3333333333333333703, 0.3333333333333333703, 0.3333333333333333703, 0.3333333333333333703, 0.3333333333333333703, 0.3333333333333333703, 0.3333333333333333703, 0.3333333333333333703, 0.3333333333333333703, 0.3333333333333333703, 0.3333333333333333703, 0.3333333333333333703, 0.3333333333333333703, 0.3333333333333333703, 0.3333333333333333703, 0.3333333333333333703, 0.3333333333333333703, 0.3333333333333333703, 0.3333333333333333703, 0.3333333333333333703, 0.3333333333333333703, 0.3333333333333333703, 0.3333333333333333703, 0.3333333333333333703, 0.3333333333333333703, 0.3333333333333333703, 0.3333333333333333703, 0.3333333333333333703, 0.3333333333333333703, 0.3333333333333333703, 0.3333333333333333703, 0.3333333333333333703, 0.3333333333333333703, 0.3333333333333333703, 0.3333333333333333703, 0.3333333333333333703, 0.3333333333333333703, 0.3333333333333333703, 0.3333333333333333703, 0.3333333333333333703, 0.3333333333333333703, 0.3333333333333333703, 0.3333333333333333703, 0.3333333333333333703, 0.3333333333333333703, 0.3333333333333333703, 0.3333333333333333703, 0.3333333333333333703, 0.3333333333333333703, 0.3333333333333333703, 0.3333333333333333703, 0.3333333333333333703, 0.3333333333333333703, 0.3333333333333333703, 0.3333333333333333703, 0.3333333333333333703, 0.3333333333333333703, 0.3333333333333333703, 0.3333333333333333703, 0.3333333333333333703, 0.3333333333333333703, 0.3333333333333333703, 0.3333333333333333703, 0.3333333333333333703, 0.3333333333333333703, 0.3333333333333333703, 0.3333333333333333703, 0.3333333333333333703, 0.3333333333333333703, 0.3333333333333333703, 0.3333333333333333703, 0.3333333333333333703, 0.3333333333333333703, 0.3333333333333333703, 0.3333333333333333703, 0.3333333333333333703, 0.3333333333333333703, 0.3333333333333333703, 0.3333333333333333703, 0.3333333333333333703, 0.3333333333333333703, 0.3333333333333333703, 0.3333333333333333703, 0.3333333333333333703, 0.3333333333333333703, 0.3333333333333333703, 0.3333333333333333703, 0.3333333333333333703, 0.3333333333333333703, 0.3333333333333333703, 0.3333333333333333703, 0.3333333333333333703, 0.3333333333333333703, 0.3333333333333333703, 0.3333333333333333703, 0.3333333333333333703, 0.3333333333333333703, 0.3333333333333333703, 0.3333333333333333703, 0.3333333333333333703, 0.3333333333333333703, 0.3333333333333333703, 0.3333333333333333703, 0.3333333333333333703, 0.3333333333333333703, 0.3333333333333333703, 0.3333333333333333703, 0.3333333333333333703, 0.3333333333333333703, 0.3333333333333333703, 0.3333333333333333703, 0.3333333333333333703, 0.3333333333333333703, 0.3333333333333333703, 0.3333333333333333703, 0.3333333333333333703, 0.3333333333333333703, 0.3333333333333333703, 0.3333333333333333703, 0.3333333333333333703, 0.3333333333333333703, 0.3333333333333333703, 0.3333333333333333703, 0.3333333333333333703, 0.3333333333333333703, 0.3333333333333333703, 0.3333333333333333703, 0.3333333333333333703, 0.3333333333333333703, 0.3333333333333333703, 0.3333333333333333703, 0.3333333333333333703, 0.3333333333333333703, 0.3333333333333333703, 0.3333333333333333703, 0.3333333333333333703, 0.3333333333333333703, 0.3333333333333333703, 0.3333333333333333703, 0.3333333333333333703, 0.3333333333333333703, 0.3333333333333333703, 0.3333333333333333703, 0.3333333333333333703, 0.3333333333333333703, 0.3333333333333333703, 0.3333333333333333703, 0.3333333333333333703, 0.3333333333333333703, 0.3333333333333333703, 0.3333333333333333703, 0.3333333333333333703, 0.3333333333333333703, 0.3333333333333333703, 0.3333333333333333703, 0.3333333333333333703, 0.3333333333333333703, 0.3333333333333333703, 0.3333333333333333703, 0.3333333333333333703, 0.3333333333333333703, 0.3333333333333333703, 0.3333333333333333703, 0.3333333333333333703, 0.3333333333333333703, 0.3333333333333333703, 0.3333333333333333703, 0.3333333333333333703, 0.3333333333333333703, 0.3333333333333333703, 0.3333333333333333703, 0.3333333333333333703, 0.3333333333333333703, 0.3333333333333333703, 0.3333333333333333703, 0.3333333333333333703, 0.3333333333333333703, 0.3333333333333333703, 0.3333333333333333703, 0.3333333333333333703, 0.3333333333333333703, 0.3333333333333333703, 0.3333333333333333703, 0.3333333333333333703, 0.3333333333333333703, 0.3333333333333333703, 0.3333333333333333703, 0.3333333333333333703, 0.3333333333333333703, 0.3333333333333333703, 0.3333333333333333703, 0.3333333333333333703, 0.3333333333333333703, 0.3333333333333333703, 0.3333333333333333703, 0.3333333333333333703, 0.3333333333333333703, 0.3333333333333333703, 0.3333333333333333703, 0.3333333333333333703, 0.3333333333333333703, 0.3333333333333333703, 0.3333333333333333703, 0.3333333333333333703, 0.3333333333333333703, 0.3333333333333333703, 0.3333333333333333703, 0.3333333333333333703, 0.3333333333333333703, 0.3333333333333333703, 0.3333333333333333703, 0.3333333333333333703, 0.3333333333333333703, 0.3333333333333333703, 0.3333333333333333703, 0.3333333333333333703, 0.3333333333333333703, 0.3333333333333333703, 0.3333333333333333703, 0.3333333333333333703, 0.3333333333333333703, 0.3333333333333333703, 0.3333333333333333703, 0.3333333333333333703, 0.3333333333333333703, 0.3333333333333333703, 0.3333333333333333703, 0.3333333333333333703, 0.3333333333333333703, 0.3333333333333333703, 0.3333333333333333703, 0.3333333333333333703, 0.3333333333333333703, 0.3333333333333333703, 0.3333333333333333703, 0.3333333333333333703, 0.3333333333333333703, 0.3333333333333333703, 0.3333333333333333703, 0.3333333333333333703, 0.3333333333333333703, 0.3333333333333333703, 0.3333333333333333703),
 ( 1.000000000000000000, 1.000000000000000000, 1.000000000000000000, 1.000000000000000000, 1.000000000000000000, 1.000000000000000000, 1.000000000000000000, 1.000000000000000000, 1.000000000000000000, 1.000000000000000000, 1.000000000000000000, 1.000000000000000000, 1.000000000000000000, 1.000000000000000000, 1.000000000000000000, 1.000000000000000000, 1.000000000000000000, 1.000000000000000000, 1.000000000000000000, 1.000000000000000000, 1.000000000000000000, 1.000000000000000000, 1.000000000000000000, 1.000000000000000000, 1.000000000000000000, 1.000000000000000000, 1.000000000000000000, 1.000000000000000000, 1.000000000000000000, 1.000000000000000000, 1.000000000000000000, 1.000000000000000000, 1.000000000000000000, 1.000000000000000000, 1.000000000000000000, 1.000000000000000000, 1.000000000000000000, 1.000000000000000000, 1.000000000000000000, 1.000000000000000000, 1.000000000000000000, 1.000000000000000000, 1.000000000000000000, 1.000000000000000000, 1.000000000000000000, 1.000000000000000000, 1.000000000000000000, 1.000000000000000000, 1.000000000000000000, 1.000000000000000000, 1.000000000000000000, 1.000000000000000000, 1.000000000000000000, 1.000000000000000000, 1.000000000000000000, 1.000000000000000000, 1.000000000000000000, 1.000000000000000000, 1.000000000000000000, 1.000000000000000000, 1.000000000000000000, 1.000000000000000000, 1.000000000000000000, 1.000000000000000000, 1.000000000000000000, 1.000000000000000000, 1.000000000000000000, 1.000000000000000000, 1.000000000000000000, 1.000000000000000000, 1.000000000000000000, 1.000000000000000000, 1.000000000000000000, 1.000000000000000000, 1.000000000000000000, 1.000000000000000000, 1.000000000000000000, 1.000000000000000000, 1.000000000000000000, 1.000000000000000000, 1.000000000000000000, 1.000000000000000000, 1.000000000000000000, 1.000000000000000000, 1.000000000000000000, 1.000000000000000000, 1.000000000000000000, 1.000000000000000000, 1.000000000000000000, 1.000000000000000000, 1.000000000000000000, 1.000000000000000000, 1.000000000000000000, 1.000000000000000000, 1.000000000000000000, 1.000000000000000000, 1.000000000000000000, 1.000000000000000000, 1.000000000000000000, 1.000000000000000000, 1.000000000000000000, 1.000000000000000000, 1.000000000000000000, 1.000000000000000000, 1.000000000000000000, 1.000000000000000000, 1.000000000000000000, 1.000000000000000000, 1.000000000000000000, 1.000000000000000000, 1.000000000000000000, 1.000000000000000000, 1.000000000000000000, 1.000000000000000000, 1.000000000000000000, 1.000000000000000000, 1.000000000000000000, 1.000000000000000000, 1.000000000000000000, 1.000000000000000000, 1.000000000000000000, 1.000000000000000000, 1.000000000000000000, 1.000000000000000000, 1.000000000000000000, 1.000000000000000000, 1.000000000000000000, 1.000000000000000000, 1.000000000000000000, 1.000000000000000000, 1.000000000000000000, 1.000000000000000000, 1.000000000000000000, 1.000000000000000000, 1.000000000000000000, 1.000000000000000000, 1.000000000000000000, 1.000000000000000000, 1.000000000000000000, 1.000000000000000000, 1.000000000000000000, 1.000000000000000000, 1.000000000000000000, 1.000000000000000000, 1.000000000000000000, 1.000000000000000000, 1.000000000000000000, 1.000000000000000000, 1.000000000000000000, 1.000000000000000000, 1.000000000000000000, 1.000000000000000000, 1.000000000000000000, 1.000000000000000000, 1.000000000000000000, 1.000000000000000000, 1.000000000000000000, 1.000000000000000000, 1.000000000000000000, 1.000000000000000000, 1.000000000000000000, 1.000000000000000000, 1.000000000000000000, 1.000000000000000000, 1.000000000000000000, 1.000000000000000000, 1.000000000000000000, 1.000000000000000000, 1.000000000000000000, 1.000000000000000000, 1.000000000000000000, 1.000000000000000000, 1.000000000000000000, 1.000000000000000000, 1.000000000000000000, 1.000000000000000000, 1.000000000000000000, 1.000000000000000000, 1.000000000000000000, 1.000000000000000000, 1.000000000000000000, 1.000000000000000000, 1.000000000000000000, 1.000000000000000000, 1.000000000000000000, 1.000000000000000000, 1.000000000000000000, 1.000000000000000000, 1.000000000000000000, 1.000000000000000000, 1.000000000000000000, 1.000000000000000000, 1.000000000000000000, 1.000000000000000000, 1.000000000000000000, 1.000000000000000000, 1.000000000000000000, 1.000000000000000000, 1.000000000000000000, 1.000000000000000000, 1.000000000000000000, 1.000000000000000000, 1.000000000000000000, 1.000000000000000000, 1.000000000000000000, 1.000000000000000000, 1.000000000000000000, 1.000000000000000000, 1.000000000000000000, 1.000000000000000000, 1.000000000000000000, 1.000000000000000000, 1.000000000000000000, 1.000000000000000000, 1.000000000000000000, 1.000000000000000000, 1.000000000000000000, 1.000000000000000000, 1.000000000000000000, 1.000000000000000000, 1.000000000000000000, 1.000000000000000000, 1.000000000000000000, 1.000000000000000000, 1.000000000000000000, 1.000000000000000000, 1.000000000000000000, 1.000000000000000000, 1.000000000000000000, 1.000000000000000000, 1.000000000000000000, 1.000000000000000000, 1.000000000000000000, 1.000000000000000000, 1.000000000000000000, 1.000000000000000000, 1.000000000000000000, 1.000000000000000000, 1.000000000000000000, 1.000000000000000000, 1.000000000000000000, 1.000000000000000000, 1.000000000000000000, 1.000000000000000000, 1.000000000000000000, 1.000000000000000000) ) ) 
 REPRESENTATION_ITEM ( '' )  SURFACE ( )  );
#21957=CARTESIAN_POINT ( 'NONE',  ( 12.26413032053702779, 8.815164712426300397, -16.54932944099246228 ) ) ;
#21959=CARTESIAN_POINT ( 'NONE',  ( 33.26400919001463308, -11.80307911188568148, -18.11217348381727632 ) ) ;
#21962=CARTESIAN_POINT ( 'NONE',  ( 9.116630548627156827, 16.16256849206635238, -17.05302909012592494 ) ) ;
#21963=CARTESIAN_POINT ( 'NONE',  ( 27.51942754507220812, -5.605608590038333006, -14.64806962472005658 ) ) ;
#21964=CARTESIAN_POINT ( 'NONE',  ( 12.79981923948071554, 9.689364640521217709, -16.15445150739013158 ) ) ;
#21970=CARTESIAN_POINT ( 'NONE',  ( 11.48043977940431226, 9.236673419044803879, -15.85762597608872326 ) ) ;
#21976=CARTESIAN_POINT ( 'NONE',  ( 12.50603416232391929, 8.608717614871036261, -16.38042650914619358 ) ) ;
#21978=CARTESIAN_POINT ( 'NONE',  ( 19.05076746314986025, 7.350425291474770084, -20.38782652337943446 ) ) ;
#21979=CARTESIAN_POINT ( 'NONE',  ( 25.79824969357368047, -12.24460132778619226, -15.92960863319586906 ) ) ;
#21986=CARTESIAN_POINT ( 'NONE',  ( 18.78845540754137744, 2.550960650414936914, -18.75190108346638951 ) ) ;
#21988=CARTESIAN_POINT ( 'NONE',  ( 15.46244301724551740, 3.702889819443702990, -17.82701508041758842 ) ) ;
#22000=CARTESIAN_POINT ( 'NONE',  ( 11.36920530384750805, 13.65748684056475426, -15.68605758175906040 ) ) ;
#22007=CARTESIAN_POINT ( 'NONE',  ( 12.50016782010997751, 8.570776461014483871, -15.13004124836345632 ) ) ;
#22009=CARTESIAN_POINT ( 'NONE',  ( 10.67335300198236148, 9.023663108408856104, -16.40923739229002010 ) ) ;
#22010=DIRECTION ( 'NONE',  ( -0.06678507476159963041, 0.9947851038922184141, -0.07708664516786083165 ) ) ;
#22015=CARTESIAN_POINT ( 'NONE',  ( 12.86479781618563045, 9.514843269526567227, -16.11816302316177030 ) ) ;
#22016=CARTESIAN_POINT ( 'NONE',  ( 34.66364242521329686, -12.71642730124038501, -18.97786663347613256 ) ) ;
#22017=CARTESIAN_POINT ( 'NONE',  ( 18.88762249820254624, 5.002188274287570735, -13.90571046850145542 ) ) ;
#22021=CARTESIAN_POINT ( 'NONE',  ( 14.73435313093308174, 9.569269045654692718, -13.91804818168885305 ) ) ;
#22025=CARTESIAN_POINT ( 'NONE',  ( 24.38930386813997586, -0.5518329404549096040, -18.38842912410832753 ) ) ;
#22026=CARTESIAN_POINT ( 'NONE',  ( 22.65897993816424716, 3.718266075228530365, -15.21131701836175232 ) ) ;
#22038=CARTESIAN_POINT ( 'NONE',  ( 11.48043977940431226, 9.236673419044803879, -15.85762597608872326 ) ) ;
#22039=CARTESIAN_POINT ( 'NONE',  ( 15.93484470893836935, 6.939319753835953009, -14.67888072223970752 ) ) ;
#22040=CARTESIAN_POINT ( 'NONE',  ( 22.68884594494833706, -6.762261587817247843, -18.56982216542981234 ) ) ;
#22050=CARTESIAN_POINT ( 'NONE',  ( 21.58242789233717573, 5.264303332692052528, -18.32037006577847293 ) ) ;
#22054=CARTESIAN_POINT ( 'NONE',  ( 12.27664511671607883, 9.495749246718952818, -15.31080714918738295 ) ) ;
#22057=CARTESIAN_POINT ( 'NONE',  ( 23.66272512268759343, 2.894330346666426745, -16.12005855839824520 ) ) ;
#22059=CARTESIAN_POINT ( 'NONE',  ( 19.52525132842032107, 6.402381508982842639, -20.74126646842140431 ) ) ;
#22062=CARTESIAN_POINT ( 'NONE',  ( 31.07149168920019733, -7.992644923617350905, -17.88177209202816087 ) ) ;
#22064=CARTESIAN_POINT ( 'NONE',  ( 25.07021298685211619, 1.093672866225363638, -16.25732641482299812 ) ) ;
#22066=CARTESIAN_POINT ( 'NONE',  ( 27.89048517759004753, -11.43816616845083445, -12.79876095355805177 ) ) ;
#22077=CARTESIAN_POINT ( 'NONE',  ( 17.83091951040035283, 10.74857467630938501, -15.40187535130914753 ) ) ;
#22078=CARTESIAN_POINT ( 'NONE',  ( 33.42826320546385688, -10.41623213582910523, -18.33855703361424361 ) ) ;
#22079=CARTESIAN_POINT ( 'NONE',  ( 9.915248083523094280, 16.41276333319327918, -16.50506225043874409 ) ) ;
#22082=CARTESIAN_POINT ( 'NONE',  ( 9.661883061612440926, 16.25482663361732705, -17.94384837343789130 ) ) ;
#22092=CARTESIAN_POINT ( 'NONE',  ( 13.36610298980765776, 7.620062051554192806, -15.71863358442526781 ) ) ;
#22093=CARTESIAN_POINT ( 'NONE',  ( 14.69524703049083492, 10.61837011038446654, -14.15659040230468690 ) ) ;
#22094=CARTESIAN_POINT ( 'NONE',  ( 28.02603357813017482, -6.678172375388682802, -19.11289830413424440 ) ) ;
#22110=CARTESIAN_POINT ( 'NONE',  ( 13.12362514754451759, 8.570858352459396201, -15.91189866610160841 ) ) ;
#22111=CARTESIAN_POINT ( 'NONE',  ( 35.18065281855160720, -20.53155141575438591, -20.22037173032050461 ) ) ;
#22113=CARTESIAN_POINT ( 'NONE',  ( 9.153102208164984432, 15.99530481237056989, -17.03794677594065021 ) ) ;
#22114=CARTESIAN_POINT ( 'NONE',  ( 27.95388715220626707, -5.541385876428546631, -15.41148221666858831 ) ) ;
#22115=CARTESIAN_POINT ( 'NONE',  ( 10.35865266338826984, 16.97210907862488938, -17.91126819201198472 ) ) ;
#22120=CARTESIAN_POINT ( 'NONE',  ( 11.47181023233108021, 9.274170903235749108, -15.86135313853478657 ) ) ;
#22125=CARTESIAN_POINT ( 'NONE',  ( 12.02817646543008934, 9.315460371489308500, -16.69127922251917795 ) ) ;
#22126=CARTESIAN_POINT ( 'NONE',  ( 20.94368124868196901, 3.275021729503806878, -20.72479390824751633 ) ) ;
#22127=CARTESIAN_POINT ( 'NONE',  ( 22.56675539556120924, 5.189497681140571750, -18.50903523470404011 ) ) ;
#22130=CARTESIAN_POINT ( 'NONE',  ( 35.98907965336992731, -19.67091466371804742, -20.42083605867238205 ) ) ;
#22132=CARTESIAN_POINT ( 'NONE',  ( 16.89609864265585060, 4.102175112930991574, -14.31125941877678720 ) ) ;
#22139=CARTESIAN_POINT ( 'NONE',  ( 35.16668739017224965, -20.46881214373840763, -20.22602438870426766 ) ) ;
#22143=CARTESIAN_POINT ( 'NONE',  ( 12.27549906412561675, 9.499463866199420181, -15.31139863700699344 ) ) ;
#22148=CARTESIAN_POINT ( 'NONE',  ( 12.49899259368311988, 8.570259324921714494, -15.13097775544467005 ) ) ;
#22150=CARTESIAN_POINT ( 'NONE',  ( 10.65857126575392400, 9.091031811597934720, -16.41538236262689310 ) ) ;
#22155=CARTESIAN_POINT ( 'NONE',  ( 12.82413367917259706, 9.577855520724041227, -16.14439663126654523 ) ) ;
#22157=CARTESIAN_POINT ( 'NONE',  ( 34.58206770820681442, -12.34995000336197890, -18.95321163875382453 ) ) ;
#22158=CARTESIAN_POINT ( 'NONE',  ( 22.09544204423535874, -4.864148257255451746, -14.35781331922719772 ) ) ;
#22163=CARTESIAN_POINT ( 'NONE',  ( 13.51621490077814691, 9.019785729699995258, -14.32023381125561556 ) ) ;
#22168=CARTESIAN_POINT ( 'NONE',  ( 23.76385019584477831, -1.264968635605209446, -19.12809044524397351 ) ) ;
#22169=CARTESIAN_POINT ( 'NONE',  ( 22.35455276305805938, 2.055732105393538678, -20.05127887597516434 ) ) ;
#22179=CARTESIAN_POINT ( 'NONE',  ( 11.47219014545126647, 9.272428573238919114, -15.86119603109536058 ) ) ;
#22180=CARTESIAN_POINT ( 'NONE',  ( 15.19603151210977821, 9.502094893032342782, -14.87270315361914896 ) ) ;
#22181=CARTESIAN_POINT ( 'NONE',  ( 25.47985489653468605, -2.350970512090694520, -13.88367939857760014 ) ) ;
#22190=CARTESIAN_POINT ( 'NONE',  ( 18.80472905218952917, 2.352968372735388503, -20.19605574946481497 ) ) ;
#22193=CARTESIAN_POINT ( 'NONE',  ( 12.27687350794345456, 9.494798321042301481, -15.31070534102384251 ) ) ;
#22197=CARTESIAN_POINT ( 'NONE',  ( 23.66601916330066402, 2.199037240492611733, -18.57254039386976885 ) ) ;
#22199=CARTESIAN_POINT ( 'NONE',  ( 20.97270766892557603, 0.7925772802953747753, -14.00178974354743033 ) ) ;
#22201=CARTESIAN_POINT ( 'NONE',  ( 35.54859390953724585, -22.18451583373416014, -18.06010107863414405 ) ) ;
#22204=CARTESIAN_POINT ( 'NONE',  ( 22.59934115267691368, -6.304331921927718518, -14.46034029096162143 ) ) ;
#22206=CARTESIAN_POINT ( 'NONE',  ( 19.83814782303322133, -0.7621604502531613701, -13.87429439740111370 ) ) ;
#22209=CARTESIAN_POINT ( 'NONE',  ( 27.11191462667604313, -11.78482644060662743, -13.28705938033944989 ) ) ;
#22218=CARTESIAN_POINT ( 'NONE',  ( 26.88076058338416274, -6.009164776401831887, -18.61148891559023255 ) ) ;
#22220=CARTESIAN_POINT ( 'NONE',  ( 36.54460969663918490, -22.16661687567949457, -18.62492107750662029 ) ) ;
#22222=CARTESIAN_POINT ( 'NONE',  ( 9.912057827679275235, 16.42739425315605928, -16.50652470164456531 ) ) ;
#22226=CARTESIAN_POINT ( 'NONE',  ( 15.00903923349565972, 9.404056492746565965, -14.40919036548495669 ) ) ;
#22229=CARTESIAN_POINT ( 'NONE',  ( 11.31072706937237982, 10.01291882189198112, -15.92796669285280764 ) ) ;
#22238=CARTESIAN_POINT ( 'NONE',  ( 13.92371455371928590, 7.866402339252101861, -15.27421329262669936 ) ) ;
#22241=CARTESIAN_POINT ( 'NONE',  ( 16.38450301900381945, 9.168174629645104545, -21.04437084800770918 ) ) ;
#22243=CARTESIAN_POINT ( 'NONE',  ( 30.62762753239542590, -8.735908549479720620, -17.37160549233551876 ) ) ;
#22256=CARTESIAN_POINT ( 'NONE',  ( 12.14965596459611774, 8.983642127099937369, -16.62385966901067391 ) ) ;
#22257=CARTESIAN_POINT ( 'NONE',  ( 35.54859390954303677, -22.18451583373416014, -15.55638201429745848 ) ) ;
#22259=CARTESIAN_POINT ( 'NONE',  ( 9.098468484354940600, 16.24586203394349582, -17.06302340752861824 ) ) ;
#22261=CARTESIAN_POINT ( 'NONE',  ( 21.94319337455657859, -4.318501116253552041, -18.82930321547734920 ) ) ;
#22262=CARTESIAN_POINT ( 'NONE',  ( 12.87265939729807762, 9.517981781931423413, -16.11192280467173532 ) ) ;
#22268=CARTESIAN_POINT ( 'NONE',  ( 11.47310491742633687, 9.268236560789974376, -15.86081749295074594 ) ) ;
#22274=CARTESIAN_POINT ( 'NONE',  ( 9.661883107508126400, 16.25482642313383508, -17.91565355200308218 ) ) ;
#22277=CARTESIAN_POINT ( 'NONE',  ( 17.94761415789183445, 0.5003475314714088684, -19.87472444338139965 ) ) ;
#22278=CARTESIAN_POINT ( 'NONE',  ( 17.49129197179432538, 0.06586305242593921971, -19.15772692538415356 ) ) ;
#22285=CARTESIAN_POINT ( 'NONE',  ( 17.08157517049449581, 7.460725202527481947, -14.57009041681831896 ) ) ;
#22290=B_SPLINE_CURVE_WITH_KNOTS ( 'NONE', 3,
 ( #1246, #6427, #29372, #26908, #8245, #1864, #13126, #1556, #11141, #20445, #6273, #1699, #17699, #17400, #20291, #22454, #12980, #17556, #3680, #22751, #22293, #24747, #25047, #15259, #27060, #4132, #26750, #27221, #29678, #15565, #13425, #5820, #10836, #18005, #24588, #5970, #1400, #15106, #12825, #10691, #24438, #8396, #29525, #20004, #24899, #20144, #3983, #8695, #6116, #15413, #8544, #27374, #3533, #22139, #17845, #13728, #157, #9435, #18761, #18158, #6723, #8984, #8844, #16465, #29977, #9289, #13869, #30127, #20893, #11733, #23056, #14169, #28114, #15862, #23495, #11428, #4873, #18305 ),
 .UNSPECIFIED., .F., .F.,
 ( 4, 2, 2, 2, 2, 2, 2, 2, 2, 2, 2, 2, 2, 2, 2, 2, 2, 2, 2, 2, 2, 2, 2, 2, 2, 2, 2, 2, 2, 2, 2, 2, 2, 2, 2, 2, 2, 2, 4 ),
 ( 0.04625696548581515605, 0.1003381136405422785, 0.1505071704608134109, 0.1755916988709489979, 0.1881339630760167636, 0.1944050951785506465, 0.2006762272810845571, 0.2086934065084689038, 0.2167105857358532783, 0.2327449441906219718, 0.2648136611001593588, 0.2968823780096967457, 0.3129167364644654947, 0.3209339156918498137, 0.3289510949192341882, 0.3346579968240730452, 0.3403648987289118466, 0.3517787025385894495, 0.3746063101579446553, 0.4202615253966550668, 0.5115719558740758899, 0.6028823863514967130, 0.6485376015902071245, 0.6713652092095623303, 0.6827790130192399332, 0.6941928168289175360, 0.7036545619149295883, 0.7131163070009416405, 0.7320397971729657449, 0.7698867775170139538, 0.8077337578610620517, 0.8266572480330862671, 0.8361189931190984304, 0.8455807382051104826, 0.8552319420672911399, 0.8648831459294716861, 0.8841855536538327787, 0.9227903691025551858, 1.000000000000000000 ),
 .UNSPECIFIED. ) ;
#22293=CARTESIAN_POINT ( 'NONE',  ( 32.96569147872224903, -11.36116021242123608, -19.12347989294568151 ) ) ;
#22299=CARTESIAN_POINT ( 'NONE',  ( 12.24519447470441413, 9.516128708456710328, -15.33325952276184445 ) ) ;
#22303=FACE_OUTER_BOUND ( 'NONE', #27527, .T. ) ;
#22305=CARTESIAN_POINT ( 'NONE',  ( 10.66464987567688993, 9.063154531648658363, -16.41286864359600983 ) ) ;
#22311=CARTESIAN_POINT ( 'NONE',  ( 10.35864918915110877, 16.97212501191939538, -17.93331994345748370 ) ) ;
#22312=CARTESIAN_POINT ( 'NONE',  ( 35.14511844984765787, -14.87944403499761670, -19.12340528518704730 ) ) ;
#22313=CARTESIAN_POINT ( 'NONE',  ( 23.76365953361780470, 2.837943588559999508, -16.54419024451982168 ) ) ;
#22320=CARTESIAN_POINT ( 'NONE',  ( 13.76974871631934860, 5.358497188706473402, -17.46738557873778674 ) ) ;
#22325=CARTESIAN_POINT ( 'NONE',  ( 27.61484239614359737, -11.78684095324212855, -18.66559939683001446 ) ) ;
#22327=CARTESIAN_POINT ( 'NONE',  ( 19.10622122644073428, 3.678778577015775042, -19.67015202264490625 ) ) ;
#22337=CARTESIAN_POINT ( 'NONE',  ( 11.60705119439842292, 8.210639978236427439, -17.01629833992986462 ) ) ;
#22339=CARTESIAN_POINT ( 'NONE',  ( 10.33811693838771717, 18.38618951776012267, -17.91928203681695564 ) ) ;
#22340=CARTESIAN_POINT ( 'NONE',  ( 23.72517123929712213, -5.798560033841243744, -19.46542475990168342 ) ) ;
#22343=CIRCLE ( 'NONE', #27267, 0.4999999999999986677 ) ;
#22346=CARTESIAN_POINT ( 'NONE',  ( 9.905109554012803130, 16.45925992188944420, -16.51025697316969953 ) ) ;
#22349=CARTESIAN_POINT ( 'NONE',  ( 24.43075134246613800, -6.859861339260811874, -14.00379227226492951 ) ) ;
#22353=CARTESIAN_POINT ( 'NONE',  ( 12.27289197906229745, 9.513064554772155290, -15.31235135250446078 ) ) ;
#22357=CARTESIAN_POINT ( 'NONE',  ( 21.94319337455657859, -4.318501116253552041, -18.82930321547734920 ) ) ;
#22359=CARTESIAN_POINT ( 'NONE',  ( 20.90484242567171691, 8.469164366756103846, -17.19731680296963106 ) ) ;
#22365=CARTESIAN_POINT ( 'NONE',  ( 23.25962485557060688, -10.00107805802020167, -16.29084171305886386 ) ) ;
#22366=CARTESIAN_POINT ( 'NONE',  ( 20.11894618883271946, -4.454955732405634805, -18.36807076737963129 ) ) ;
#22369=CARTESIAN_POINT ( 'NONE',  ( 26.48263329513011755, -12.06126822337667903, -13.95730679897583038 ) ) ;
#22379=CARTESIAN_POINT ( 'NONE',  ( 23.13192804015912785, -6.366449129859712563, -15.65771855518050870 ) ) ;
#22382=CARTESIAN_POINT ( 'NONE',  ( 32.72409873491027099, -9.637868425582460929, -18.36260606011342844 ) ) ;
#22384=CARTESIAN_POINT ( 'NONE',  ( 9.916775705961365261, 16.40575746196480011, -16.50441451066904364 ) ) ;
#22387=CARTESIAN_POINT ( 'NONE',  ( 9.661883061612440926, 16.25482663361732705, -17.92015940598198753 ) ) ;
#22391=CARTESIAN_POINT ( 'NONE',  ( 9.981537699549546616, 16.10875070413535681, -16.47763325427154868 ) ) ;
#22396=CARTESIAN_POINT ( 'NONE',  ( 17.17204249742301059, 10.23148044644768362, -15.96021614775051667 ) ) ;
#22400=CARTESIAN_POINT ( 'NONE',  ( 8.944585198251687075, 16.95159039956950764, -17.91368623377419667 ) ) ;
#22401=CARTESIAN_POINT ( 'NONE',  ( 34.19383894405228830, -12.60584912221051290, -20.92049940795970997 ) ) ;
#22402=CARTESIAN_POINT ( 'NONE',  ( 16.80873327975549003, 11.45062080556171757, -15.01659013532395370 ) ) ;
#22403=CARTESIAN_POINT ( 'NONE',  ( 26.69342817538273138, -7.978421288772274522, -19.59580293194042966 ) ) ;
#22416=CARTESIAN_POINT ( 'NONE',  ( 13.12048998592846871, 8.569482736746577345, -15.91439669260688561 ) ) ;
#22419=CARTESIAN_POINT ( 'NONE',  ( 35.34747194004189907, -20.28098136206135749, -19.25482875754748946 ) ) ;
#22421=CARTESIAN_POINT ( 'NONE',  ( 9.112356771736518368, 16.18216857766665484, -17.05479705382001399 ) ) ;
#22425=CARTESIAN_POINT ( 'NONE',  ( 31.22280883588763700, -10.09333740185288875, -13.86128061636125786 ) ) ;
#22426=CARTESIAN_POINT ( 'NONE',  ( 13.14063544215093948, 9.636405190433555035, -15.89834116682275145 ) ) ;
#22431=CARTESIAN_POINT ( 'NONE',  ( 11.47293561586387867, 9.269010148984008879, -15.86088772249501666 ) ) ;
#22436=CARTESIAN_POINT ( 'NONE',  ( 9.661883061612440926, 16.25482663361732705, -21.33333333332589632 ) ) ;
#22439=CARTESIAN_POINT ( 'NONE',  ( 13.73972855572809060, 6.741564148929986011, -15.48174541850189811 ) ) ;
#22440=CARTESIAN_POINT ( 'NONE',  ( 18.97315296117551497, 8.914538345978252565, -15.07232217507325345 ) ) ;
#22445=CARTESIAN_POINT ( 'NONE',  ( 23.66272512268759343, 2.894330346666426745, -16.12005855839824520 ) ) ;
#22454=CARTESIAN_POINT ( 'NONE',  ( 32.67186286342521839, -11.06527230177895227, -18.43913201350460440 ) ) ;
#22459=VERTEX_POINT ( 'NONE', #5680 ) ;
#22463=CARTESIAN_POINT ( 'NONE',  ( 11.05541531668977662, 17.68942339022145305, -17.93331994345748726 ) ) ;
#22464=CARTESIAN_POINT ( 'NONE',  ( 35.52699606538937616, -23.08748816067360465, -19.11185354855568619 ) ) ;
#22467=CARTESIAN_POINT ( 'NONE',  ( 10.67100603215144794, 9.034109945373653972, -16.41023209856668785 ) ) ;
#22473=CARTESIAN_POINT ( 'NONE',  ( 12.86851577213266928, 9.516150637207879015, -16.11522534726903899 ) ) ;
#22474=CARTESIAN_POINT ( 'NONE',  ( 36.35319451023849524, -20.30668983862152288, -19.44923342519521370 ) ) ;
#22476=CARTESIAN_POINT ( 'NONE',  ( 22.89472691350227507, 1.279074496056108901, -19.72372301458170796 ) ) ;
#22482=CARTESIAN_POINT ( 'NONE',  ( 28.67999647541807207, -5.919990246138143952, -18.25217309140403188 ) ) ;
#22483=CARTESIAN_POINT ( 'NONE',  ( 27.04162508513615393, -6.753966733322825711, -13.61186222264828771 ) ) ;
#22495=CARTESIAN_POINT ( 'NONE',  ( 12.27065153619900961, 7.644304191818388716, -16.55295716654172722 ) ) ;
#22497=CARTESIAN_POINT ( 'NONE',  ( 12.50226005284522657, 8.571700941790735939, -15.12837371066060221 ) ) ;
#22504=CARTESIAN_POINT ( 'NONE',  ( 9.641359250860388030, 17.66885243249017634, -17.90483003768722625 ) ) ;
#22508=CARTESIAN_POINT ( 'NONE',  ( 26.72358035960067824, -3.685970424986596772, -17.59444040205794835 ) ) ;
#22512=CARTESIAN_POINT ( 'NONE',  ( 12.24516416863347956, 9.516115402270077794, -15.33328367062981279 ) ) ;
#22513=CARTESIAN_POINT ( 'NONE',  ( 32.45272648307624053, -11.02157468472264412, -17.82583700188536824 ) ) ;
#22515=CARTESIAN_POINT ( 'NONE',  ( 24.36497833745277930, -6.082191617938494055, -18.74521747929614435 ) ) ;
#22517=CARTESIAN_POINT ( 'NONE',  ( 21.82779397375749753, -0.5565768812632180262, -18.88406021698092729 ) ) ;
#22522=SURFACE_STYLE_USAGE ( .BOTH. , #18370 ) ;
#22523=CARTESIAN_POINT ( 'NONE',  ( 15.84550288711180777, 10.06862660282224731, -14.00251831694083826 ) ) ;
#22524=CARTESIAN_POINT ( 'NONE',  ( 27.48568275346891809, -3.109927088581168952, -18.71928346135984711 ) ) ;
#22527=CARTESIAN_POINT ( 'NONE',  ( 29.72799312938100513, -7.689056491358781997, -15.42978383025728384 ) ) ;
#22537=CARTESIAN_POINT ( 'NONE',  ( 24.00126410897001605, -3.753019607378720757, -14.48453144943877113 ) ) ;
#22538=CARTESIAN_POINT ( 'NONE',  ( 21.44014932938603835, 4.813297736510089742, -15.98289606589226075 ) ) ;
#22539=CARTESIAN_POINT ( 'NONE',  ( 33.21349783521664278, -10.00660656636812007, -19.57461044683394746 ) ) ;
#22541=CARTESIAN_POINT ( 'NONE',  ( 11.47464782381437587, 9.261287281732329291, -15.86016978468419936 ) ) ;
#22544=CARTESIAN_POINT ( 'NONE',  ( 13.17827647522021906, 8.595009676161804890, -15.86834059905992511 ) ) ;
#22548=CARTESIAN_POINT ( 'NONE',  ( 12.50226005284522657, 8.571700941790735939, -15.12837371066060221 ) ) ;
#22556=CARTESIAN_POINT ( 'NONE',  ( 8.945111769380243771, 16.94917547725161810, -17.84906893764549451 ) ) ;
#22557=CARTESIAN_POINT ( 'NONE',  ( 35.65609946332594404, -19.17501105436304343, -21.36250568352834378 ) ) ;
#22558=CARTESIAN_POINT ( 'NONE',  ( 19.52525132842032107, 6.402381508982842639, -20.74126646842140431 ) ) ;
#22559=CARTESIAN_POINT ( 'NONE',  ( 27.15293434934692129, -9.258526923162836653, -12.62629486378885701 ) ) ;
#22565=CARTESIAN_POINT ( 'NONE',  ( 20.30290135898079384, 0.5855005908018823257, -19.57000235946889433 ) ) ;
#22569=FILL_AREA_STYLE_COLOUR ( '', #13121 ) ;
#22571=CARTESIAN_POINT ( 'NONE',  ( 13.11965390131543430, 8.569119222385459977, -15.91506261175275760 ) ) ;
#22572=CARTESIAN_POINT ( 'NONE',  ( 35.54859390954303677, -21.18451583373416014, -15.55638201429745848 ) ) ;
#22573=CARTESIAN_POINT ( 'NONE',  ( 12.74802704355670535, 7.622310320333636646, -14.93249076938322162 ) ) ;
#22576=CARTESIAN_POINT ( 'NONE',  ( 27.21278356834291756, -7.014839303453253905, -18.45691071023835761 ) ) ;
#22577=CARTESIAN_POINT ( 'NONE',  ( 10.35864918915110877, 16.97212501191939538, -17.92015940598198753 ) ) ;
#22586=CARTESIAN_POINT ( 'NONE',  ( 13.12362514754451759, 8.570858352459396201, -15.91189866610160841 ) ) ;
#22587=CARTESIAN_POINT ( 'NONE',  ( 25.07020310977553024, -1.264175079641418398, -16.65545549153034699 ) ) ;
#22588=CARTESIAN_POINT ( 'NONE',  ( 16.15008960989130671, 4.591438144365319829, -20.60273134265763062 ) ) ;
#22593=CARTESIAN_POINT ( 'NONE',  ( 17.36512755686010934, 0.5347363583120325892, -15.24149349723765390 ) ) ;
#22607=CARTESIAN_POINT ( 'NONE',  ( 11.05541533128794107, 17.68942332327241829, -17.91551483529627120 ) ) ;
#22612=CARTESIAN_POINT ( 'NONE',  ( 9.641354186875979337, 17.66887565656821124, -17.90893343548146177 ) ) ;
#22618=CARTESIAN_POINT ( 'NONE',  ( 10.35864919664826900, 16.97212497753646687, -17.91558149794984445 ) ) ;
#22619=CARTESIAN_POINT ( 'NONE',  ( 34.63381380623899020, -13.58242311684542081, -20.01117170570581649 ) ) ;
#22620=CARTESIAN_POINT ( 'NONE',  ( 16.94076125623460527, 0.4124075662712927692, -16.40086227390004936 ) ) ;
#22627=CARTESIAN_POINT ( 'NONE',  ( 28.67543231808702942, -10.82877479041544433, -19.00874469794426602 ) ) ;
#22629=CARTESIAN_POINT ( 'NONE',  ( 28.63860307613198941, -6.423989724335291918, -15.76775560094196749 ) ) ;
#22641=CARTESIAN_POINT ( 'NONE',  ( 13.16425014233558954, 7.550783913790151125, -15.87799427043765021 ) ) ;
#22643=CARTESIAN_POINT ( 'NONE',  ( 10.33811693838771717, 18.38618951776012267, -17.92279151347708677 ) ) ;
#22644=CARTESIAN_POINT ( 'NONE',  ( 29.95311431238071975, -11.57681909846818691, -12.96816900313696230 ) ) ;
#22648=CARTESIAN_POINT ( 'NONE',  ( 9.649959050778257108, 17.62941265384766254, -17.56860460898032628 ) ) ;
#22652=CARTESIAN_POINT ( 'NONE',  ( 25.67262840375075328, -3.322766148301121714, -14.04542551033457798 ) ) ;
#22656=CARTESIAN_POINT ( 'NONE',  ( 11.05541531668977662, 17.68942339022145305, -21.33333333332589632 ) ) ;
#22657=CARTESIAN_POINT ( 'NONE',  ( 34.39741479528305490, -17.01287786994462792, -20.00997473120332515 ) ) ;
#22659=CARTESIAN_POINT ( 'NONE',  ( 26.61709978538234012, -3.831456866606135492, -17.85214630790261836 ) ) ;
#22662=CARTESIAN_POINT ( 'NONE',  ( 21.98307778806466928, -1.383504679822651795, -14.66368364926259460 ) ) ;
#22666=CARTESIAN_POINT ( 'NONE',  ( 26.19910047366428429, -13.48590472426672626, -13.82108881675422829 ) ) ;
#22667=CARTESIAN_POINT ( 'NONE',  ( 27.65280983889778810, -8.379432582749632985, -19.23476105915534973 ) ) ;
#22682=CARTESIAN_POINT ( 'NONE',  ( 27.60672911170952304, -4.775276709060196190, -16.23362067418393195 ) ) ;
#22683=CARTESIAN_POINT ( 'NONE',  ( 19.54522145393098498, 6.247755356217567169, -19.64858106251988801 ) ) ;
#22684=CARTESIAN_POINT ( 'NONE',  ( 35.26378566547066384, -17.41255297500571331, -21.24391863398521352 ) ) ;
#22686=CARTESIAN_POINT ( 'NONE',  ( 12.48484057295006977, 8.564241722236854315, -15.14223913367768759 ) ) ;
#22689=CARTESIAN_POINT ( 'NONE',  ( 13.25994536507779742, 8.631100619704961119, -15.80324905228922994 ) ) ;
#22693=CARTESIAN_POINT ( 'NONE',  ( 12.49860086554322436, 8.570087612320898884, -15.13128986298120537 ) ) ;
#22700=CARTESIAN_POINT ( 'NONE',  ( 13.38095672321806795, 7.626547943635540783, -15.70680086385617358 ) ) ;
#22701=CARTESIAN_POINT ( 'NONE',  ( 34.21167138940940333, -12.68596085309027899, -20.92588972839351058 ) ) ;
#22702=CARTESIAN_POINT ( 'NONE',  ( 20.32371149932726695, 7.300285753667301591, -19.85501735805741319 ) ) ;
#22705=CARTESIAN_POINT ( 'NONE',  ( 17.63088349262504551, 4.212901655933308120, -18.95607689789294170 ) ) ;
#22711=CARTESIAN_POINT ( 'NONE',  ( 23.15972007162554291, -8.148303969466700991, -13.79129035937103431 ) ) ;
#22715=( NAMED_UNIT ( * ) PLANE_ANGLE_UNIT ( ) SI_UNIT ( $, .RADIAN. ) );
#22721=CARTESIAN_POINT ( 'NONE',  ( 32.48803055552120611, -10.90163289162770432, -13.69202896798154256 ) ) ;
#22723=CARTESIAN_POINT ( 'NONE',  ( 10.67054149815029618, 9.036200773601834157, -16.41042721873081689 ) ) ;
#22726=CARTESIAN_POINT ( 'NONE',  ( 25.79824969357368047, -12.24460132778619226, -15.92960863319586906 ) ) ;
#22728=CARTESIAN_POINT ( 'NONE',  ( 10.35864918915110877, 16.97212501191939538, -19.66666666666842644 ) ) ;
#22737=CARTESIAN_POINT ( 'NONE',  ( 13.11714404544056656, 8.568033937426095648, -15.91706119101506545 ) ) ;
#22738=CARTESIAN_POINT ( 'NONE',  ( 19.88518670226333995, -2.923732859705698850, -17.09422515135678111 ) ) ;
#22739=CARTESIAN_POINT ( 'NONE',  ( 17.31888479101057143, -0.09998177899580885930, -18.75936487049801116 ) ) ;
#22745=CARTESIAN_POINT ( 'NONE',  ( 17.33713706444265412, 0.9871066061555996418, -18.79342181739402307 ) ) ;
#22751=CARTESIAN_POINT ( 'NONE',  ( 32.89062095351589932, -11.25267498498577723, -18.96775996542842435 ) ) ;
#22757=CARTESIAN_POINT ( 'NONE',  ( 17.12833724908345800, 9.171387755021909172, -19.38714867094073213 ) ) ;
#22758=CARTESIAN_POINT ( 'NONE',  ( 12.78959314398258940, 9.756708335562493062, -14.89936416525698526 ) ) ;
#22759=CARTESIAN_POINT ( 'NONE',  ( 33.75544676243647757, -14.12885555826641593, -19.81592319558764004 ) ) ;
#22767=CARTESIAN_POINT ( 'NONE',  ( 12.75568354342045119, 7.625663700289499580, -14.92639070443840588 ) ) ;
#22773=CARTESIAN_POINT ( 'NONE',  ( 12.86785267122296794, 9.515866005961482799, -16.11575320936711364 ) ) ;
#22774=CARTESIAN_POINT ( 'NONE',  ( 34.36632712588347260, -12.38074715364594347, -19.93031689919964222 ) ) ;
#22775=CARTESIAN_POINT ( 'NONE',  ( 25.21413058671614849, -1.115224416820481457, -18.44856734933592080 ) ) ;
#22780=CARTESIAN_POINT ( 'NONE',  ( 26.95082352492110189, -12.40836276091286194, -17.97502949936508898 ) ) ;
#22781=CARTESIAN_POINT ( 'NONE',  ( 26.47302276827314671, -6.985584592454325836, -13.42065591321591711 ) ) ;
#22789=CARTESIAN_POINT ( 'NONE',  ( 10.33811693838771717, 18.38618951776012267, -17.98596209335946128 ) ) ;
#22796=CARTESIAN_POINT ( 'NONE',  ( 9.641350810849047548, 17.66889113945805789, -17.97192418671891190 ) ) ;
#22800=CARTESIAN_POINT ( 'NONE',  ( 18.80816768961129881, 6.772028514247487863, -18.23967922641782380 ) ) ;
#22804=CARTESIAN_POINT ( 'NONE',  ( 23.77086030874127687, -7.150112426529108944, -14.59934731766091431 ) ) ;
#22808=CARTESIAN_POINT ( 'NONE',  ( 12.46291758456249354, 9.612344561400664844, -15.15973035232449462 ) ) ;
#22811=CARTESIAN_POINT ( 'NONE',  ( 35.54859390953724585, -22.18451583373416014, -17.99055332684694974 ) ) ;
#22813=CARTESIAN_POINT ( 'NONE',  ( 21.16681283796276603, -5.103637247178538061, -17.00692323485822754 ) ) ;
#22815=CARTESIAN_POINT ( 'NONE',  ( 23.33644427035094537, 1.513498076802863190, -16.07814869553001103 ) ) ;
#22818=CIRCLE ( 'NONE', #15014, 0.5000000000000004441 ) ;
#22819=SHAPE_REPRESENTATION ( 'Pedal Return Coil Spring', ( #13190 ), #21465 ) ;
#22820=CARTESIAN_POINT ( 'NONE',  ( 18.00441060066494003, 9.543425513107552050, -19.87907960298149490 ) ) ;
#22821=CARTESIAN_POINT ( 'NONE',  ( 27.90801785101615096, -12.26699769840798204, -14.39122685649866717 ) ) ;
#22833=CARTESIAN_POINT ( 'NONE',  ( 25.04368804655567970, -3.332730676350641463, -14.85212872609148427 ) ) ;
#22834=CARTESIAN_POINT ( 'NONE',  ( 16.95656709563420250, 3.789241241613106048, -19.64973185778705655 ) ) ;
#22836=CARTESIAN_POINT ( 'NONE',  ( 34.19383894405228830, -12.60584912221051290, -20.92049940795970997 ) ) ;
#22839=CARTESIAN_POINT ( 'NONE',  ( 11.47257016429183452, 9.270685755423764718, -15.86103888016343255 ) ) ;
#22844=CARTESIAN_POINT ( 'NONE',  ( 9.663058643182488083, 16.24943526668553062, -17.89776827055807118 ) ) ;
#22848=CARTESIAN_POINT ( 'NONE',  ( 11.92109019680886206, 8.606374460406147620, -15.56934379943068336 ) ) ;
#22851=CARTESIAN_POINT ( 'NONE',  ( 36.04859390953723874, -22.18451583373416014, -15.00000000000000000 ) ) ;
#22854=CARTESIAN_POINT ( 'NONE',  ( 9.111692801717447665, 16.18521362881060455, -17.05508072787638696 ) ) ;
#22855=CARTESIAN_POINT ( 'NONE',  ( 33.26197456417788345, -12.91194637099222575, -20.70907993653955970 ) ) ;
#22857=CARTESIAN_POINT ( 'NONE',  ( 18.26618351132839280, 3.382507019981081164, -13.19753224271465797 ) ) ;
#22858=CARTESIAN_POINT ( 'NONE',  ( 18.30550780621970475, 8.505200139115956404, -19.80988581799093140 ) ) ;
#22860=CARTESIAN_POINT ( 'NONE',  ( 23.45579420008465732, -3.438291973250592992, -12.29892528769388349 ) ) ;
#22868=CARTESIAN_POINT ( 'NONE',  ( 33.90312036197754963, -11.11655558909185615, -17.69153855583423862 ) ) ;
#22871=CARTESIAN_POINT ( 'NONE',  ( 10.67335300198236148, 9.023663108408856104, -16.40923739229002010 ) ) ;
#22875=CARTESIAN_POINT ( 'NONE',  ( 26.87449084144840938, -11.88902188497427481, -13.49525739704605343 ) ) ;
#22878=CARTESIAN_POINT ( 'NONE',  ( 10.36430886937160167, 16.94616899698690204, -17.73806594831300032 ) ) ;
#22886=CARTESIAN_POINT ( 'NONE',  ( 12.50076791318051761, 8.571041463825640250, -15.12956297801270900 ) ) ;
#22892=CARTESIAN_POINT ( 'NONE',  ( 17.47275436513300662, 10.49281628697410262, -12.44556591811621082 ) ) ;
#22894=CARTESIAN_POINT ( 'NONE',  ( 17.31888479101057143, -0.09998177899580885930, -18.75936487049801116 ) ) ;
#22895=CARTESIAN_POINT ( 'NONE',  ( 24.88259999727891625, -1.109419405293186944, -15.69091174474707451 ) ) ;
#22896=CARTESIAN_POINT ( 'NONE',  ( 19.54218497767158169, 4.227554098413554229, -14.22708607227295730 ) ) ;
#22900=CARTESIAN_POINT ( 'NONE',  ( 17.18819971663578272, 0.8441372818425427749, -18.45219435416397502 ) ) ;
#22906=CARTESIAN_POINT ( 'NONE',  ( 10.35864918915110877, 16.97212501191939538, -17.91796598306941135 ) ) ;
#22913=CARTESIAN_POINT ( 'NONE',  ( 17.08157517049449581, 7.460725202527481947, -14.57009041681831896 ) ) ;
#22914=CARTESIAN_POINT ( 'NONE',  ( 11.40579136381300174, 16.08255417555669453, -16.73093107180499928 ) ) ;
#22915=CARTESIAN_POINT ( 'NONE',  ( 35.54859390953724585, -22.18451583373416014, -16.11276402859391865 ) ) ;
#22919=CARTESIAN_POINT ( 'NONE',  ( 13.15390973649967599, 8.859676595473322536, -14.60899741038990562 ) ) ;
#22921=CARTESIAN_POINT ( 'NONE',  ( 12.81042928357508970, 7.649856678006609734, -14.88275739421262855 ) ) ;
#22928=CARTESIAN_POINT ( 'NONE',  ( 13.41286507499157388, 9.756708335562493062, -15.68136934427840856 ) ) ;
#22929=CARTESIAN_POINT ( 'NONE',  ( 33.01527616964045109, -10.33189599206409959, -17.18388710919138873 ) ) ;
#22930=CARTESIAN_POINT ( 'NONE',  ( 26.47511176763426377, -7.718147522161595830, -18.64721581247919602 ) ) ;
#22936=CARTESIAN_POINT ( 'NONE',  ( 30.62762753239542590, -8.735908549479720620, -17.37160549233551876 ) ) ;
#22938=CARTESIAN_POINT ( 'NONE',  ( 23.31633574299079825, -8.368445843159939557, -15.61931793633953980 ) ) ;
#22947=CARTESIAN_POINT ( 'NONE',  ( 15.61762486822808604, 9.948436389806387226, -12.64537296286936829 ) ) ;
#22948=CARTESIAN_POINT ( 'NONE',  ( 28.67543231808702942, -10.82877479041544433, -19.00874469794426602 ) ) ;
#22952=CARTESIAN_POINT ( 'NONE',  ( 9.641350810849047548, 17.66889113945805789, -19.66666666666842644 ) ) ;
#22953=CARTESIAN_POINT ( 'NONE',  ( 16.71823672545656336, 7.456161109308904855, -19.47106720222115683 ) ) ;
#22956=CARTESIAN_POINT ( 'NONE',  ( 24.36497833745277930, -6.082191617938494055, -18.74521747929614435 ) ) ;
#22959=CARTESIAN_POINT ( 'NONE',  ( 11.05541531668977662, 17.68942339022145305, -17.94384837343789130 ) ) ;
#22961=CARTESIAN_POINT ( 'NONE',  ( 33.54145741815126058, -13.16751478770765793, -19.75123935038191192 ) ) ;
#22964=CARTESIAN_POINT ( 'NONE',  ( 24.81358459371387326, -5.676498915796258871, -18.90393244824272756 ) ) ;
#22966=CARTESIAN_POINT ( 'NONE',  ( 22.60637541839240683, -1.101515789306901194, -14.68923631892221948 ) ) ;
#22969=FILL_AREA_STYLE ('',( #8905 ) ) ;
#22970=CARTESIAN_POINT ( 'NONE',  ( 16.02150382621726976, 6.204807860950024789, -14.00014022580063155 ) ) ;
#22971=CARTESIAN_POINT ( 'NONE',  ( 25.78329585330208218, -10.67969159757694086, -14.14496057932236361 ) ) ;
#22983=CARTESIAN_POINT ( 'NONE',  ( 23.64629180402988951, 0.1506760071912668364, -12.95843554106259710 ) ) ;
#22984=CARTESIAN_POINT ( 'NONE',  ( 16.00562779705659011, 2.776126820729137190, -17.20623408552720690 ) ) ;
#22985=CARTESIAN_POINT ( 'NONE',  ( 33.01522398464379648, -9.800858501837518943, -19.11635465682842394 ) ) ;
#22988=CARTESIAN_POINT ( 'NONE',  ( 11.58682163191119230, 8.958038730125363003, -15.79767441425272345 ) ) ;
#22991=CARTESIAN_POINT ( 'NONE',  ( 9.664814466656260095, 16.24138283641780944, -17.88982567228806175 ) ) ;
#22996=CARTESIAN_POINT ( 'NONE',  ( 12.49742530276927610, 8.569573706352677789, -15.13222638044318735 ) ) ;
#23001=CARTESIAN_POINT ( 'NONE',  ( 16.01392728624657025, 9.853228751548474662, -15.03783782146776105 ) ) ;
#23004=CARTESIAN_POINT ( 'NONE',  ( 9.113844519079130180, 16.17534557870975576, -17.05418121134841414 ) ) ;
#23005=CARTESIAN_POINT ( 'NONE',  ( 34.17142927738225922, -16.99764464586957402, -20.98398627866201238 ) ) ;
#23006=CARTESIAN_POINT ( 'NONE',  ( 16.44673144568935541, 3.517958023484313301, -20.47440421422559353 ) ) ;
#23007=CARTESIAN_POINT ( 'NONE',  ( 14.77364001808635585, 4.929448384924057791, -16.82930887520970131 ) ) ;
#23009=CARTESIAN_POINT ( 'NONE',  ( 24.20684193479931068, 1.026663266619176840, -14.52337054612115708 ) ) ;
#23022=CARTESIAN_POINT ( 'NONE',  ( 33.98852084862024725, -11.13792163938717472, -17.92802646347312034 ) ) ;
#23023=CARTESIAN_POINT ( 'NONE',  ( 10.66743590522492369, 9.050377445005224786, -16.41171652237351353 ) ) ;
#23027=CARTESIAN_POINT ( 'NONE',  ( 26.38113052396219516, -11.59678093645141672, -17.84452879788985769 ) ) ;
#23029=CARTESIAN_POINT ( 'NONE',  ( 10.47212132250356120, 16.45172734403231729, -17.33476278219207956 ) ) ;
#23034=CARTESIAN_POINT ( 'NONE',  ( 12.53458732174692258, 8.585986940276173485, -15.10260830673100330 ) ) ;
#23038=CARTESIAN_POINT ( 'NONE',  ( 9.667771292961528928, 16.22782245407549340, -17.88511957776909966 ) ) ;
#23040=CARTESIAN_POINT ( 'NONE',  ( 21.24065112674864864, -1.570060580458334965, -19.57950003236798864 ) ) ;
#23041=CARTESIAN_POINT ( 'NONE',  ( 24.32739057165333207, -2.318628849198325348, -18.36682367714799824 ) ) ;
#23043=CARTESIAN_POINT ( 'NONE',  ( 21.44014932938603835, 4.813297736510089742, -15.98289606589226075 ) ) ;
#23046=CARTESIAN_POINT ( 'NONE',  ( 18.50902107916489570, 2.085137940960992697, -20.06823964296112450 ) ) ;
#23055=CARTESIAN_POINT ( 'NONE',  ( 10.35864918915110877, 16.97212501191939538, -17.98596209335946128 ) ) ;
#23056=CARTESIAN_POINT ( 'NONE',  ( 35.54859390953724585, -22.18451583373416014, -17.99055332684694974 ) ) ;
#23061=CARTESIAN_POINT ( 'NONE',  ( 15.41431293496917121, 3.575304669039410133, -17.09800041271234150 ) ) ;
#23062=CARTESIAN_POINT ( 'NONE',  ( 11.05541700792677062, 17.68941563399299710, -17.91138715956864047 ) ) ;
#23063=CARTESIAN_POINT ( 'NONE',  ( 35.54859390954303677, -22.18451583373416014, -15.55638201429745848 ) ) ;
#23066=CARTESIAN_POINT ( 'NONE',  ( 9.642214727206800617, 17.66492910891761525, -17.80644250212319690 ) ) ;
#23068=CARTESIAN_POINT ( 'NONE',  ( 12.76449053303042902, 7.629555522264023892, -14.91937138927071160 ) ) ;
#23071=ORIENTED_EDGE ( 'NONE', *, *, #9238, .T. ) ;
#23074=CARTESIAN_POINT ( 'NONE',  ( 10.46722255365007115, 16.47419372244215197, -17.33720764016775462 ) ) ;
#23075=CARTESIAN_POINT ( 'NONE',  ( 33.78657425947636739, -10.78854458652579495, -19.16640759269550287 ) ) ;
#23076=CARTESIAN_POINT ( 'NONE',  ( 25.73595588610537277, -4.826321120321507507, -18.84379041344559269 ) ) ;
#23082=CARTESIAN_POINT ( 'NONE',  ( 18.30550780621970475, 8.505200139115956404, -19.80988581799093140 ) ) ;
#23083=CARTESIAN_POINT ( 'NONE',  ( 24.94059380785660451, 0.5691772567322460619, -14.01379559947946518 ) ) ;
#23092=CARTESIAN_POINT ( 'NONE',  ( 10.72208662246453770, 16.62525560183325624, -15.95366392025685620 ) ) ;
#23097=CARTESIAN_POINT ( 'NONE',  ( 9.916118674515717046, 16.40877069192658055, -16.50468880802031890 ) ) ;
#23098=CARTESIAN_POINT ( 'NONE',  ( 16.64656040655037827, 6.484405094197702724, -15.29036880746224014 ) ) ;
#23101=CARTESIAN_POINT ( 'NONE',  ( 29.66490191837812773, -8.365349891895018430, -17.62461620872172574 ) ) ;
#23105=CARTESIAN_POINT ( 'NONE',  ( 12.27235684156208961, 9.528132359803098694, -15.31161062812042317 ) ) ;
#23107=CARTESIAN_POINT ( 'NONE',  ( 35.54859390954303677, -22.18451583373416014, -15.55638201429745848 ) ) ;
#23110=CARTESIAN_POINT ( 'NONE',  ( 23.28032035799162358, -0.8411909528121862545, -14.99295998388115869 ) ) ;
#23113=CARTESIAN_POINT ( 'NONE',  ( 19.75232399841803854, 1.290101960903724754, -14.36573431580270999 ) ) ;
#23114=CARTESIAN_POINT ( 'NONE',  ( 28.07139740185986199, -11.61962552671339388, -17.78409693965565452 ) ) ;
#23122=CARTESIAN_POINT ( 'NONE',  ( 9.870716668364401869, 16.61699007954640805, -16.53972800451630931 ) ) ;
#23123=CARTESIAN_POINT ( 'NONE',  ( 18.38621934312857320, -2.136830130942094730, -15.12482301043797683 ) ) ;
#23124=CARTESIAN_POINT ( 'NONE',  ( 16.12927480167980576, 2.990883400875756326, -18.25071113400840517 ) ) ;
#23125=CARTESIAN_POINT ( 'NONE',  ( 33.20847722810714231, -12.67161117835268058, -20.69290897523819694 ) ) ;
#23128=CARTESIAN_POINT ( 'NONE',  ( 12.37169234869624646, 8.529253869913038244, -15.23127513898213081 ) ) ;
#23132=CARTESIAN_POINT ( 'NONE',  ( 17.29421355564066332, 9.360779442694735053, -19.18964209290773937 ) ) ;
#23135=CARTESIAN_POINT ( 'NONE',  ( 12.52778158092594474, 8.582979361647906202, -15.10803260229456946 ) ) ;
#23141=CARTESIAN_POINT ( 'NONE',  ( 17.88091890332929523, 4.544920326333207861, -13.91018511019278669 ) ) ;
#23143=CARTESIAN_POINT ( 'NONE',  ( 9.193626274318058123, 15.80945627937554576, -17.02118864906812234 ) ) ;
#23144=CARTESIAN_POINT ( 'NONE',  ( 31.63980255171021483, -10.89810845426378982, -15.52824638758754183 ) ) ;
#23145=CARTESIAN_POINT ( 'NONE',  ( 15.23446545079332815, 2.143032791470029341, -16.75203451335420368 ) ) ;
#23146=CARTESIAN_POINT ( 'NONE',  ( 15.30293317557315902, 5.113330479851449617, -15.60941525921096051 ) ) ;
#23148=CARTESIAN_POINT ( 'NONE',  ( 22.59259966355045890, -3.831908474886262184, -12.47183693924707804 ) ) ;
#23157=CARTESIAN_POINT ( 'NONE',  ( 34.61014508914255572, -12.47609210860084161, -18.96169567217477692 ) ) ;
#23158=CARTESIAN_POINT ( 'NONE',  ( 12.70479305047265761, 7.604386330824797646, -14.96685888413283294 ) ) ;
#23162=CARTESIAN_POINT ( 'NONE',  ( 10.47187086816178159, 16.45287595956923354, -17.33486661187913214 ) ) ;
#23171=CARTESIAN_POINT ( 'NONE',  ( 12.56861602585598980, 8.601024833420110483, -15.07548682890769243 ) ) ;
#23175=CARTESIAN_POINT ( 'NONE',  ( 9.688134281814004822, 16.13443519152062677, -17.87669530545171881 ) ) ;
#23176=CARTESIAN_POINT ( 'NONE',  ( 24.39898194048076974, -1.181968365584514791, -14.84216225329429051 ) ) ;
#23177=CARTESIAN_POINT ( 'NONE',  ( 22.74932893098897324, -1.793276863599028381, -13.92998459126509836 ) ) ;
#23178=CARTESIAN_POINT ( 'NONE',  ( 18.25949499138229726, 0.6315596619015936275, -15.69045325149238934 ) ) ;
#23182=CARTESIAN_POINT ( 'NONE',  ( 28.15048769591263067, -5.842385520647848551, -16.89978903947823241 ) ) ;
#23191=CARTESIAN_POINT ( 'NONE',  ( 10.35870477237433818, 16.97187010017241349, -17.89775757279876700 ) ) ;
#23195=CARTESIAN_POINT ( 'NONE',  ( 11.22298328736398965, 9.095422004326360721, -17.24198125015536576 ) ) ;
#23198=CARTESIAN_POINT ( 'NONE',  ( 19.83745040964868522, -2.306422872736943575, -14.39351019504378293 ) ) ;
#23199=CARTESIAN_POINT ( 'NONE',  ( 11.27618196228310232, 16.67695941232857137, -16.78452903358395076 ) ) ;
#23200=CARTESIAN_POINT ( 'NONE',  ( 35.54859569580823830, -22.18452385850428499, -18.27063337037174762 ) ) ;
#23203=CARTESIAN_POINT ( 'NONE',  ( 9.916824447075894611, 16.40553392900050156, -16.50439446175997205 ) ) ;
#23206=CARTESIAN_POINT ( 'NONE',  ( 9.641350810849047548, 17.66889113945805789, -17.93331994345748370 ) ) ;
#23214=CARTESIAN_POINT ( 'NONE',  ( 10.47175433613752027, 16.45341039028688002, -17.33491556667247835 ) ) ;
#23216=CARTESIAN_POINT ( 'NONE',  ( 34.14034160798153295, -12.36551392957089135, -20.90432844665832590 ) ) ;
#23217=CARTESIAN_POINT ( 'NONE',  ( 26.61709978538234012, -3.831456866606135492, -17.85214630790261836 ) ) ;
#23223=CARTESIAN_POINT ( 'NONE',  ( 18.83884422780463552, 9.149888288241003309, -18.99120665306858768 ) ) ;
#23224=CARTESIAN_POINT ( 'NONE',  ( 30.43753979984721525, -10.17066761781405937, -14.50402091508011537 ) ) ;
#23235=CARTESIAN_POINT ( 'NONE',  ( 10.68867725192709273, 16.77847523382220984, -15.97313786900300059 ) ) ;
#23240=CARTESIAN_POINT ( 'NONE',  ( 9.916775705961365261, 16.40575746196480011, -16.50441451066904364 ) ) ;
#23244=CARTESIAN_POINT ( 'NONE',  ( 17.80416238081608071, 8.561068417093343541, -18.87148919878627140 ) ) ;
#23248=CARTESIAN_POINT ( 'NONE',  ( 28.09718568327657806, -5.958257988085632562, -17.17874431236187149 ) ) ;
#23253=CARTESIAN_POINT ( 'NONE',  ( 11.35716248442908061, 16.30557241515140277, -16.75104082405111683 ) ) ;
#23255=CARTESIAN_POINT ( 'NONE',  ( 35.54859390953723874, -22.18451583373416014, -15.00000000000000000 ) ) ;
#23259=CARTESIAN_POINT ( 'NONE',  ( 27.22116495027615812, -8.412805768781604243, -11.93592671293571605 ) ) ;
#23263=CARTESIAN_POINT ( 'NONE',  ( 16.37314578033188894, 3.237113944496374351, -18.86778596048347723 ) ) ;
#23265=CARTESIAN_POINT ( 'NONE',  ( 30.29779709953443501, -9.168887887504279632, -16.05354238668875055 ) ) ;
#23272=CARTESIAN_POINT ( 'NONE',  ( 9.643509238790151983, 17.65899231378470446, -17.74106871770035099 ) ) ;
#23273=CARTESIAN_POINT ( 'NONE',  ( 22.70908579165946506, -0.2254420654732764706, -12.61778515557981528 ) ) ;
#23274=CARTESIAN_POINT ( 'NONE',  ( 23.41849298471255381, -3.203224238779429633, -13.27670244232306018 ) ) ;
#23275=CARTESIAN_POINT ( 'NONE',  ( 32.00851579392290347, -10.30430276118739918, -18.57203464379605151 ) ) ;
#23279=CARTESIAN_POINT ( 'NONE',  ( 12.77278825050581013, 8.691252192278360766, -14.91275796197543890 ) ) ;
#23283=CARTESIAN_POINT ( 'NONE',  ( 17.17204249742301059, 10.23148044644768362, -15.96021614775051667 ) ) ;
#23287=CARTESIAN_POINT ( 'NONE',  ( 10.72892505862787971, 16.59389366189031634, -15.95083598634710320 ) ) ;
#23291=CARTESIAN_POINT ( 'NONE',  ( 20.23291344124205793, 5.521974472852556381, -14.51730806008046137 ) ) ;
#23294=CARTESIAN_POINT ( 'NONE',  ( 33.10306327339915811, -12.22190834454405106, -20.64716665866461298 ) ) ;
#23295=CARTESIAN_POINT ( 'NONE',  ( 21.76348650023563636, -1.483442554740824537, -14.70963264896640155 ) ) ;
#23296=CARTESIAN_POINT ( 'NONE',  ( 31.88113401528661939, -11.03952345999570639, -14.96145667752709585 ) ) ;
#23298=CARTESIAN_POINT ( 'NONE',  ( 23.10480167063333212, 0.6704577443818302562, -13.62402792225823944 ) ) ;
#23308=CARTESIAN_POINT ( 'NONE',  ( 36.54859390953724585, -21.18451583373416014, -17.64281456791166391 ) ) ;
#23309=CARTESIAN_POINT ( 'NONE',  ( 9.641350777746193756, 17.66889129127197577, -17.91630266473768884 ) ) ;
#23314=CARTESIAN_POINT ( 'NONE',  ( 10.47008273352651564, 16.46107657294071203, -17.33567129194344858 ) ) ;
#23324=CARTESIAN_POINT ( 'NONE',  ( 9.672937757006597081, 16.20412839139380168, -17.88297960302892520 ) ) ;
#23326=CARTESIAN_POINT ( 'NONE',  ( 25.61676826379006400, -5.274948970184475172, -14.00514367894158418 ) ) ;
#23327=CARTESIAN_POINT ( 'NONE',  ( 21.31799488982693802, -2.441251725956471219, -14.24326171688714204 ) ) ;
#23328=CARTESIAN_POINT ( 'NONE',  ( 18.32179412900206827, 3.681508181950223335, -14.15692665485406643 ) ) ;
#23332=CARTESIAN_POINT ( 'NONE',  ( 24.43075134246613800, -6.859861339260811874, -14.00379227226492951 ) ) ;
#23343=CARTESIAN_POINT ( 'NONE',  ( 10.35867142355733783, 16.97202304209818990, -17.90451223021000260 ) ) ;
#23346=CARTESIAN_POINT ( 'NONE',  ( 32.52799721746220740, -11.03300674309804386, -18.03857687357939099 ) ) ;
#23348=CARTESIAN_POINT ( 'NONE',  ( 11.25771276049011327, 8.953580691464267716, -17.22628983894280807 ) ) ;
#23351=CARTESIAN_POINT ( 'NONE',  ( 19.68115760211910725, 3.144890361740488860, -20.29587546762095940 ) ) ;
#23352=CARTESIAN_POINT ( 'NONE',  ( 11.05818223728759264, 17.67673393965927175, -17.74095938596937572 ) ) ;
#23356=CARTESIAN_POINT ( 'NONE',  ( 9.641351338355821810, 17.66888872024471624, -17.91303689663363130 ) ) ;
#23358=CARTESIAN_POINT ( 'NONE',  ( 10.04637620539468124, 15.81139305134258599, -16.45082025127570091 ) ) ;
#23364=CARTESIAN_POINT ( 'NONE',  ( 10.47187086816178159, 16.45287595956923354, -17.33486661187913214 ) ) ;
#23367=CARTESIAN_POINT ( 'NONE',  ( 35.97124720801268438, -19.59080293283771823, -20.41544573823858144 ) ) ;
#23368=CARTESIAN_POINT ( 'NONE',  ( 26.07968421886551980, -9.001936657367064498, -13.61655714643126913 ) ) ;
#23371=CARTESIAN_POINT ( 'NONE',  ( 33.33685173283005554, -10.38074443705513161, -18.09276096107157628 ) ) ;
#23373=CARTESIAN_POINT ( 'NONE',  ( 27.39958189869922123, -12.72506959635235368, -13.65552181841346524 ) ) ;
#23374=CARTESIAN_POINT ( 'NONE',  ( 25.72483820513325270, -9.972596264566449875, -15.12420980763781664 ) ) ;
#23389=CARTESIAN_POINT ( 'NONE',  ( 10.33811767156285555, 18.38618615532545064, -17.91197029530843565 ) ) ;
#23394=CARTESIAN_POINT ( 'NONE',  ( 11.21346931060482000, 10.45895530107994098, -15.96818619734747458 ) ) ;
#23396=CARTESIAN_POINT ( 'NONE',  ( 16.52347908691095668, 7.282719431485021211, -19.45954596032283845 ) ) ;
#23399=CARTESIAN_POINT ( 'NONE',  ( 24.87127057246125972, -9.548149280147088191, -14.79180087847266556 ) ) ;
#23402=CARTESIAN_POINT ( 'NONE',  ( 11.26682494837019277, 16.71987187087499294, -16.78921452078379062 ) ) ;
#23404=CARTESIAN_POINT ( 'NONE',  ( 33.98143228033899987, -14.14408878234146982, -18.84191164812894570 ) ) ;
#23405=CARTESIAN_POINT ( 'NONE',  ( 17.78594395145776019, 10.14170102421038422, -17.68001733040774681 ) ) ;
#23407=CARTESIAN_POINT ( 'NONE',  ( 26.37963984661160310, -4.639223599391875119, -13.30093322687953616 ) ) ;
#23408=ORIENTED_EDGE ( 'NONE', *, *, #6052, .T. ) ;
#23412=CARTESIAN_POINT ( 'NONE',  ( 17.70500667399921824, 3.403337836861581867, -14.36321643528369663 ) ) ;
#23413=CARTESIAN_POINT ( 'NONE',  ( 18.80816768961129881, 6.772028514247487863, -18.23967922641782380 ) ) ;
#23428=CARTESIAN_POINT ( 'NONE',  ( 9.916637298967875935, 16.40639221407973380, -16.50447193873893781 ) ) ;
#23429=CARTESIAN_POINT ( 'NONE',  ( 27.79171034377997884, -3.119812929724471662, -15.83729198868751276 ) ) ;
#23430=CARTESIAN_POINT ( 'NONE',  ( 19.95076809599375878, -1.008983920988137495, -18.52968236344498720 ) ) ;
#23431=CARTESIAN_POINT ( 'NONE',  ( 32.19500574710832552, -10.39459394146955518, -19.06308269698291014 ) ) ;
#23435=CARTESIAN_POINT ( 'NONE',  ( 12.60945047077962933, 8.619070305187777947, -15.04294105552940231 ) ) ;
#23438=CARTESIAN_POINT ( 'NONE',  ( 14.73401617531889229, 6.408058468588501810, -15.60580005407095960 ) ) ;
#23441=CARTESIAN_POINT ( 'NONE',  ( 10.33811693838771717, 18.38618951776012267, -17.91928203681695564 ) ) ;
#23445=CARTESIAN_POINT ( 'NONE',  ( 21.41025690189560748, 5.821651141963339882, -16.00656683556521998 ) ) ;
#23447=CARTESIAN_POINT ( 'NONE',  ( 27.89044320811645505, -9.967159925860730851, -19.81290489186636350 ) ) ;
#23449=CARTESIAN_POINT ( 'NONE',  ( 34.74206752880779447, -19.56122003402509080, -21.15647653254228189 ) ) ;
#23451=CARTESIAN_POINT ( 'NONE',  ( 21.82779397375749753, -0.5565768812632180262, -18.88406021698092729 ) ) ;
#23454=CARTESIAN_POINT ( 'NONE',  ( 19.48014203372339992, 3.175912578606837844, -18.88683143354647243 ) ) ;
#23455=CARTESIAN_POINT ( 'NONE',  ( 25.37029659992048281, -10.87484012800900501, -14.78472363349550811 ) ) ;
#23464=CARTESIAN_POINT ( 'NONE',  ( 36.49521523454778560, -20.94471372247522467, -19.05937150832556526 ) ) ;
#23466=CARTESIAN_POINT ( 'NONE',  ( 12.77299770905688803, 7.633314995549595139, -14.91259101981587420 ) ) ;
#23470=CARTESIAN_POINT ( 'NONE',  ( 10.47604570704546845, 16.43372961628045559, -17.33313991065496751 ) ) ;
#23480=CARTESIAN_POINT ( 'NONE',  ( 9.992064777962580635, 14.74057119405591543, -17.75100935390776158 ) ) ;
#23483=CARTESIAN_POINT ( 'NONE',  ( 25.59007283008577005, -3.201708215360036913, -15.56755918271449168 ) ) ;
#23484=CARTESIAN_POINT ( 'NONE',  ( 16.03657434348277633, 2.746931742562784162, -16.83325620853174698 ) ) ;
#23488=CARTESIAN_POINT ( 'NONE',  ( 26.58455406938135468, -5.910422570377376950, -13.89432871846328688 ) ) ;
#23494=CARTESIAN_POINT ( 'NONE',  ( 10.47705880869930084, 16.42908340295556258, -17.33272095748315422 ) ) ;
#23495=CARTESIAN_POINT ( 'NONE',  ( 35.54859390953724585, -22.18451583373416014, -16.94733705004010460 ) ) ;
#23496=CARTESIAN_POINT ( 'NONE',  ( 33.68411698100747032, -13.80840863474736935, -19.79436191385186916 ) ) ;
#23498=CARTESIAN_POINT ( 'NONE',  ( 13.37894900189793290, 7.625660844661456217, -15.70840104182326513 ) ) ;
#23502=CARTESIAN_POINT ( 'NONE',  ( 16.89609864265585060, 4.102175112930991574, -14.31125941877678720 ) ) ;
#23503=CARTESIAN_POINT ( 'NONE',  ( 11.27636807789780171, 16.67610586239533177, -16.78445215232725118 ) ) ;
#23507=CARTESIAN_POINT ( 'NONE',  ( 9.675370519060759733, 17.51287242109451014, -17.23928541814325399 ) ) ;
#23509=CARTESIAN_POINT ( 'NONE',  ( 9.675370519060759733, 17.51287242109451014, -17.23928541814325399 ) ) ;
#23515=CARTESIAN_POINT ( 'NONE',  ( 10.35865474790814211, 16.97209951875106526, -17.91014213605047445 ) ) ;
#23518=CARTESIAN_POINT ( 'NONE',  ( 36.13838427452936486, -20.34166123773320578, -20.43658233646779365 ) ) ;
#23519=CARTESIAN_POINT ( 'NONE',  ( 31.59793210864275537, -10.01186915388335485, -14.42687813506083039 ) ) ;
#23520=CARTESIAN_POINT ( 'NONE',  ( 26.18758235895636233, -4.355437658720127558, -18.53605802859044260 ) ) ;
#23526=CARTESIAN_POINT ( 'NONE',  ( 33.78657425947636739, -10.78854458652579495, -19.16640759269550287 ) ) ;
#23528=CARTESIAN_POINT ( 'NONE',  ( 16.80936620776159884, 5.784822248606665163, -14.58992565756060245 ) ) ;
#23529=CARTESIAN_POINT ( 'NONE',  ( 15.19603151210977821, 9.502094893032342782, -14.87270315361914896 ) ) ;
#23540=CARTESIAN_POINT ( 'NONE',  ( 10.33886748782435561, 18.38274740237080351, -17.79416814676874381 ) ) ;
#23544=CARTESIAN_POINT ( 'NONE',  ( 11.47257016429183452, 9.270685755423764718, -15.86103888016343255 ) ) ;
#23546=CARTESIAN_POINT ( 'NONE',  ( 9.662623034719734605, 16.25143302262299372, -17.90105808085208849 ) ) ;
#23548=CARTESIAN_POINT ( 'NONE',  ( 17.00905032053054811, 4.985101812230166907, -18.82491780458422781 ) ) ;
#23551=CARTESIAN_POINT ( 'NONE',  ( 24.68825858685077179, -9.385095155728059524, -16.92495907518576104 ) ) ;
#23554=CARTESIAN_POINT ( 'NONE',  ( 11.05558847800967648, 17.68862925033535660, -17.87192865789842955 ) ) ;
#23557=CARTESIAN_POINT ( 'NONE',  ( 35.54859306210901337, -21.18451202668684985, -18.38798429269037271 ) ) ;
#23563=CARTESIAN_POINT ( 'NONE',  ( 30.62308825650849187, -7.210737555064373083, -14.15269394828060889 ) ) ;
#23566=CARTESIAN_POINT ( 'NONE',  ( 19.30972751531945519, 5.994221256738944348, -19.84686166629000326 ) ) ;
#23567=CARTESIAN_POINT ( 'NONE',  ( 14.65865118920550714, 8.193166376910747672, -14.78953851775792216 ) ) ;
#23577=CARTESIAN_POINT ( 'NONE',  ( 9.641350810849047548, 17.66889113945805789, -17.91796598306941135 ) ) ;
#23578=CARTESIAN_POINT ( 'NONE',  ( 18.80130396411469462, -1.975481315223051704, -14.30362724594584378 ) ) ;
#23579=CARTESIAN_POINT ( 'NONE',  ( 19.39950943988042553, -1.649204456521256246, -16.58530004841527727 ) ) ;
#23580=CARTESIAN_POINT ( 'NONE',  ( 36.52535953212831998, -23.08013608362457703, -19.17046861472280028 ) ) ;
#23586=CARTESIAN_POINT ( 'NONE',  ( 17.12833724908345800, 9.171387755021909172, -19.38714867094073213 ) ) ;
#23589=CARTESIAN_POINT ( 'NONE',  ( 10.33812866905494587, 18.38613571942487113, -17.90056368370468931 ) ) ;
#23594=CARTESIAN_POINT ( 'NONE',  ( 19.11618317516819587, 7.271703427217982352, -19.10559232466456692 ) ) ;
#23598=CARTESIAN_POINT ( 'NONE',  ( 32.75486304968715245, -9.956179044816899193, -14.71053347703266212 ) ) ;
#23601=CARTESIAN_POINT ( 'NONE',  ( 35.54859569580823830, -22.18452385850428499, -18.27063337037174762 ) ) ;
#23602=CARTESIAN_POINT ( 'NONE',  ( 23.33733100364600688, 1.020658515592549609, -17.81090727445316446 ) ) ;
#23603=CARTESIAN_POINT ( 'NONE',  ( 16.84916689134472989, 3.454690908320265041, -17.64892000621457413 ) ) ;
#23605=CARTESIAN_POINT ( 'NONE',  ( 28.24905293252005123, -11.45655955306129314, -17.88756844200554141 ) ) ;
#23614=CARTESIAN_POINT ( 'NONE',  ( 36.54517214193456454, -21.16914364445853280, -18.53042016804813841 ) ) ;
#23615=CARTESIAN_POINT ( 'NONE',  ( 12.75629879507850717, 7.625935294889710114, -14.92590036059129943 ) ) ;
#23619=CARTESIAN_POINT ( 'NONE',  ( 11.94706930840425407, 9.687427868553587729, -16.72481990518296158 ) ) ;
#23633=CARTESIAN_POINT ( 'NONE',  ( 9.668505437271095460, 16.22445557469016464, -17.88481252315560965 ) ) ;
#23634=CARTESIAN_POINT ( 'NONE',  ( 24.61983070264756890, -3.485318192270607351, -14.59657465048590907 ) ) ;
#23636=CARTESIAN_POINT ( 'NONE',  ( 20.75491211191951635, -1.144232541536293946, -14.27023797479654554 ) ) ;
#23641=CARTESIAN_POINT ( 'NONE',  ( 26.61709978538234012, -3.831456866606135492, -17.85214630790261836 ) ) ;
#23648=CARTESIAN_POINT ( 'NONE',  ( 11.98759337455738816, 9.501579335558542283, -16.70806177831036976 ) ) ;
#23650=CARTESIAN_POINT ( 'NONE',  ( 34.75406370242679799, -18.61511248754081294, -20.11778113987843852 ) ) ;
#23652=CARTESIAN_POINT ( 'NONE',  ( 8.944605280299260386, 16.95149830073946617, -17.90242062344065843 ) ) ;
#23656=CARTESIAN_POINT ( 'NONE',  ( 23.66601916330066402, 2.199037240492611733, -18.57254039386976885 ) ) ;
#23657=CARTESIAN_POINT ( 'NONE',  ( 12.83257874964047929, 9.539242390270068483, -16.14089537112711525 ) ) ;
#23661=CARTESIAN_POINT ( 'NONE',  ( 9.870716668364401869, 16.61699007954640805, -16.53972800451630931 ) ) ;
#23663=CARTESIAN_POINT ( 'NONE',  ( 9.997747326010761881, 16.03441129093729245, -16.47093000352221637 ) ) ;
#23669=CARTESIAN_POINT ( 'NONE',  ( 10.60167031212029443, 15.85759916399494607, -17.28118971735050735 ) ) ;
#23672=CARTESIAN_POINT ( 'NONE',  ( 36.18478257229246964, -20.55010421171508028, -20.40673782175607442 ) ) ;
#23673=CARTESIAN_POINT ( 'NONE',  ( 29.46565128511723586, -7.689737916804423534, -14.82739468409561567 ) ) ;
#23674=CARTESIAN_POINT ( 'NONE',  ( 14.45328171724474231, 7.053988074037379263, -14.59236433646538522 ) ) ;
#23677=CARTESIAN_POINT ( 'NONE',  ( 34.91913293194685508, -14.86421081092256280, -20.09741683264573808 ) ) ;
#23679=CARTESIAN_POINT ( 'NONE',  ( 17.54325408622900184, 7.715740848240963068, -20.30207397218512000 ) ) ;
#23681=CARTESIAN_POINT ( 'NONE',  ( 27.63516133065608926, -10.68623331565014034, -17.71408682504818088 ) ) ;
#23692=CARTESIAN_POINT ( 'NONE',  ( 10.33830461362823883, 18.38532881518400686, -17.85494544563047370 ) ) ;
#23697=CARTESIAN_POINT ( 'NONE',  ( 9.918725397012197575, 16.39681593027784956, -16.50360835092378409 ) ) ;
#23699=CARTESIAN_POINT ( 'NONE',  ( 9.667845848563926481, 16.22748053257927126, -17.88508528815513543 ) ) ;
#23701=CARTESIAN_POINT ( 'NONE',  ( 23.16309603597909472, 3.730466837354933674, -16.34659541137592598 ) ) ;
#23704=CARTESIAN_POINT ( 'NONE',  ( 24.78692427941192733, -9.284778175067517125, -17.23615439686343720 ) ) ;
#23708=CARTESIAN_POINT ( 'NONE',  ( 11.05584814685795081, 17.68743837589741830, -17.84564518929906285 ) ) ;
#23709=VERTEX_POINT ( 'NONE', #15309 ) ;
#23710=CARTESIAN_POINT ( 'NONE',  ( 34.33808118748100924, -15.74632339993765484, -18.94971805680347998 ) ) ;
#23711=CARTESIAN_POINT ( 'NONE',  ( 16.09764958744793262, 8.143416238145906760, -19.84970969296679044 ) ) ;
#23713=CARTESIAN_POINT ( 'NONE',  ( 9.026809008904539411, 16.57450152281700184, -17.18797639273109112 ) ) ;
#23714=CARTESIAN_POINT ( 'NONE',  ( 31.07149168920019733, -7.992644923617350905, -17.88177209202816087 ) ) ;
#23718=CARTESIAN_POINT ( 'NONE',  ( 17.40782953567980229, 3.270613820851801190, -14.52895612053623609 ) ) ;
#23719=CARTESIAN_POINT ( 'NONE',  ( 15.96855819401819865, 6.783166013289068985, -19.29613786212107840 ) ) ;
#23736=CARTESIAN_POINT ( 'NONE',  ( 9.916775705961365261, 16.40575746196480011, -16.50441451066904364 ) ) ;
#23737=CARTESIAN_POINT ( 'NONE',  ( 25.65469514739125856, -9.762610920096198797, -17.09127189072687614 ) ) ;
#23738=CARTESIAN_POINT ( 'NONE',  ( 20.49605984403359216, -1.259233478192978373, -14.44550164344372511 ) ) ;
#23739=CARTESIAN_POINT ( 'NONE',  ( 33.52946124453396237, -14.11362233419136381, -20.78993474304632372 ) ) ;
#23746=CARTESIAN_POINT ( 'NONE',  ( 16.77165338796101324, 10.12286561294300569, -15.51291369241808304 ) ) ;
#23749=CARTESIAN_POINT ( 'NONE',  ( 10.33811723165831786, 18.38618817278374706, -17.91339614244408907 ) ) ;
#23753=CARTESIAN_POINT ( 'NONE',  ( 17.63704213852533442, 9.806822523219006271, -18.50018230520716145 ) ) ;
#23754=CARTESIAN_POINT ( 'NONE',  ( 30.27995308908331751, -6.828448725465094959, -15.78586218199752622 ) ) ;
#23756=CARTESIAN_POINT ( 'NONE',  ( 34.54007435814109783, -17.65377171698271752, -20.05309729467257540 ) ) ;
#23757=CARTESIAN_POINT ( 'NONE',  ( 20.82085833995528290, -1.902372073343062908, -15.34044165217533617 ) ) ;
#23758=CARTESIAN_POINT ( 'NONE',  ( 20.30290135898079384, 0.5855005908018823257, -19.57000235946889433 ) ) ;
#23760=CARTESIAN_POINT ( 'NONE',  ( 29.03550452591436937, -6.934775515252377787, -18.27713033076000215 ) ) ;
#23774=CARTESIAN_POINT ( 'NONE',  ( 36.00107582698698394, -18.72480711723410352, -19.38214066600889751 ) ) ;
#23776=CARTESIAN_POINT ( 'NONE',  ( 9.644802874473198173, 17.65305953564175567, -17.69767226479352118 ) ) ;
#23780=CARTESIAN_POINT ( 'NONE',  ( 12.02871927673971619, 9.312984558958580905, -16.69105371450780595 ) ) ;
#23790=CARTESIAN_POINT ( 'NONE',  ( 13.37597118643279970, 7.624349635725309327, -15.71077405172158947 ) ) ;
#23792=CARTESIAN_POINT ( 'NONE',  ( 22.79055345825320344, -4.301464833599455417, -14.90020420563294046 ) ) ;
#23793=CARTESIAN_POINT ( 'NONE',  ( 19.79269262995316936, -1.159804626089355084, -18.29502107036499581 ) ) ;
#23809=CARTESIAN_POINT ( 'NONE',  ( 10.47139596700049147, 16.45505391683073526, -17.33506929010674114 ) ) ;
#23811=CARTESIAN_POINT ( 'NONE',  ( 32.36240160181304759, -11.00785621467150044, -17.57054915585148436 ) ) ;
#23814=CARTESIAN_POINT ( 'NONE',  ( 8.944617638130560877, 16.95144162614991501, -17.89908301402565982 ) ) ;
#23815=CARTESIAN_POINT ( 'NONE',  ( 18.04049687913209610, 0.8262538513465327306, -14.27019888128743297 ) ) ;
#23816=CARTESIAN_POINT ( 'NONE',  ( 12.83625023806442655, 9.529724225483313660, -16.13881881377442795 ) ) ;
#23820=CARTESIAN_POINT ( 'NONE',  ( 10.04637620539468124, 15.81139305134258599, -16.45082025127570091 ) ) ;
#23822=CARTESIAN_POINT ( 'NONE',  ( 11.40798482813988635, 9.566882342703072695, -15.88774718835883348 ) ) ;
#23825=ORIENTED_EDGE ( 'NONE', *, *, #10730, .T. ) ;
#23828=CARTESIAN_POINT ( 'NONE',  ( 12.01190781424926435, 9.390070215761314287, -16.69800690218674788 ) ) ;
#23830=CARTESIAN_POINT ( 'NONE',  ( 36.54859390953724585, -22.18451583373416014, -18.06010107863414405 ) ) ;
#23831=CARTESIAN_POINT ( 'NONE',  ( 25.97851742199650005, -11.98992670343847244, -16.97112261376066655 ) ) ;
#23832=CARTESIAN_POINT ( 'NONE',  ( 29.72799312938100513, -7.689056491358781997, -15.42978383025728384 ) ) ;
#23835=CARTESIAN_POINT ( 'NONE',  ( 33.01527616964045109, -10.33189599206409959, -17.18388710919138873 ) ) ;
#23838=CARTESIAN_POINT ( 'NONE',  ( 19.97593658988278165, 3.663230212540239616, -18.70116431613266883 ) ) ;
#23840=CARTESIAN_POINT ( 'NONE',  ( 28.54819463643023880, -8.737303380947411213, -14.37855314081258307 ) ) ;
#23853=CARTESIAN_POINT ( 'NONE',  ( 12.24912255266251293, 9.517392596235749735, -15.33016477413064393 ) ) ;
#23859=CARTESIAN_POINT ( 'NONE',  ( 11.47338783222600789, 9.266948822715743717, -15.86069975447064806 ) ) ;
#23861=CARTESIAN_POINT ( 'NONE',  ( 19.75347561433959953, 2.650395817966514578, -13.58229691592852184 ) ) ;
#23867=CARTESIAN_POINT ( 'NONE',  ( 11.05544237569323762, 17.68929929418238700, -17.89823164173536441 ) ) ;
#23869=CARTESIAN_POINT ( 'NONE',  ( 35.54859390953724585, -21.18451583373416014, -17.99055332684694974 ) ) ;
#23870=CARTESIAN_POINT ( 'NONE',  ( 17.95327243003904982, 7.812726124483462264, -14.88485059575767266 ) ) ;
#23873=CARTESIAN_POINT ( 'NONE',  ( 9.111161770198492604, 16.18764900704733378, -17.05531488649033633 ) ) ;
#23874=CARTESIAN_POINT ( 'NONE',  ( 30.37590262355644910, -7.260401249342992358, -13.74898149931492775 ) ) ;
#23880=CARTESIAN_POINT ( 'NONE',  ( 21.19231167106929803, 0.1271100694386541607, -19.24388053421374778 ) ) ;
#23881=CARTESIAN_POINT ( 'NONE',  ( 15.19333023161420648, 6.044621996704095501, -18.15278115226310263 ) ) ;
#23895=CARTESIAN_POINT ( 'NONE',  ( 11.47395765415086188, 9.264374527449886543, -15.86046114005151075 ) ) ;
#23896=CARTESIAN_POINT ( 'NONE',  ( 27.04128250769109698, -11.23896722199365961, -17.17396923023889244 ) ) ;
#23897=CARTESIAN_POINT ( 'NONE',  ( 22.96196402503608169, -2.069733343145511828, -19.51364111617685992 ) ) ;
#23898=CARTESIAN_POINT ( 'NONE',  ( 35.46335518829674527, -22.80158341140986167, -19.83799967047498924 ) ) ;
#23902=CARTESIAN_POINT ( 'NONE',  ( 12.50226005284522657, 8.571700941790735939, -15.12837371066060221 ) ) ;
#23905=CARTESIAN_POINT ( 'NONE',  ( 23.66272512268759343, 2.894330346666426745, -16.12005855839824520 ) ) ;
#23909=CARTESIAN_POINT ( 'NONE',  ( 10.65690970294255280, 16.92416526288626955, -16.00322527524160066 ) ) ;
#23913=CARTESIAN_POINT ( 'NONE',  ( 23.61827771231835982, -0.6465389018800060672, -13.57143891608981612 ) ) ;
#23915=CARTESIAN_POINT ( 'NONE',  ( 17.99586569009407455, 10.99629947005995767, -19.18704736271931210 ) ) ;
#23917=CARTESIAN_POINT ( 'NONE',  ( 33.44337896868773186, -12.72690026786775341, -19.72159258799634074 ) ) ;
#23919=CARTESIAN_POINT ( 'NONE',  ( 21.64008331710702038, -0.7226702609205537531, -18.85644019536628946 ) ) ;
#23921=CARTESIAN_POINT ( 'NONE',  ( 16.81761937449845234, 3.371063479271922514, -17.17107737352595720 ) ) ;
#23923=CARTESIAN_POINT ( 'NONE',  ( 26.92475197568164802, -10.17130474311345800, -13.43658410890694732 ) ) ;
#23933=CARTESIAN_POINT ( 'NONE',  ( 36.09161981528372110, -20.13157329416283048, -20.44814669990763889 ) ) ;
#23934=CARTESIAN_POINT ( 'NONE',  ( 12.89209817343266984, 7.685947621549766851, -14.81766584744191739 ) ) ;
#23938=CARTESIAN_POINT ( 'NONE',  ( 12.22285885739602662, 8.868278133530205665, -16.57678160000113721 ) ) ;
#23950=CARTESIAN_POINT ( 'NONE',  ( 11.22589550380084411, 9.082134330754477958, -17.24077175062176082 ) ) ;
#23953=CARTESIAN_POINT ( 'NONE',  ( 24.97936687747968776, -7.804033356035183999, -18.74018705570338028 ) ) ;
#23955=CARTESIAN_POINT ( 'NONE',  ( 22.68884594494833706, -6.762261587817247843, -18.56982216542981234 ) ) ;
#23967=CARTESIAN_POINT ( 'NONE',  ( 12.02835731808789355, 9.314632867394664117, -16.69120428796748357 ) ) ;
#23969=CARTESIAN_POINT ( 'NONE',  ( 32.96569147872224903, -11.36116021242123608, -19.12347989294568151 ) ) ;
#23971=CARTESIAN_POINT ( 'NONE',  ( 13.37268442792299261, 7.622911828202562745, -15.71339253741762221 ) ) ;
#23973=CARTESIAN_POINT ( 'NONE',  ( 24.14317479683219858, -6.286850201977149055, -18.60698471650063723 ) ) ;
#23974=CARTESIAN_POINT ( 'NONE',  ( 12.82717298413408358, 9.563916880749394167, -16.14313977175105919 ) ) ;
#23978=CARTESIAN_POINT ( 'NONE',  ( 11.47652547240386944, 9.253065934422213701, -15.85936358228339316 ) ) ;
#23980=CARTESIAN_POINT ( 'NONE',  ( 9.917712295358372288, 16.40146214360271770, -16.50402730409559027 ) ) ;
#23985=CARTESIAN_POINT ( 'NONE',  ( 12.02823749386838514, 9.315180647891255106, -16.69125397286443047 ) ) ;
#23987=CARTESIAN_POINT ( 'NONE',  ( 36.45689639539443050, -22.77256747621617095, -19.95163700058902734 ) ) ;
#23988=CARTESIAN_POINT ( 'NONE',  ( 15.23264752967198099, 8.612683518626374379, -20.21708921969009154 ) ) ;
#23989=CARTESIAN_POINT ( 'NONE',  ( 16.60417661732421735, 9.954854064686266213, -19.72231676211552909 ) ) ;
#23998=CARTESIAN_POINT ( 'NONE',  ( 16.84916689134472989, 3.454690908320265041, -17.64892000621457413 ) ) ;
#23999=CARTESIAN_POINT ( 'NONE',  ( 18.88762249820254624, 5.002188274287570735, -13.90571046850145542 ) ) ;
#24007=CARTESIAN_POINT ( 'NONE',  ( 12.27491818236995691, 9.503772128122387031, -15.31151344616081822 ) ) ;
#24011=CARTESIAN_POINT ( 'NONE',  ( 12.07641845611955489, 8.540206757827041528, -15.45582622123028216 ) ) ;
#24014=CARTESIAN_POINT ( 'NONE',  ( 20.52698940127687877, 5.222567878441341627, -18.38034891569893503 ) ) ;
#24018=CARTESIAN_POINT ( 'NONE',  ( 12.82970573826865390, 9.552301347437191836, -16.14209238882153130 ) ) ;
#24020=CARTESIAN_POINT ( 'NONE',  ( 35.15837367389831769, -19.43146302041509443, -19.19767279675701488 ) ) ;
#24021=CARTESIAN_POINT ( 'NONE',  ( 20.99533150354982070, 4.487273811465053441, -19.54336078777620500 ) ) ;
#24025=CARTESIAN_POINT ( 'NONE',  ( 17.46151185945609186, 6.859213057953727599, -13.86392132274949418 ) ) ;
#24030=CARTESIAN_POINT ( 'NONE',  ( 21.56383972367567736, -3.323709001909281202, -18.92284382192250192 ) ) ;
#24031=CARTESIAN_POINT ( 'NONE',  ( 16.25879716139461095, 4.256374150336979412, -17.55500201710977137 ) ) ;
#24040=CARTESIAN_POINT ( 'NONE',  ( 9.981537699549546616, 16.10875070413535681, -16.47763325427154868 ) ) ;
#24041=CARTESIAN_POINT ( 'NONE',  ( 28.32023557703361405, -7.180604414193060059, -17.61256657898508138 ) ) ;
#24042=CARTESIAN_POINT ( 'NONE',  ( 26.42570577731286718, -9.588051360687080305, -12.79080846482418643 ) ) ;
#24044=CARTESIAN_POINT ( 'NONE',  ( 32.12153525177792091, -10.97127362787143312, -16.88978156643115724 ) ) ;
#24052=CARTESIAN_POINT ( 'NONE',  ( 21.64656857049893901, 5.639188926465734220, -17.17864421186117951 ) ) ;
#24055=CARTESIAN_POINT ( 'NONE',  ( 12.26606010314042017, 9.512972848517913249, -15.31757320754432605 ) ) ;
#24058=CARTESIAN_POINT ( 'NONE',  ( 18.04049687913209610, 0.8262538513465327306, -14.27019888128743297 ) ) ;
#24059=CARTESIAN_POINT ( 'NONE',  ( 22.63682584648026008, 4.680144189823682410, -16.86151017930854223 ) ) ;
#24062=CARTESIAN_POINT ( 'NONE',  ( 35.52583876341286384, -22.08228901593173177, -18.97221062538168113 ) ) ;
#24063=CARTESIAN_POINT ( 'NONE',  ( 24.27832910178602788, -5.559203070376852018, -13.12236226054620047 ) ) ;
#24064=CARTESIAN_POINT ( 'NONE',  ( 20.25556019283287768, 3.967930604842117681, -18.44304694949289569 ) ) ;
#24074=CARTESIAN_POINT ( 'NONE',  ( 36.44920892064849482, -21.73803172434679354, -19.68085951391205057 ) ) ;
#24075=CARTESIAN_POINT ( 'NONE',  ( 9.910898653440767703, 16.43271037397421708, -16.50709950392603531 ) ) ;
#24080=CARTESIAN_POINT ( 'NONE',  ( 12.02908293258818517, 9.311337566433326884, -16.69090174519279657 ) ) ;
#24090=CARTESIAN_POINT ( 'NONE',  ( 11.22336320048417591, 9.093679674329528950, -17.24182414271593800 ) ) ;
#24091=CARTESIAN_POINT ( 'NONE',  ( 25.18430082464795916, -12.47910854170484818, -17.34997305645471855 ) ) ;
#24092=CARTESIAN_POINT ( 'NONE',  ( 23.76385019584477831, -1.264968635605209446, -19.12809044524397351 ) ) ;
#24103=CARTESIAN_POINT ( 'NONE',  ( 11.76876341733043141, 10.50516141373230106, -16.79855566342228101 ) ) ;
#24106=CARTESIAN_POINT ( 'NONE',  ( 35.54859390953724585, -22.18451583373416014, -18.06010107863414405 ) ) ;
#24108=CARTESIAN_POINT ( 'NONE',  ( 8.944584683310379702, 16.95159276115599667, -17.92454625180715411 ) ) ;
#24111=CARTESIAN_POINT ( 'NONE',  ( 23.22413189157496305, -7.367447486509826504, -15.63851824576001981 ) ) ;
#24112=CARTESIAN_POINT ( 'NONE',  ( 12.83220575256047802, 9.540835953717470730, -16.14105854569320542 ) ) ;
#24116=CARTESIAN_POINT ( 'NONE',  ( 11.48890098693651396, 9.204103201752445784, -15.85365151319587440 ) ) ;
#24119=CARTESIAN_POINT ( 'NONE',  ( 11.48890098693651396, 9.204103201752445784, -15.85365151319587440 ) ) ;
#24124=CARTESIAN_POINT ( 'NONE',  ( 12.02761088988360783, 9.318053909225662679, -16.69151312802368636 ) ) ;
#24126=CARTESIAN_POINT ( 'NONE',  ( 36.54859390953724585, -23.18451583373416014, -18.06010107863414405 ) ) ;
#24127=CARTESIAN_POINT ( 'NONE',  ( 29.88803641097454999, -7.968445601786871002, -16.75847372370488131 ) ) ;
#24128=CARTESIAN_POINT ( 'NONE',  ( 13.51959648670337444, 7.024181567627514333, -18.72314150793285492 ) ) ;
#24134=CARTESIAN_POINT ( 'NONE',  ( 20.55682936838109498, 0.8107970201405315658, -19.60370085144657182 ) ) ;
#24135=CARTESIAN_POINT ( 'NONE',  ( 15.93484470893836935, 6.939319753835953009, -14.67888072223970752 ) ) ;
#24145=CARTESIAN_POINT ( 'NONE',  ( 12.27670864112623583, 9.495496515443743846, -15.31077793565516565 ) ) ;
#24151=CARTESIAN_POINT ( 'NONE',  ( 11.49350937636955372, 9.187954247928445284, -15.85136552863131421 ) ) ;
#24153=CARTESIAN_POINT ( 'NONE',  ( 17.21229802721762780, 1.518872817929493912, -15.34595729721386448 ) ) ;
#24159=CARTESIAN_POINT ( 'NONE',  ( 12.84980237226573863, 9.516412629723424388, -16.12948954962132575 ) ) ;
#24160=CARTESIAN_POINT ( 'NONE',  ( 35.71575670127456448, -17.44301942315582110, -19.29589553906783905 ) ) ;
#24161=CARTESIAN_POINT ( 'NONE',  ( 15.41431293496917121, 3.575304669039410133, -17.09800041271234150 ) ) ;
#24167=CARTESIAN_POINT ( 'NONE',  ( 14.59671049609067950, 6.266606045730605423, -20.00302036566705155 ) ) ;
#24170=CARTESIAN_POINT ( 'NONE',  ( 20.75491211191951635, -1.144232541536293946, -14.27023797479654554 ) ) ;
#24171=CARTESIAN_POINT ( 'NONE',  ( 20.59810038911313157, 5.339108984243529754, -18.13170489685289510 ) ) ;
#24185=CARTESIAN_POINT ( 'NONE',  ( 11.77869587587188249, 8.711114196793760200, -15.67004689359726299 ) ) ;
#24187=CARTESIAN_POINT ( 'NONE',  ( 25.90061519764796572, -9.523157571424881951, -17.57609359838447816 ) ) ;
#24188=CARTESIAN_POINT ( 'NONE',  ( 25.05301747714807448, -9.477991407908255894, -18.78921932654604632 ) ) ;
#24189=CARTESIAN_POINT ( 'NONE',  ( 32.52799721746220740, -11.03300674309804386, -18.03857687357939099 ) ) ;
#24197=CARTESIAN_POINT ( 'NONE',  ( 19.71807001554888217, -1.708786246101231532, -19.21472004699903380 ) ) ;
#24200=CARTESIAN_POINT ( 'NONE',  ( 10.74108227847380448, 16.53813910199176007, -15.94580854828543437 ) ) ;
#24201=CARTESIAN_POINT ( 'NONE',  ( 32.96569147872224903, -11.36116021242123608, -19.12347989294568151 ) ) ;
#24204=CARTESIAN_POINT ( 'NONE',  ( 25.36810815240369621, -0.9165050883202133791, -18.11329069065276443 ) ) ;
#24205=CARTESIAN_POINT ( 'NONE',  ( 18.57670912428364574, -0.2836015139962214660, -15.28694485256269608 ) ) ;
#24207=CARTESIAN_POINT ( 'NONE',  ( 35.18065281855160720, -20.53155141575438591, -20.22037173032050461 ) ) ;
#24209=CARTESIAN_POINT ( 'NONE',  ( 23.29143545295710638, -10.05536756138072718, -15.72373794962660831 ) ) ;
#24211=CARTESIAN_POINT ( 'NONE',  ( 26.15289264771154620, -4.614421047071551207, -20.21764904625508663 ) ) ;
#24214=CARTESIAN_POINT ( 'NONE',  ( 23.29338531092689735, -7.078548041224526521, -17.51562821661096336 ) ) ;
#24224=CARTESIAN_POINT ( 'NONE',  ( 18.04976943019953239, 10.79320383120880145, -15.74583687248850161 ) ) ;
#24225=CARTESIAN_POINT ( 'NONE',  ( 36.13838427452936486, -20.34166123773320578, -20.43658233646779365 ) ) ;
#24227=CARTESIAN_POINT ( 'NONE',  ( 9.916118674515717046, 16.40877069192658055, -16.50468880802031890 ) ) ;
#24230=CARTESIAN_POINT ( 'NONE',  ( 12.02305193244137449, 9.338961869187645704, -16.69339841729684437 ) ) ;
#24239=CARTESIAN_POINT ( 'NONE',  ( 11.22458689634746776, 9.088074461393535586, -17.24131758186684138 ) ) ;
#24240=CARTESIAN_POINT ( 'NONE',  ( 29.81560109580191664, -6.784977964013398477, -14.56477501241906403 ) ) ;
#24241=CARTESIAN_POINT ( 'NONE',  ( 24.14852421541024441, 0.2028892341458684023, -15.23052705399570428 ) ) ;
#24256=CARTESIAN_POINT ( 'NONE',  ( 12.02908293258818517, 9.311337566433326884, -16.69090174519279657 ) ) ;
#24257=CARTESIAN_POINT ( 'NONE',  ( 33.23402178976249388, -11.79005478413273522, -18.03234444571244666 ) ) ;
#24259=CARTESIAN_POINT ( 'NONE',  ( 8.952973202525470242, 16.91312194274802749, -17.65238394630757313 ) ) ;
#24261=CARTESIAN_POINT ( 'NONE',  ( 26.84970692451943819, -5.812874930055231815, -14.04107299160273037 ) ) ;
#24262=CARTESIAN_POINT ( 'NONE',  ( 12.85536779349230052, 9.514564043964993445, -16.12538237964846388 ) ) ;
#24264=VERTEX_POINT ( 'NONE', #1416 ) ;
#24267=CARTESIAN_POINT ( 'NONE',  ( 11.47029057985033340, 9.281140223223081520, -15.86198156829250117 ) ) ;
#24271=ORIENTED_EDGE ( 'NONE', *, *, #1414, .F. ) ;
#24272=CARTESIAN_POINT ( 'NONE',  ( 11.96327893486549776, 9.613088455355432771, -16.71811665443363992 ) ) ;
#24274=CARTESIAN_POINT ( 'NONE',  ( 18.68383238644686273, 8.832144196210188980, -14.76942027321762119 ) ) ;
#24275=CARTESIAN_POINT ( 'NONE',  ( 31.81434894052502571, -10.04473835610349575, -15.03854332269495764 ) ) ;
#24282=CARTESIAN_POINT ( 'NONE',  ( 20.63695664501197413, 4.642632487595073520, -17.05591670970450124 ) ) ;
#24284=CARTESIAN_POINT ( 'NONE',  ( 17.69365662292968366, 10.27476822432933545, -17.01437286930526227 ) ) ;
#24292=CARTESIAN_POINT ( 'NONE',  ( 12.27662779141079596, 9.495931643136637845, -15.31080646268338974 ) ) ;
#24296=CARTESIAN_POINT ( 'NONE',  ( 11.47511325496290624, 9.259230714725578792, -15.85997136665693041 ) ) ;
#24299=CARTESIAN_POINT ( 'NONE',  ( 10.66893569228806271, 9.043500038842159583, -16.41109624600252559 ) ) ;
#24306=CARTESIAN_POINT ( 'NONE',  ( 12.83230269852989203, 9.540395929213350001, -16.14101810565610151 ) ) ;
#24308=CARTESIAN_POINT ( 'NONE',  ( 34.04598001273328833, -11.17175086900407166, -18.07582794505754364 ) ) ;
#24309=CARTESIAN_POINT ( 'NONE',  ( 15.70491959545049987, 3.570626008024105680, -15.63470537622339229 ) ) ;
#24313=CARTESIAN_POINT ( 'NONE',  ( 20.37871551743239351, 7.600776799596193456, -17.08157252577618479 ) ) ;
#24319=CARTESIAN_POINT ( 'NONE',  ( 23.39789874936200320, -0.01207823811560896493, -14.43595595811700782 ) ) ;
#24321=CARTESIAN_POINT ( 'NONE',  ( 18.80130396411469462, -1.975481315223051704, -14.30362724594584378 ) ) ;
#24331=CARTESIAN_POINT ( 'NONE',  ( 9.932908820165812003, 16.33176894372950727, -16.49774300651844072 ) ) ;
#24333=CARTESIAN_POINT ( 'NONE',  ( 29.36168402625536444, -8.616725751243539122, -15.73432514746931155 ) ) ;
#24334=CARTESIAN_POINT ( 'NONE',  ( 29.00434111665888182, -5.389956126880047549, -17.18324766788818181 ) ) ;
#24340=CARTESIAN_POINT ( 'NONE',  ( 23.16390915794477223, 2.882539813099532555, -14.99485278278146438 ) ) ;
#24343=CARTESIAN_POINT ( 'NONE',  ( 12.27662779141079596, 9.495931643136637845, -15.31080646268338974 ) ) ;
#24344=CARTESIAN_POINT ( 'NONE',  ( 31.39893620166130717, -10.86152586746012183, -14.84747879817187943 ) ) ;
#24347=CARTESIAN_POINT ( 'NONE',  ( 19.18841159021359033, -2.222386543571284179, -18.22349448661670834 ) ) ;
#24349=CARTESIAN_POINT ( 'NONE',  ( 22.38244025736702625, 4.876565640102752397, -15.59977576251379539 ) ) ;
#24354=CARTESIAN_POINT ( 'NONE',  ( 27.13218800474287207, -6.260320175479137106, -19.66075965151719984 ) ) ;
#24355=CARTESIAN_POINT ( 'NONE',  ( 24.97326132480219485, 0.3353791038140019887, -18.64228740943764961 ) ) ;
#24362=CARTESIAN_POINT ( 'NONE',  ( 27.26129135193747999, -10.77754955263135095, -18.64424489656416739 ) ) ;
#24368=CARTESIAN_POINT ( 'NONE',  ( 13.93491968177131923, 5.624373287173536795, -18.66784319378200863 ) ) ;
#24369=CARTESIAN_POINT ( 'NONE',  ( 36.35800453371076202, -21.32829872614925648, -20.07395605779921155 ) ) ;
#24371=CARTESIAN_POINT ( 'NONE',  ( 11.45661370752365116, 9.343864103108954211, -15.86763743611193789 ) ) ;
#24375=CARTESIAN_POINT ( 'NONE',  ( 13.12723341905928898, 8.572452836447732594, -15.90902281579132449 ) ) ;
#24385=CARTESIAN_POINT ( 'NONE',  ( 11.22390034614927856, 9.091215689738174177, -17.24160205726399653 ) ) ;
#24387=CARTESIAN_POINT ( 'NONE',  ( 30.75621536574076487, -10.42133643238263829, -12.14063830390948517 ) ) ;
#24390=CARTESIAN_POINT ( 'NONE',  ( 22.75855789899217640, -7.280205122891536540, -14.30210469086359915 ) ) ;
#24406=CARTESIAN_POINT ( 'NONE',  ( 12.50603416232391929, 8.608717614871036261, -16.38042650914619358 ) ) ;
#24407=CARTESIAN_POINT ( 'NONE',  ( 33.20927704557755789, -11.78629111679139996, -17.96241082601573424 ) ) ;
#24410=CARTESIAN_POINT ( 'NONE',  ( 9.101278670497288559, 16.23297416207913813, -17.06093009358445300 ) ) ;
#24411=CARTESIAN_POINT ( 'NONE',  ( 25.04068920418659161, -5.475481712173364990, -18.92835678451453774 ) ) ;
#24412=CARTESIAN_POINT ( 'NONE',  ( 10.35864953657871190, 16.97212341857210660, -17.91436492910080247 ) ) ;
#24418=CARTESIAN_POINT ( 'NONE',  ( 12.49957999542663600, 8.570517509188613658, -15.13050969259218981 ) ) ;
#24423=CARTESIAN_POINT ( 'NONE',  ( 13.01452397926061089, 8.532813591658360508, -15.99807864679971026 ) ) ;
#24425=CARTESIAN_POINT ( 'NONE',  ( 22.44359388949645151, 4.989503210053415572, -18.93028356096972686 ) ) ;
#24426=CARTESIAN_POINT ( 'NONE',  ( 20.05201200715256249, 8.675301412908657639, -18.33989206490851842 ) ) ;
#24428=ORIENTED_EDGE ( 'NONE', *, *, #29650, .T. ) ;
#24429=CARTESIAN_POINT ( 'NONE',  ( 35.70376052765831787, -18.38912696963886617, -20.33459093173238941 ) ) ;
#24434=CARTESIAN_POINT ( 'NONE',  ( 19.51440197245297270, 8.071880087464508691, -17.28625796899888201 ) ) ;
#24438=CARTESIAN_POINT ( 'NONE',  ( 34.11209566957792561, -15.73109017586260272, -19.92372960426217787 ) ) ;
#24442=CARTESIAN_POINT ( 'NONE',  ( 12.23642031952448406, 9.680328234467932447, -15.32743366668982432 ) ) ;
#24448=CARTESIAN_POINT ( 'NONE',  ( 12.46899830068120352, 8.557956911948249257, -15.15481108270911825 ) ) ;
#24450=CARTESIAN_POINT ( 'NONE',  ( 12.72406076201818870, 7.612173793771704666, -14.95155764689848965 ) ) ;
#24456=CARTESIAN_POINT ( 'NONE',  ( 12.79171442625009547, 9.726534347120292523, -16.15780313276466273 ) ) ;
#24457=CARTESIAN_POINT ( 'NONE',  ( 33.63214571818804188, -11.07540017893869866, -16.92567501773416794 ) ) ;
#24458=CARTESIAN_POINT ( 'NONE',  ( 21.54098841764929873, -5.100688324319140321, -15.19385678519978633 ) ) ;
#24462=CARTESIAN_POINT ( 'NONE',  ( 25.88562516208081021, -13.15641406947225889, -17.87304489109560990 ) ) ;
#24467=CARTESIAN_POINT ( 'NONE',  ( 20.97044927184332508, -4.289323992320570156, -15.06659861376252429 ) ) ;
#24468=CARTESIAN_POINT ( 'NONE',  ( 17.21229802721762780, 1.518872817929493912, -15.34595729721386448 ) ) ;
#24479=CARTESIAN_POINT ( 'NONE',  ( 11.34314632229486364, 9.864239995495806212, -15.91456019135469013 ) ) ;
#24480=CARTESIAN_POINT ( 'NONE',  ( 15.73644607668725826, 9.740111719757674535, -14.94734896276200153 ) ) ;
#24481=CARTESIAN_POINT ( 'NONE',  ( 27.03959252790357581, -7.665547941290169476, -19.57376043866218041 ) ) ;
#24494=CARTESIAN_POINT ( 'NONE',  ( 19.23836061553175369, 5.151828676608854352, -13.99136221198299168 ) ) ;
#24498=CARTESIAN_POINT ( 'NONE',  ( 12.27693553943969818, 9.494520259125854622, -15.31067919898749352 ) ) ;
#24503=CARTESIAN_POINT ( 'NONE',  ( 22.39939798857497877, 2.694615832958070722, -14.02792042734668065 ) ) ;
#24505=CARTESIAN_POINT ( 'NONE',  ( 15.19363621961471722, 2.181190162186355419, -17.24139079752846015 ) ) ;
#24508=CARTESIAN_POINT ( 'NONE',  ( 24.09482019364002880, -4.431952660107454811, -19.05667854325333721 ) ) ;
#24510=CARTESIAN_POINT ( 'NONE',  ( 20.25494212361869728, -4.857969563408182090, -14.64469595162225701 ) ) ;
#24519=CARTESIAN_POINT ( 'NONE',  ( 26.91914097958202845, -7.808663323052361882, -12.67700453112951209 ) ) ;
#24521=CARTESIAN_POINT ( 'NONE',  ( 34.91913293194685508, -14.86421081092256280, -20.09741683264573808 ) ) ;
#24523=CARTESIAN_POINT ( 'NONE',  ( 11.46269231744662420, 9.315986823159681407, -15.86512371708112212 ) ) ;
#24529=CARTESIAN_POINT ( 'NONE',  ( 9.661883061612440926, 16.25482663361732705, -17.92454625180715411 ) ) ;
#24541=CARTESIAN_POINT ( 'NONE',  ( 8.944584683310379702, 16.95159276115599667, -17.92454625180715411 ) ) ;
#24543=CARTESIAN_POINT ( 'NONE',  ( 17.55932102202221046, 11.64018535857498193, -15.95102284318303276 ) ) ;
#24544=CARTESIAN_POINT ( 'NONE',  ( 23.87675077653036126, -6.787291307973906562, -13.16608595595566733 ) ) ;
#24555=CARTESIAN_POINT ( 'NONE',  ( 13.06976498004312326, 8.549601185932660385, -15.95463209657921055 ) ) ;
#24556=CARTESIAN_POINT ( 'NONE',  ( 35.53434814243864537, -22.12051714835155281, -18.84852710552948096 ) ) ;
#24558=CARTESIAN_POINT ( 'NONE',  ( 10.58765414998594245, 9.416266744339480965, -16.44470908465386572 ) ) ;
#24562=CARTESIAN_POINT ( 'NONE',  ( 22.51149892830068211, -1.106640851078940502, -13.23823320067571885 ) ) ;
#24564=CARTESIAN_POINT ( 'NONE',  ( 12.87180867969543385, 9.517605834602926862, -16.11260084161717998 ) ) ;
#24571=CARTESIAN_POINT ( 'NONE',  ( 11.45256130090833935, 9.362448956408465861, -15.86931324879919991 ) ) ;
#24576=CARTESIAN_POINT ( 'NONE',  ( 9.661883062155979474, 16.25482663112457971, -17.91578995581314260 ) ) ;
#24578=CARTESIAN_POINT ( 'NONE',  ( 13.44640266258695327, 6.638963897028184569, -16.15403403936744198 ) ) ;
#24579=CARTESIAN_POINT ( 'NONE',  ( 21.84805831652669283, 4.237162156985878170, -20.00989837289113282 ) ) ;
#24582=CARTESIAN_POINT ( 'NONE',  ( 36.54859390953724585, -22.18451583373416014, -18.06010107863414405 ) ) ;
#24583=CARTESIAN_POINT ( 'NONE',  ( 15.39489021548154568, 6.697694061803245447, -14.95590323207311734 ) ) ;
#24588=CARTESIAN_POINT ( 'NONE',  ( 33.48796008207983022, -12.92717959506727965, -19.73506838908087246 ) ) ;
#24593=CARTESIAN_POINT ( 'NONE',  ( 11.05541599318665469, 17.68942028772053376, -17.91303167831651422 ) ) ;
#24600=CARTESIAN_POINT ( 'NONE',  ( 12.74802704355670535, 7.622310320333636646, -14.93249076938322162 ) ) ;
#24606=CARTESIAN_POINT ( 'NONE',  ( 12.83388176712078810, 9.535019011556107316, -16.14022287234750408 ) ) ;
#24607=CARTESIAN_POINT ( 'NONE',  ( 33.96051107771264554, -11.12695408846492739, -17.85276550113785277 ) ) ;
#24608=CARTESIAN_POINT ( 'NONE',  ( 18.34549112274340033, 0.9605221043122941227, -13.99314825615798341 ) ) ;
#24612=CARTESIAN_POINT ( 'NONE',  ( 14.06424326207706699, 5.752694757912038881, -19.02294901845717945 ) ) ;
#24615=CARTESIAN_POINT ( 'NONE',  ( 27.50962693642323131, -9.092369620780022643, -12.61635453147917474 ) ) ;
#24616=CARTESIAN_POINT ( 'NONE',  ( 19.45720675144774603, -0.6714082060231494342, -20.03460252700725519 ) ) ;
#24628=CARTESIAN_POINT ( 'NONE',  ( 13.34629304935920757, 7.611730149031187054, -15.73439023580873730 ) ) ;
#24629=CARTESIAN_POINT ( 'NONE',  ( 10.33811693838771717, 18.38618951776012267, -17.94384837343789130 ) ) ;
#24630=CARTESIAN_POINT ( 'NONE',  ( 28.02603357813017482, -6.678172375388682802, -19.11289830413424440 ) ) ;
#24639=CARTESIAN_POINT ( 'NONE',  ( 26.58455406938135468, -5.910422570377376950, -13.89432871846328688 ) ) ;
#24643=CARTESIAN_POINT ( 'NONE',  ( 10.98017426877725811, 15.44163275732038443, -15.84693559973663035 ) ) ;
#24644=CARTESIAN_POINT ( 'NONE',  ( 32.63711423693117553, -11.05166607373017484, -18.34576405707344549 ) ) ;
#24647=CARTESIAN_POINT ( 'NONE',  ( 27.21278356834291756, -7.014839303453253905, -18.45691071023835761 ) ) ;
#24649=CARTESIAN_POINT ( 'NONE',  ( 20.32371149932726695, 7.300285753667301591, -19.85501735805741319 ) ) ;
#24651=CARTESIAN_POINT ( 'NONE',  ( 35.54859390953724585, -22.18451583373416014, -17.99055332684694974 ) ) ;
#24654=CARTESIAN_POINT ( 'NONE',  ( 27.46460276834485370, -5.912627539431687396, -19.42860466253708296 ) ) ;
#24655=CARTESIAN_POINT ( 'NONE',  ( 26.13670795350922660, -6.813068953109826076, -12.41955265015470999 ) ) ;
#24673=CARTESIAN_POINT ( 'NONE',  ( 26.12748305362656254, -5.066878407431925524, -14.17679521427828071 ) ) ;
#24675=CARTESIAN_POINT ( 'NONE',  ( 31.25429145842602452, -9.414624517878500853, -14.20845315089566441 ) ) ;
#24677=CARTESIAN_POINT ( 'NONE',  ( 9.913797604922770290, 16.41941541294738727, -16.50570979788118464 ) ) ;
#24681=CARTESIAN_POINT ( 'NONE',  ( 9.661883061612440926, 16.25482663361732705, -17.91752729848688830 ) ) ;
#24684=CARTESIAN_POINT ( 'NONE',  ( 11.47372892693763902, 9.265404009280679531, -15.86055721330185619 ) ) ;
#24693=CARTESIAN_POINT ( 'NONE',  ( 8.944584683310379702, 16.95159276115599667, -17.92015940598198753 ) ) ;
#24694=CARTESIAN_POINT ( 'NONE',  ( 36.26977878907645447, -21.93194718998534753, -20.87741241889870736 ) ) ;
#24695=CARTESIAN_POINT ( 'NONE',  ( 16.48605814428184857, 11.34583003460130435, -14.75612992736757256 ) ) ;
#24696=CARTESIAN_POINT ( 'NONE',  ( 29.49448338005720416, -10.05855281841770221, -18.88094824714235642 ) ) ;
#24712=CARTESIAN_POINT ( 'NONE',  ( 13.17827647522021906, 8.595009676161804890, -15.86834059905992511 ) ) ;
#24713=CARTESIAN_POINT ( 'NONE',  ( 35.54859390953724585, -21.18451583373416014, -18.19919658220850422 ) ) ;
#24715=CARTESIAN_POINT ( 'NONE',  ( 9.112530393872706469, 16.18137232441842954, -17.05472470070859714 ) ) ;
#24718=CARTESIAN_POINT ( 'NONE',  ( 28.47856004806874353, -11.16640101040803401, -12.66155532224275149 ) ) ;
#24719=CARTESIAN_POINT ( 'NONE',  ( 10.35864918915110877, 16.97212501191939538, -17.94384837343789485 ) ) ;
#24725=CARTESIAN_POINT ( 'NONE',  ( 11.47257016429183452, 9.270685755423764718, -15.86103888016343255 ) ) ;
#24729=CARTESIAN_POINT ( 'NONE',  ( 13.34161425493533315, 8.667191563245470576, -15.73815750552000381 ) ) ;
#24731=CARTESIAN_POINT ( 'NONE',  ( 17.13759149762038803, 5.494404601539362609, -21.09448147619161418 ) ) ;
#24732=CARTESIAN_POINT ( 'NONE',  ( 14.60232135752762517, 2.980368010496468933, -17.13315712471359475 ) ) ;
#24735=CARTESIAN_POINT ( 'NONE',  ( 36.53271160917758209, -22.11316507130252873, -18.90714217169671230 ) ) ;
#24737=CARTESIAN_POINT ( 'NONE',  ( 24.79644250101478065, -1.608028467720058918, -19.02763285027648976 ) ) ;
#24747=CARTESIAN_POINT ( 'NONE',  ( 33.10952763335142635, -11.62914684427059697, -19.38687730282833499 ) ) ;
#24752=PRODUCT_DEFINITION_CONTEXT ( 'detailed design', #28058, 'design' ) ;
#24753=CARTESIAN_POINT ( 'NONE',  ( 16.59405769476016701, 11.43796928512929867, -11.86713876492064124 ) ) ;
#24754=CARTESIAN_POINT ( 'NONE',  ( 32.30218501430429967, -10.99871056796995816, -17.40035725849610060 ) ) ;
#24759=CARTESIAN_POINT ( 'NONE',  ( 10.66616952815763320, 9.056185211661334833, -16.41224021383828102 ) ) ;
#24763=CARTESIAN_POINT ( 'NONE',  ( 14.75361449413180637, 10.34920949090176201, -14.61276839131081218 ) ) ;
#24764=CARTESIAN_POINT ( 'NONE',  ( 33.87301206822314725, -11.11198276574163302, -17.60644260715651299 ) ) ;
#24765=CARTESIAN_POINT ( 'NONE',  ( 25.36810815240369621, -0.9165050883202133791, -18.11329069065276443 ) ) ;
#24772=CARTESIAN_POINT ( 'NONE',  ( 24.51672896724849338, -10.45039314358892035, -14.45231470433035170 ) ) ;
#24774=CARTESIAN_POINT ( 'NONE',  ( 21.18694592818775746, 3.276320881159561438, -13.81383015674761339 ) ) ;
#24785=CARTESIAN_POINT ( 'NONE',  ( 11.40026617402801179, 8.559985368287675200, -17.14749594687102174 ) ) ;
#24786=CARTESIAN_POINT ( 'NONE',  ( 12.39803340617553928, 8.535179507765855433, -15.21071672276548625 ) ) ;
#24793=CARTESIAN_POINT ( 'NONE',  ( 9.641350810849047548, 17.66889113945805789, -17.91752729848689185 ) ) ;
#24796=CARTESIAN_POINT ( 'NONE',  ( 24.14317479683219858, -6.286850201977149055, -18.60698471650063723 ) ) ;
#24800=CARTESIAN_POINT ( 'NONE',  ( 11.05541531668977662, 17.68942339022145305, -17.93331994345748726 ) ) ;
#24807=CARTESIAN_POINT ( 'NONE',  ( 23.29338531092689735, -7.078548041224526521, -17.51562821661096336 ) ) ;
#24809=CARTESIAN_POINT ( 'NONE',  ( 22.26732294003774015, -3.469656073077215463, -14.71322089325822624 ) ) ;
#24812=CARTESIAN_POINT ( 'NONE',  ( 19.42071131597032974, 7.574497315622086724, -15.00200944635056644 ) ) ;
#24813=CARTESIAN_POINT ( 'NONE',  ( 20.76230466941008146, -3.840972149463459218, -19.45223659164069474 ) ) ;
#24816=CARTESIAN_POINT ( 'NONE',  ( 31.81434894052502571, -10.04473835610349575, -15.03854332269495764 ) ) ;
#24825=CARTESIAN_POINT ( 'NONE',  ( 26.63310354640557520, -6.268104337495945977, -18.78393408973622769 ) ) ;
#24826=CARTESIAN_POINT ( 'NONE',  ( 21.10828700581006601, 3.717818950362942854, -18.90958453460783417 ) ) ;
#24827=CARTESIAN_POINT ( 'NONE',  ( 36.54859390954303677, -22.18451583373416014, -15.55638201429745848 ) ) ;
#24829=CARTESIAN_POINT ( 'NONE',  ( 12.49664108868010182, 8.569232744350554043, -15.13285098609708790 ) ) ;
#24832=CARTESIAN_POINT ( 'NONE',  ( 13.34161425493533315, 8.667191563245470576, -15.73815750552000381 ) ) ;
#24835=CARTESIAN_POINT ( 'NONE',  ( 11.47257016429183452, 9.270685755423764718, -15.86103888016343255 ) ) ;
#24844=CIRCLE ( 'NONE', #7294, 0.4999999999999986677 ) ;
#24846=CARTESIAN_POINT ( 'NONE',  ( 8.944617638130560877, 16.95144162614991501, -17.89908301402565982 ) ) ;
#24847=CARTESIAN_POINT ( 'NONE',  ( 36.54859105337858693, -23.18450300252589003, -18.42496455282032386 ) ) ;
#24849=CARTESIAN_POINT ( 'NONE',  ( 18.57953865233433532, 8.080199298666570940, -13.63460617990120838 ) ) ;
#24850=CARTESIAN_POINT ( 'NONE',  ( 27.87518295380144551, -11.54787579004265652, -18.81772651352153858 ) ) ;
#24854=CARTESIAN_POINT ( 'NONE',  ( 22.48601049859325585, 2.925819830077934558, -17.76611561182923893 ) ) ;
#24865=CARTESIAN_POINT ( 'NONE',  ( 12.84373479294319864, 8.511860559062048637, -16.13004233893675377 ) ) ;
#24866=CARTESIAN_POINT ( 'NONE',  ( 35.54859390953724585, -21.18451583373416014, -17.22552805718784441 ) ) ;
#24868=CARTESIAN_POINT ( 'NONE',  ( 10.62817821613907476, 9.230418211344437296, -16.42795095778131298 ) ) ;
#24870=CARTESIAN_POINT ( 'NONE',  ( 24.87127057246125972, -9.548149280147088191, -14.79180087847266556 ) ) ;
#24871=CARTESIAN_POINT ( 'NONE',  ( 12.90243451339205194, 9.531139938431367753, -16.08819151157827321 ) ) ;
#24884=CARTESIAN_POINT ( 'NONE',  ( 13.39606018151479461, 8.691252192278360766, -15.69476314099692971 ) ) ;
#24886=CARTESIAN_POINT ( 'NONE',  ( 16.96299543436377633, 3.857017182823994084, -13.23919852190412527 ) ) ;
#24887=CARTESIAN_POINT ( 'NONE',  ( 17.83966564144121136, 6.109271821037239647, -21.09843361817607388 ) ) ;
#24892=CARTESIAN_POINT ( 'NONE',  ( 19.61192361542596529, -2.405681417800469291, -14.70675912396028906 ) ) ;
#24899=CARTESIAN_POINT ( 'NONE',  ( 34.82539348385352440, -18.93555941106099993, -20.13934242161363741 ) ) ;
#24904=CARTESIAN_POINT ( 'NONE',  ( 12.24532799939971284, 9.516186676127107447, -15.33315318048745013 ) ) ;
#24905=CARTESIAN_POINT ( 'NONE',  ( 35.54859390953724585, -23.18451583373416014, -17.99055332684694974 ) ) ;
#24909=CARTESIAN_POINT ( 'NONE',  ( 11.28991474634619863, 7.910464746135025926, -16.02350989558273753 ) ) ;
#24918=CARTESIAN_POINT ( 'NONE',  ( 10.35864918915110877, 16.97212501191939538, -17.91752729848689185 ) ) ;
#24920=CARTESIAN_POINT ( 'NONE',  ( 34.41982446195410716, -12.62108234628556680, -19.94648786050102274 ) ) ;
#24922=CARTESIAN_POINT ( 'NONE',  ( 23.86551563699305234, 2.542095107771292106, -17.79649620197707094 ) ) ;
#24928=CARTESIAN_POINT ( 'NONE',  ( 29.30807694892355286, -8.357723062633453992, -13.20244061823602522 ) ) ;
#24929=CARTESIAN_POINT ( 'NONE',  ( 23.94974919959990345, -8.117095362258064384, -14.41405346848900848 ) ) ;
#24940=CARTESIAN_POINT ( 'NONE',  ( 11.22387317355479475, 9.091340879052031809, -17.24161325043666082 ) ) ;
#24941=CARTESIAN_POINT ( 'NONE',  ( 10.33811693838771717, 18.38618951776012267, -17.93331994345748726 ) ) ;
#24947=CARTESIAN_POINT ( 'NONE',  ( 9.641350777746193756, 17.66889129127197577, -17.91630266473768884 ) ) ;
#24953=CARTESIAN_POINT ( 'NONE',  ( 25.21413058671614849, -1.115224416820481457, -18.44856734933592080 ) ) ;
#24958=CARTESIAN_POINT ( 'NONE',  ( 12.25364105430271700, 9.519861518574414205, -15.32652744092241726 ) ) ;
#24959=CARTESIAN_POINT ( 'NONE',  ( 33.14486676600987636, -11.77651092997264293, -17.78036478212233717 ) ) ;
#24961=CARTESIAN_POINT ( 'NONE',  ( 28.15048769591263067, -5.842385520647848551, -16.89978903947823241 ) ) ;
#24963=CARTESIAN_POINT ( 'NONE',  ( 24.04487210496366245, -0.6674514567044148583, -16.01806975046538284 ) ) ;
#24968=SURFACE_STYLE_FILL_AREA ( #22969 ) ;
#24969=CARTESIAN_POINT ( 'NONE',  ( 13.93491968177131923, 5.624373287173536795, -18.66784319378200863 ) ) ;
#24970=CARTESIAN_POINT ( 'NONE',  ( 29.99716341122577745, -11.34936846952144585, -14.08097903537201212 ) ) ;
#24972=CARTESIAN_POINT ( 'NONE',  ( 26.57062215293289498, -11.41726559881178638, -18.09730928560479057 ) ) ;
#24973=PRODUCT_DEFINITION_SHAPE ( 'NONE', 'NONE',  #11917 ) ;
#24981=CARTESIAN_POINT ( 'NONE',  ( 27.63487812444411418, -5.020849242181972372, -17.14317672846274831 ) ) ;
#24982=CARTESIAN_POINT ( 'NONE',  ( 16.29141254853644227, 2.771581735061156682, -15.76764191790683611 ) ) ;
#24983=CARTESIAN_POINT ( 'NONE',  ( 34.30083361619418980, -13.08651950748960680, -20.95284133056243192 ) ) ;
#24986=CARTESIAN_POINT ( 'NONE',  ( 11.97192087863669663, 8.579774655713777065, -15.53257280409644991 ) ) ;
#24989=CARTESIAN_POINT ( 'NONE',  ( 9.661883066202028303, 16.25482661256886630, -17.91573536996246929 ) ) ;
#24993=CARTESIAN_POINT ( 'NONE',  ( 12.49664108868010182, 8.569232744350554043, -15.13285098609708790 ) ) ;
#25000=CARTESIAN_POINT ( 'NONE',  ( 13.39286676965551059, 7.631811206235384226, -15.69730834661896424 ) ) ;
#25001=CARTESIAN_POINT ( 'NONE',  ( 36.19022241692326247, -21.57454255207833071, -21.10101832753974449 ) ) ;
#25002=CARTESIAN_POINT ( 'NONE',  ( 18.25722813608836859, -0.08152059447761372812, -18.39925177747023710 ) ) ;
#25003=CARTESIAN_POINT ( 'NONE',  ( 19.09420370221858931, 5.586061004495046056, -18.95245686415860220 ) ) ;
#25007=CARTESIAN_POINT ( 'NONE',  ( 24.91205307904067112, 1.131441846345163427, -15.76301496618838627 ) ) ;
#25014=CARTESIAN_POINT ( 'NONE',  ( 33.85795792134603488, -11.10969635406632072, -17.56389463281766439 ) ) ;
#25016=CARTESIAN_POINT ( 'NONE',  ( 10.60386377644718614, 9.341927331141327784, -16.43800583390468262 ) ) ;
#25019=CARTESIAN_POINT ( 'NONE',  ( 30.24922550192677306, -10.40856591028444278, -13.02298783260255988 ) ) ;
#25021=CARTESIAN_POINT ( 'NONE',  ( 12.87521155010636242, 9.519109623917222152, -16.10988869383489686 ) ) ;
#25026=CARTESIAN_POINT ( 'NONE',  ( 12.77278825050581013, 8.691252192278360766, -14.91275796197543890 ) ) ;
#25031=CARTESIAN_POINT ( 'NONE',  ( 9.661883061612440926, 16.25482663361732705, -17.91752729848688830 ) ) ;
#25032=CARTESIAN_POINT ( 'NONE',  ( 22.87531825017061848, 1.851759407679815173, -13.77476424085121742 ) ) ;
#25033=CARTESIAN_POINT ( 'NONE',  ( 18.23272808550097679, 0.7689261898593379163, -20.18852386690180367 ) ) ;
#25035=CARTESIAN_POINT ( 'NONE',  ( 31.84774147790582433, -10.54213090804960018, -15.00000000011102763 ) ) ;
#25037=CARTESIAN_POINT ( 'NONE',  ( 19.38992137333195842, 2.881095379261479739, -20.30776781288435373 ) ) ;
#25046=CARTESIAN_POINT ( 'NONE',  ( 10.46960557229346733, 16.46326489517938541, -17.33590790293451178 ) ) ;
#25047=CARTESIAN_POINT ( 'NONE',  ( 33.17819505895439391, -11.78846528140086924, -19.49437495119144259 ) ) ;
#25051=CARTESIAN_POINT ( 'NONE',  ( 30.71753525214919378, -10.10955902127019179, -14.92479911117869484 ) ) ;
#25052=CARTESIAN_POINT ( 'NONE',  ( 12.24503583471362234, 9.516058715885376884, -15.33338595299508889 ) ) ;
#25057=CARTESIAN_POINT ( 'NONE',  ( 12.77299770905688803, 7.633314995549595139, -14.91259101981587420 ) ) ;
#25061=CARTESIAN_POINT ( 'NONE',  ( 10.35864917552468611, 16.97212507441191320, -17.91611982430173455 ) ) ;
#25062=CARTESIAN_POINT ( 'NONE',  ( 33.68917633736438688, -10.64779379647620949, -18.96437360758372748 ) ) ;
#25063=CARTESIAN_POINT ( 'NONE',  ( 24.00918528248616468, -0.5066965781341161712, -13.81223085940890627 ) ) ;
#25067=CARTESIAN_POINT ( 'NONE',  ( 27.85014272824177795, -5.137623357037004013, -13.74226875356335320 ) ) ;
#25068=CARTESIAN_POINT ( 'NONE',  ( 24.68698569862014480, -7.792836496385216805, -13.74806253080685359 ) ) ;
#25077=CARTESIAN_POINT ( 'NONE',  ( 11.14294825671155209, 9.462472856991839265, -17.27507855072861176 ) ) ;
#25079=CARTESIAN_POINT ( 'NONE',  ( 12.50098444160134470, 8.571137227758441668, -15.12939039523150520 ) ) ;
#25084=CARTESIAN_POINT ( 'NONE',  ( 9.641352920869014298, 17.66888146263751125, -17.91030124961049097 ) ) ;
#25086=CARTESIAN_POINT ( 'NONE',  ( 30.81871029749655477, -11.10956723898439868, -14.94490981684777431 ) ) ;
#25089=CARTESIAN_POINT ( 'NONE',  ( 24.92864811393110358, -0.2441600445015326137, -14.78813717129899885 ) ) ;
#25093=CARTESIAN_POINT ( 'NONE',  ( 12.24591402697972775, 9.516428332920080280, -15.33268742708093235 ) ) ;
#25095=CARTESIAN_POINT ( 'NONE',  ( 35.18065281855160720, -20.53155141575438591, -20.22037173032050461 ) ) ;
#25097=CARTESIAN_POINT ( 'NONE',  ( 25.71553203045151292, -8.406338935355361031, -18.42709291467145150 ) ) ;
#25100=CARTESIAN_POINT ( 'NONE',  ( 20.63450008290067927, -1.653576198284400833, -18.07233451455898532 ) ) ;
#25103=CARTESIAN_POINT ( 'NONE',  ( 26.89114594638229505, -13.18314149429672000, -12.91981678032827041 ) ) ;
#25104=CARTESIAN_POINT ( 'NONE',  ( 25.09247252535503492, -10.89683230441130135, -15.98339435310939827 ) ) ;
#25106=EDGE_LOOP ( 'NONE', ( #13737, #4257, #20499, #26075, #29662 ) ) ;
#25118=CARTESIAN_POINT ( 'NONE',  ( 9.641350810849047548, 17.66889113945805789, -23.00000000000000711 ) ) ;
#25119=CARTESIAN_POINT ( 'NONE',  ( 25.82086518536678454, -3.233603117969178875, -16.21460360555060021 ) ) ;
#25120=CARTESIAN_POINT ( 'NONE',  ( 19.36978511310259421, 2.022953856625822944, -19.43459320487130171 ) ) ;
#25121=CARTESIAN_POINT ( 'NONE',  ( 32.62421882425100961, -9.622687980317111922, -18.08031881573170097 ) ) ;
#25123=CARTESIAN_POINT ( 'NONE',  ( 12.50076791318051761, 8.571041463825640250, -15.12956297801270900 ) ) ;
#25126=CARTESIAN_POINT ( 'NONE',  ( 9.678003265275730627, 16.18089732476941833, -17.88088483716984811 ) ) ;
#25131=CARTESIAN_POINT ( 'NONE',  ( 10.33811693838771717, 18.38618951776012267, -19.66666666666843000 ) ) ;
#25137=CARTESIAN_POINT ( 'NONE',  ( 8.944584683310379702, 16.95159276115599667, -19.66666666666843000 ) ) ;
#25138=CARTESIAN_POINT ( 'NONE',  ( 35.54859390953724585, -23.18451583373416014, -17.78191007148576119 ) ) ;
#25139=CARTESIAN_POINT ( 'NONE',  ( 19.82966512453777952, 6.730073478465656400, -20.48479553209826065 ) ) ;
#25141=CARTESIAN_POINT ( 'NONE',  ( 31.37220973900873489, -11.08107799475175348, -13.94606079199652982 ) ) ;
#25144=CARTESIAN_POINT ( 'NONE',  ( 20.16317987096495656, -0.6177526724804084379, -13.65447574297484223 ) ) ;
#25150=( LENGTH_UNIT ( ) NAMED_UNIT ( * ) SI_UNIT ( .MILLI., .METRE. ) );
#25156=CARTESIAN_POINT ( 'NONE',  ( 35.54686456755326418, -21.17674681625933530, -18.46270299499373735 ) ) ;
#25159=CARTESIAN_POINT ( 'NONE',  ( 12.22241433628510165, 7.513235304754858568, -15.34201686955167609 ) ) ;
#25164=CARTESIAN_POINT ( 'NONE',  ( 11.86602117609799301, 10.05912493454434120, -16.75833615892761586 ) ) ;
#25175=CARTESIAN_POINT ( 'NONE',  ( 13.15785925275590529, 8.585986940276173485, -15.88461348575242305 ) ) ;
#25177=CARTESIAN_POINT ( 'NONE',  ( 20.53425600248055005, 0.8933117467920750343, -13.02782074225586406 ) ) ;
#25178=CARTESIAN_POINT ( 'NONE',  ( 21.76882177598054113, -1.089445278190608102, -19.78435629462099854 ) ) ;
#25179=CARTESIAN_POINT ( 'NONE',  ( 18.72775033408030154, 1.433941090885695768, -19.03071139844121262 ) ) ;
#25185=CARTESIAN_POINT ( 'NONE',  ( 22.86252235622482587, -0.9498377794471745128, -13.29674124224850118 ) ) ;
#25197=CARTESIAN_POINT ( 'NONE',  ( 17.85084670134855145, 5.929878015568476712, -20.08862479909851828 ) ) ;
#25198=CARTESIAN_POINT ( 'NONE',  ( 12.29957980484737767, 9.540162674316999158, -15.28991344586433421 ) ) ;
#25199=CARTESIAN_POINT ( 'NONE',  ( 34.75406370242679799, -18.61511248754081294, -20.11778113987843852 ) ) ;
#25204=CARTESIAN_POINT ( 'NONE',  ( 9.641350810849047548, 17.66889113945805789, -17.91664992932186351 ) ) ;
#25210=CARTESIAN_POINT ( 'NONE',  ( 12.87053260329167692, 9.517041913610183812, -16.11361789703515868 ) ) ;
#25214=CARTESIAN_POINT ( 'NONE',  ( 34.31936231504242585, -12.17391896401218609, -19.91370162440023250 ) ) ;
#25215=CARTESIAN_POINT ( 'NONE',  ( 28.15048769591263067, -5.842385520647848551, -16.89978903947823241 ) ) ;
#25222=CARTESIAN_POINT ( 'NONE',  ( 22.98083118076628040, -7.181321033737746440, -13.97658420854277850 ) ) ;
#25223=CARTESIAN_POINT ( 'NONE',  ( 25.54411345550068191, -6.057473962578058035, -19.57277538061955013 ) ) ;
#25231=CARTESIAN_POINT ( 'NONE',  ( 12.53458732174692258, 8.585986940276173485, -15.10260830673100330 ) ) ;
#25236=CARTESIAN_POINT ( 'NONE',  ( 9.641350810849047548, 17.66889113945805789, -17.95086732675817132 ) ) ;
#25238=CARTESIAN_POINT ( 'NONE',  ( 27.28133297882270014, -12.52022702279392874, -15.45456112525011427 ) ) ;
#25241=CARTESIAN_POINT ( 'NONE',  ( 26.18758235895636233, -4.355437658720127558, -18.53605802859044260 ) ) ;
#25244=CARTESIAN_POINT ( 'NONE',  ( 12.25159070717542065, 9.517778977577904698, -15.32825133053543887 ) ) ;
#25248=CARTESIAN_POINT ( 'NONE',  ( 35.22227017426903473, -20.71851614966110233, -20.19360243392694088 ) ) ;
#25252=CARTESIAN_POINT ( 'NONE',  ( 24.18219217278060995, -6.970120066757704791, -14.18070892486464629 ) ) ;
#25255=CARTESIAN_POINT ( 'NONE',  ( 20.47999367081501632, -2.041782396245861442, -15.93780510180117638 ) ) ;
#25258=CARTESIAN_POINT ( 'NONE',  ( 25.88562516208081021, -13.15641406947225889, -17.87304489109560990 ) ) ;
#25259=CARTESIAN_POINT ( 'NONE',  ( 30.94061990612449264, -11.12808277128230294, -15.28946652318938959 ) ) ;
#25270=CARTESIAN_POINT ( 'NONE',  ( 23.05283280155556724, -4.691836721735100468, -12.69353859562758124 ) ) ;
#25271=CARTESIAN_POINT ( 'NONE',  ( 17.97606266963480692, 4.724414365053664966, -20.23074386977120298 ) ) ;
#25272=CARTESIAN_POINT ( 'NONE',  ( 36.54859390953723874, -22.18451583373416014, -15.00000000000000000 ) ) ;
#25274=CARTESIAN_POINT ( 'NONE',  ( 11.47231678315799464, 9.271847796573304379, -15.86114366194887815 ) ) ;
#25277=CARTESIAN_POINT ( 'NONE',  ( 9.732710754582456048, 15.93000180522596665, -17.85826136589200175 ) ) ;
#25279=EDGE_LOOP ( 'NONE', ( #21245, #18352 ) ) ;
#25281=CARTESIAN_POINT ( 'NONE',  ( 15.61762486822808604, 9.948436389806387226, -12.64537296286936829 ) ) ;
#25291=CARTESIAN_POINT ( 'NONE',  ( 9.153102208164984432, 15.99530481237056989, -17.03794677594065021 ) ) ;
#25292=CARTESIAN_POINT ( 'NONE',  ( 35.54859125455464408, -23.18450390630307822, -18.42126094939176895 ) ) ;
#25294=CARTESIAN_POINT ( 'NONE',  ( 18.57670912428364574, -0.2836015139962214660, -15.28694485256269608 ) ) ;
#25295=CARTESIAN_POINT ( 'NONE',  ( 17.54325408622900184, 7.715740848240963068, -20.30207397218512000 ) ) ;
#25298=CARTESIAN_POINT ( 'NONE',  ( 19.06759106800826586, -1.100202736525451641, -14.71838255749352165 ) ) ;
#25308=CARTESIAN_POINT ( 'NONE',  ( 35.24753590068310416, -19.83202167481471889, -19.22462439892593977 ) ) ;
#25310=CARTESIAN_POINT ( 'NONE',  ( 10.65249265583095095, 9.118909091547207524, -16.41789608165773728 ) ) ;
#25312=CARTESIAN_POINT ( 'NONE',  ( 29.90031526554274777, -7.862644070287768905, -16.42500436498598049 ) ) ;
#25314=CARTESIAN_POINT ( 'NONE',  ( 10.47175433613752027, 16.45341039028688002, -17.33491556667247835 ) ) ;
#25321=CARTESIAN_POINT ( 'NONE',  ( 12.51757296969303290, 8.578467993704791184, -15.11616904564172792 ) ) ;
#25328=CARTESIAN_POINT ( 'NONE',  ( 10.96464236563772943, 10.28020640217055259, -17.34881430896752619 ) ) ;
#25329=CARTESIAN_POINT ( 'NONE',  ( 24.32739057165333207, -2.318628849198325348, -18.36682367714799824 ) ) ;
#25330=CARTESIAN_POINT ( 'NONE',  ( 23.89160689111651337, -1.335809292830872241, -14.36923488517323477 ) ) ;
#25331=CARTESIAN_POINT ( 'NONE',  ( 21.13650371987585075, 4.769999862021419901, -15.38713752973847448 ) ) ;
#25332=DIRECTION ( 'NONE',  ( 0.3331260486002958765, -0.05059491534325381845, -0.9415238660200613285 ) ) ;
#25335=CARTESIAN_POINT ( 'NONE',  ( 24.66978787416869068, -0.3063955544261361963, -14.42797892638687784 ) ) ;
#25340=CARTESIAN_POINT ( 'NONE',  ( 10.35864918915110877, 16.97212501191939538, -17.92454625180715766 ) ) ;
#25345=CARTESIAN_POINT ( 'NONE',  ( 16.34386185847872142, 4.569898679961749366, -19.52586945278800812 ) ) ;
#25346=CARTESIAN_POINT ( 'NONE',  ( 11.05542614047498873, 17.68937375096277265, -17.90480922774079175 ) ) ;
#25351=CARTESIAN_POINT ( 'NONE',  ( 9.917332382238186028, 16.40320447359955125, -16.50418441153501448 ) ) ;
#25352=CARTESIAN_POINT ( 'NONE',  ( 9.641890818133653340, 17.66641459721583374, -17.82828029666912073 ) ) ;
#25359=CARTESIAN_POINT ( 'NONE',  ( 10.35864918915110877, 16.97212501191939538, -17.98596209335946128 ) ) ;
#25360=CARTESIAN_POINT ( 'NONE',  ( 34.28781561389841670, -12.04879923890588422, -19.89451123369701691 ) ) ;
#25361=CARTESIAN_POINT ( 'NONE',  ( 26.04489551603160180, -6.130266781319400948, -13.71289979607875154 ) ) ;
#25368=CARTESIAN_POINT ( 'NONE',  ( 14.69068284915647560, 4.968298739062387170, -17.53091140782979807 ) ) ;
#25369=CARTESIAN_POINT ( 'NONE',  ( 21.89112544314524200, -5.209854132323804343, -13.34451667507982364 ) ) ;
#25379=CARTESIAN_POINT ( 'NONE',  ( 10.78565875124225393, 16.33370571569710705, -15.92737460872590738 ) ) ;
#25380=CARTESIAN_POINT ( 'NONE',  ( 26.88053589187069292, -12.95240298029966119, -14.33176627689639382 ) ) ;
#25387=CARTESIAN_POINT ( 'NONE',  ( 11.47079713067724782, 9.278817116560638567, -15.86177209170659275 ) ) ;
#25388=CARTESIAN_POINT ( 'NONE',  ( 15.31194320040279777, 8.488938064892046498, -14.62880434596509183 ) ) ;
#25391=CARTESIAN_POINT ( 'NONE',  ( 26.87449084144840938, -11.88902188497427481, -13.49525739704605343 ) ) ;
#25395=CARTESIAN_POINT ( 'NONE',  ( 12.25193961909737794, 9.519109623917222152, -15.32788351481347355 ) ) ;
#25398=CARTESIAN_POINT ( 'NONE',  ( 35.54859390953724585, -22.18451583373416014, -17.22552805718784441 ) ) ;
#25401=CARTESIAN_POINT ( 'NONE',  ( 23.72730982194951466, -1.509008702439352589, -18.09242500859757996 ) ) ;
#25404=CARTESIAN_POINT ( 'NONE',  ( 28.55206495951409096, -10.69471729813234795, -19.99811924356017911 ) ) ;
#25405=CARTESIAN_POINT ( 'NONE',  ( 29.77493782482978091, -9.049732786019394126, -14.43420072379011643 ) ) ;
#25419=CARTESIAN_POINT ( 'NONE',  ( 18.23559491442917135, -2.176271773050306724, -15.57877364869929515 ) ) ;
#25420=CARTESIAN_POINT ( 'NONE',  ( 20.73027244251523626, 3.305903845835247434, -19.25852547563239625 ) ) ;
#25421=CARTESIAN_POINT ( 'NONE',  ( 33.08402606333302742, -12.15068820457383403, -20.63309441556253176 ) ) ;
#25423=CARTESIAN_POINT ( 'NONE',  ( 11.65548303173490652, 8.849831895876286936, -15.75351705932409985 ) ) ;
#25429=CARTESIAN_POINT ( 'NONE',  ( 12.46899830068120352, 8.557956911948249257, -15.15481108270911825 ) ) ;
#25434=FACE_OUTER_BOUND ( 'NONE', #12836, .T. ) ;
#25436=CARTESIAN_POINT ( 'NONE',  ( 9.112223960064733674, 16.18277766892301983, -17.05485288603163951 ) ) ;
#25437=CARTESIAN_POINT ( 'NONE',  ( 34.86302720852563652, -20.10462780087231138, -21.19305451400748552 ) ) ;
#25438=CARTESIAN_POINT ( 'NONE',  ( 15.95545008109832530, 6.956385541780823800, -13.20154910664163950 ) ) ;
#25439=CARTESIAN_POINT ( 'NONE',  ( 15.50826552155665183, 8.864470348925614474, -13.64319937614855149 ) ) ;
#25441=CARTESIAN_POINT ( 'NONE',  ( 25.18022790295009727, 0.7303485828293051485, -17.76052596840512621 ) ) ;
#25454=CARTESIAN_POINT ( 'NONE',  ( 36.30315773322485740, -20.08190110472122214, -19.47147371593984388 ) ) ;
#25455=CARTESIAN_POINT ( 'NONE',  ( 12.00353595525870887, 7.537035219234042849, -15.50727442731917272 ) ) ;
#25459=CARTESIAN_POINT ( 'NONE',  ( 10.48820292689142519, 16.37797505638186735, -17.32811247259324716 ) ) ;
#25469=CARTESIAN_POINT ( 'NONE',  ( 9.661894807476521407, 16.25477276558749296, -17.91386948909976695 ) ) ;
#25470=CARTESIAN_POINT ( 'NONE',  ( 20.53830075755067952, -2.223150928429542095, -18.95983797452030828 ) ) ;
#25471=CARTESIAN_POINT ( 'NONE',  ( 24.26229878782818261, 2.002655289519151172, -16.31248287692968546 ) ) ;
#25473=CARTESIAN_POINT ( 'NONE',  ( 18.63710449947919301, 3.826706299981984305, -14.11708861520305192 ) ) ;
#25478=CARTESIAN_POINT ( 'NONE',  ( 28.09718568327657806, -5.958257988085632562, -17.17874431236187149 ) ) ;
#25497=CARTESIAN_POINT ( 'NONE',  ( 19.20291185354690811, 8.143073066566493878, -16.32372945079811188 ) ) ;
#25498=CARTESIAN_POINT ( 'NONE',  ( 11.21766632152761822, 16.94531959984159641, -16.84123939818963223 ) ) ;
#25499=CARTESIAN_POINT ( 'NONE',  ( 33.44337896868773186, -12.72690026786775341, -19.72159258799634074 ) ) ;
#25502=CARTESIAN_POINT ( 'NONE',  ( 9.916336358462064737, 16.40777236560037622, -16.50459729666445696 ) ) ;
#25503=CARTESIAN_POINT ( 'NONE',  ( 9.641350810849047548, 17.66889113945805789, -17.98596209335946128 ) ) ;
#25509=CARTESIAN_POINT ( 'NONE',  ( 10.38089682401341385, 16.87009452252716102, -17.57504515238516873 ) ) ;
#25510=CARTESIAN_POINT ( 'NONE',  ( 34.38415957124060895, -12.46085888452578594, -19.93570721963346060 ) ) ;
#25511=CARTESIAN_POINT ( 'NONE',  ( 28.12266609392075267, -5.599633216697744942, -16.00068813756295327 ) ) ;
#25516=CARTESIAN_POINT ( 'NONE',  ( 13.80032290073870449, 8.087308377618120048, -14.09379472307618641 ) ) ;
#25517=CARTESIAN_POINT ( 'NONE',  ( 25.51035504519657593, -9.958856436819656821, -16.28203429854516315 ) ) ;
#25526=CARTESIAN_POINT ( 'NONE',  ( 10.33811697311952216, 18.38618935847563307, -17.91478972043705298 ) ) ;
#25530=CARTESIAN_POINT ( 'NONE',  ( 9.916411867603999397, 16.40742607105030260, -16.50456570466356965 ) ) ;
#25531=CARTESIAN_POINT ( 'NONE',  ( 16.02697758069565381, 6.204487712298734081, -15.55946274640501237 ) ) ;
#25534=CARTESIAN_POINT ( 'NONE',  ( 31.59793210864275537, -10.01186915388335485, -14.42687813506083039 ) ) ;
#25538=CARTESIAN_POINT ( 'NONE',  ( 11.34095285796786712, 16.37991182834946713, -16.75774407480071559 ) ) ;
#25540=CARTESIAN_POINT ( 'NONE',  ( 35.07504771885155037, -20.05712364337910714, -20.21480690768607857 ) ) ;
#25543=CARTESIAN_POINT ( 'NONE',  ( 24.92984004655564334, -8.306894832562658593, -19.61321747044761921 ) ) ;
#25547=CARTESIAN_POINT ( 'NONE',  ( 20.05507840940144959, 2.642024363331392234, -19.51255487852252912 ) ) ;
#25548=CARTESIAN_POINT ( 'NONE',  ( 26.63012090756776828, -10.30360588212082007, -13.56444477573641905 ) ) ;
#25555=CARTESIAN_POINT ( 'NONE',  ( 9.905109554012803130, 16.45925992188944420, -16.51025697316969953 ) ) ;
#25556=CARTESIAN_POINT ( 'NONE',  ( 26.07721637849146390, 0.4197350235787081774, -17.11807909718082144 ) ) ;
#25557=CARTESIAN_POINT ( 'NONE',  ( 22.42023978564754927, -3.655767601918122445, -13.54521809681785172 ) ) ;
#25558=CARTESIAN_POINT ( 'NONE',  ( 33.10306327339915811, -12.22190834454405106, -20.64716665866461298 ) ) ;
#25564=CARTESIAN_POINT ( 'NONE',  ( 15.54217852991911997, 3.796156774867226247, -18.16774540469225485 ) ) ;
#25567=CARTESIAN_POINT ( 'NONE',  ( 10.33811693838771717, 18.38618951776012267, -17.92981046679734547 ) ) ;
#25571=CARTESIAN_POINT ( 'NONE',  ( 16.06572049258021195, 3.735912457719189117, -15.00855390560170477 ) ) ;
#25573=CARTESIAN_POINT ( 'NONE',  ( 35.28941737075538043, -22.02017293461823755, -20.69856730472309891 ) ) ;
#25577=CARTESIAN_POINT ( 'NONE',  ( 23.98539618923253514, -1.204509296099786297, -17.73462021633622143 ) ) ;
#25579=CARTESIAN_POINT ( 'NONE',  ( 14.86918570794847305, 4.945381287188965302, -16.48322999939953704 ) ) ;
#25581=CARTESIAN_POINT ( 'NONE',  ( 20.85427418779519826, -0.3072727129311651484, -13.36207100503020584 ) ) ;
#25590=CARTESIAN_POINT ( 'NONE',  ( 36.14373538984320078, -19.36570096427324827, -19.42526322947885475 ) ) ;
#25591=CARTESIAN_POINT ( 'NONE',  ( 9.641350810849047548, 17.66889113945805789, -17.94384837343789485 ) ) ;
#25595=CARTESIAN_POINT ( 'NONE',  ( 10.44197622278032611, 16.58997661396885803, -17.36392598754248695 ) ) ;
#25605=CARTESIAN_POINT ( 'NONE',  ( 9.665905706931651409, 16.23637826941602569, -17.88729680195882565 ) ) ;
#25608=CARTESIAN_POINT ( 'NONE',  ( 23.43490106394649430, 0.5024168867186777909, -19.39616715318824802 ) ) ;
#25609=CARTESIAN_POINT ( 'NONE',  ( 23.01595892079019379, -1.674233493421072305, -13.97569732891719241 ) ) ;
#25613=CARTESIAN_POINT ( 'NONE',  ( 20.07445496384854877, 6.874260549971754841, -18.87959640166664954 ) ) ;
#25620=CARTESIAN_POINT ( 'NONE',  ( 26.85315702054868936, -3.432285194908070380, -17.01323758698984889 ) ) ;
#25630=CARTESIAN_POINT ( 'NONE',  ( 10.35864919664826900, 16.97212497753646687, -17.91558149794984445 ) ) ;
#25632=CARTESIAN_POINT ( 'NONE',  ( 33.38708106686501509, -12.47399286361455850, -19.70456970583452616 ) ) ;
#25635=CARTESIAN_POINT ( 'NONE',  ( 11.22408442728515077, 9.090372555205103566, -17.24152585048573982 ) ) ;
#25638=CARTESIAN_POINT ( 'NONE',  ( 20.52488529563827058, 3.974637744936419637, -19.97762432673833288 ) ) ;
#25639=CARTESIAN_POINT ( 'NONE',  ( 11.27588265011317326, 16.67833209609329259, -16.78465339804365541 ) ) ;
#25643=CARTESIAN_POINT ( 'NONE',  ( 9.915248083523094280, 16.41276333319327918, -16.50506225043874409 ) ) ;
#25646=CARTESIAN_POINT ( 'NONE',  ( 9.916775705961365261, 16.40575746196480011, -16.50441451066904364 ) ) ;
#25652=CARTESIAN_POINT ( 'NONE',  ( 10.50441255335269020, 16.30363564318377811, -17.32140922184415288 ) ) ;
#25655=CARTESIAN_POINT ( 'NONE',  ( 36.48591233058812833, -21.90292070287360460, -19.44112467175505898 ) ) ;
#25656=CARTESIAN_POINT ( 'NONE',  ( 24.14317479683219858, -6.286850201977149055, -18.60698471650063723 ) ) ;
#25666=CARTESIAN_POINT ( 'NONE',  ( 18.18682981270212196, 6.389142113859191952, -14.72334701657588063 ) ) ;
#25667=CARTESIAN_POINT ( 'NONE',  ( 29.41685937463160272, -8.713933360145817986, -16.19581194183416883 ) ) ;
#25678=CARTESIAN_POINT ( 'NONE',  ( 10.72061166913284325, 16.63201992582523658, -15.95427402900266856 ) ) ;
#25684=CARTESIAN_POINT ( 'NONE',  ( 11.47288049726737214, 9.269262779257836371, -15.86091052746238184 ) ) ;
#25686=CARTESIAN_POINT ( 'NONE',  ( 15.10317701704014226, 5.923596928851710075, -17.67988701311836053 ) ) ;
#25689=CARTESIAN_POINT ( 'NONE',  ( 27.89048517759004753, -11.43816616845083445, -12.79876095355805177 ) ) ;
#25692=CARTESIAN_POINT ( 'NONE',  ( 11.27636807789780171, 16.67610586239533177, -16.78445215232725118 ) ) ;
#25693=CARTESIAN_POINT ( 'NONE',  ( 35.26536834604049631, -19.91213340569504808, -19.23001471935974038 ) ) ;
#25699=CARTESIAN_POINT ( 'NONE',  ( 23.53678897557974281, -9.624609092408482169, -17.82855203159936863 ) ) ;
#25706=CARTESIAN_POINT ( 'NONE',  ( 22.98323032518889519, 2.094654362561221284, -17.51695658672324640 ) ) ;
#25708=CARTESIAN_POINT ( 'NONE',  ( 16.16754939756797782, 8.873905313537072459, -14.69432754670026142 ) ) ;
#25719=CARTESIAN_POINT ( 'NONE',  ( 9.642214727206800617, 17.66492910891761525, -17.80644250212319690 ) ) ;
#25720=CARTESIAN_POINT ( 'NONE',  ( 23.72497280669020014, -7.722717790116627512, -18.49470058199314693 ) ) ;
#25721=CARTESIAN_POINT ( 'NONE',  ( 23.07678757892180244, -0.1267571646896241688, -14.23703129728563965 ) ) ;
#25723=CARTESIAN_POINT ( 'NONE',  ( 32.11502935538656800, -10.34531343835429062, -18.85863636141847621 ) ) ;
#25726=CARTESIAN_POINT ( 'NONE',  ( 12.56861602585598980, 8.601024833420110483, -15.07548682890769243 ) ) ;
#25729=CARTESIAN_POINT ( 'NONE',  ( 17.63704213852533442, 9.806822523219006271, -18.50018230520716145 ) ) ;
#25732=CARTESIAN_POINT ( 'NONE',  ( 10.33811811146757265, 18.38618413786636552, -17.91101973220562371 ) ) ;
#25736=CARTESIAN_POINT ( 'NONE',  ( 17.21692058948253035, 4.245457944912791604, -14.13226496128363863 ) ) ;
#25737=CARTESIAN_POINT ( 'NONE',  ( 13.18850634723077242, 6.203946520731500769, -19.20132247218941401 ) ) ;
#25740=CARTESIAN_POINT ( 'NONE',  ( 33.13932541451587355, -12.36573032794433047, -20.66922553108291538 ) ) ;
#25741=CARTESIAN_POINT ( 'NONE',  ( 20.63450008290067927, -1.653576198284400833, -18.07233451455898532 ) ) ;
#25742=CARTESIAN_POINT ( 'NONE',  ( 20.64697163712990857, 4.580154932681155699, -17.29389188279686707 ) ) ;
#25745=CARTESIAN_POINT ( 'NONE',  ( 28.34689840388910653, -5.967659833748593101, -13.48819167749268644 ) ) ;
#25755=CARTESIAN_POINT ( 'NONE',  ( 36.27242973171742335, -19.94385647102418702, -19.46417027601260230 ) ) ;
#25756=CARTESIAN_POINT ( 'NONE',  ( 9.641350810849047548, 17.66889113945805789, -21.33333333332589277 ) ) ;
#25762=CARTESIAN_POINT ( 'NONE',  ( 10.47249985125707106, 16.44999136291752251, -17.33460624675630513 ) ) ;
#25773=CARTESIAN_POINT ( 'NONE',  ( 9.662070302079424522, 16.25396792496884046, -17.90822120357413638 ) ) ;
#25776=CARTESIAN_POINT ( 'NONE',  ( 23.95332181684718975, -6.025008234661991757, -14.41687206698971124 ) ) ;
#25777=CARTESIAN_POINT ( 'NONE',  ( 20.41927524488895429, 4.553956414902842198, -14.69105443414393264 ) ) ;
#25781=CARTESIAN_POINT ( 'NONE',  ( 24.18219217278060995, -6.970120066757704791, -14.18070892486464629 ) ) ;
#25790=CARTESIAN_POINT ( 'NONE',  ( 10.47184394332236224, 16.45299944031493311, -17.33487789703667303 ) ) ;
#25793=CARTESIAN_POINT ( 'NONE',  ( 33.10952763335142635, -11.62914684427059697, -19.38687730282833499 ) ) ;
#25795=CARTESIAN_POINT ( 'NONE',  ( 8.944584683310379702, 16.95159276115599667, -21.33333333332589632 ) ) ;
#25799=CARTESIAN_POINT ( 'NONE',  ( 20.72626264887238534, -1.914771856900582714, -13.62749948506543518 ) ) ;
#25800=CARTESIAN_POINT ( 'NONE',  ( 11.26867954870061439, 16.71136643735313143, -16.78814161468471156 ) ) ;
#25804=CARTESIAN_POINT ( 'NONE',  ( 9.641350944112486943, 17.66889052829492002, -17.91441860517739215 ) ) ;
#25806=CARTESIAN_POINT ( 'NONE',  ( 11.34314632229486364, 9.864239995495806212, -15.91456019135469013 ) ) ;
#25812=CARTESIAN_POINT ( 'NONE',  ( 10.79618582965528439, 14.96552620561766567, -17.20075070836251996 ) ) ;
#25815=CARTESIAN_POINT ( 'NONE',  ( 36.07559364978101968, -20.05957622185551870, -20.44697815928661200 ) ) ;
#25816=CARTESIAN_POINT ( 'NONE',  ( 14.78952226657687063, 10.37904477376192069, -15.12939866669752575 ) ) ;
#25817=CARTESIAN_POINT ( 'NONE',  ( 27.95388715220626707, -5.541385876428546631, -15.41148221666858831 ) ) ;
#25820=( GEOMETRIC_REPRESENTATION_CONTEXT ( 3 ) GLOBAL_UNCERTAINTY_ASSIGNED_CONTEXT ( ( #7366 ) ) GLOBAL_UNIT_ASSIGNED_CONTEXT ( ( #25150, #22715, #1516 ) ) REPRESENTATION_CONTEXT ( 'NONE', 'WORKASPACE' ) );
#25823=CARTESIAN_POINT ( 'NONE',  ( 17.40794641162625567, 9.636182090832996039, -14.27881468665684395 ) ) ;
#25824=CARTESIAN_POINT ( 'NONE',  ( 14.03850921439652311, 8.975161913830900673, -15.18271992443145635 ) ) ;
#25837=CARTESIAN_POINT ( 'NONE',  ( 10.71880336532874445, 16.64031303757595026, -15.95504377300109944 ) ) ;
#25844=CARTESIAN_POINT ( 'NONE',  ( 10.95411528722473626, 11.64838591225006859, -16.07543820933196699 ) ) ;
#25846=CARTESIAN_POINT ( 'NONE',  ( 9.665905706931651409, 16.23637826941602569, -17.88729680195882565 ) ) ;
#25847=CARTESIAN_POINT ( 'NONE',  ( 16.58324305800299925, 4.586402732284541095, -18.38077023430394163 ) ) ;
#25850=CARTESIAN_POINT ( 'NONE',  ( 27.91615220763155847, -6.225400021157185826, -17.67258836524805332 ) ) ;
#25853=CARTESIAN_POINT ( 'NONE',  ( 11.05542208158282769, 17.68939236555957706, -17.90700183802944778 ) ) ;
#25855=CARTESIAN_POINT ( 'NONE',  ( 34.76605987604303749, -17.66900494105776787, -19.07908574721388462 ) ) ;
#25859=CARTESIAN_POINT ( 'NONE',  ( 23.66316133457650750, -10.02594615916883392, -14.11990577516520595 ) ) ;
#25863=CARTESIAN_POINT ( 'NONE',  ( 16.05281274719596496, 2.901206577426825639, -17.92093306952238407 ) ) ;
#25864=CARTESIAN_POINT ( 'NONE',  ( 16.85369750842388825, 4.841181898090542113, -18.70119709635011418 ) ) ;
#25876=CARTESIAN_POINT ( 'NONE',  ( 9.914377700407460026, 16.41675502110963336, -16.50544604630902867 ) ) ;
#25878=CARTESIAN_POINT ( 'NONE',  ( 22.63726333831294468, -4.877931240889711972, -12.86144741616201870 ) ) ;
#25879=CARTESIAN_POINT ( 'NONE',  ( 22.47820520476076567, 2.340993144345510313, -15.49451772223075707 ) ) ;
#25880=CARTESIAN_POINT ( 'NONE',  ( 33.31547190024930671, -13.15228156363260581, -20.72525089784059560 ) ) ;
#25884=CARTESIAN_POINT ( 'NONE',  ( 12.51417009928267099, 8.576964204390579383, -15.11888119342340353 ) ) ;
#25887=CARTESIAN_POINT ( 'NONE',  ( 19.11618317516819587, 7.271703427217982352, -19.10559232466456692 ) ) ;
#25889=CARTESIAN_POINT ( 'NONE',  ( 10.72183334705107960, 16.62641715516447150, -15.95376865854981929 ) ) ;
#25894=CARTESIAN_POINT ( 'NONE',  ( 16.89609864265585060, 4.102175112930991574, -14.31125941877678720 ) ) ;
#25896=CARTESIAN_POINT ( 'NONE',  ( 13.03988341252192917, 6.056598437983586436, -18.79510648546616736 ) ) ;
#25898=CARTESIAN_POINT ( 'NONE',  ( 32.62126879184269512, -11.04717877266006987, -18.30218954475424908 ) ) ;
#25900=CARTESIAN_POINT ( 'NONE',  ( 23.56326861202678202, -1.685860805813322427, -18.23406631578895798 ) ) ;
#25902=CARTESIAN_POINT ( 'NONE',  ( 18.96452888794134495, 2.710274068595869057, -18.82741851907772457 ) ) ;
#25903=CARTESIAN_POINT ( 'NONE',  ( 28.79879967665997142, -10.96283228269853893, -18.01937015232834938 ) ) ;
#25913=CARTESIAN_POINT ( 'NONE',  ( 36.36958547251401797, -20.38032574959806098, -19.43068663056894252 ) ) ;
#25915=CARTESIAN_POINT ( 'NONE',  ( 9.641351338355821810, 17.66888872024471624, -17.91303689663363130 ) ) ;
#25919=CARTESIAN_POINT ( 'NONE',  ( 12.07790154976966868, 9.144051220271959934, -16.66639656463015839 ) ) ;
#25928=CARTESIAN_POINT ( 'NONE',  ( 9.668002105539015290, 16.22676391817335784, -17.88502066855795292 ) ) ;
#25929=CARTESIAN_POINT ( 'NONE',  ( 27.39421632154990505, -5.413734532252513887, -17.93514013592066902 ) ) ;
#25930=CARTESIAN_POINT ( 'NONE',  ( 20.31878617967674217, -0.6648838724932636390, -18.90140657046049455 ) ) ;
#25935=CARTESIAN_POINT ( 'NONE',  ( 25.77659985377941254, -6.250509680199615836, -13.67467641272277312 ) ) ;
#25941=CARTESIAN_POINT ( 'NONE',  ( 10.53683180627515981, 16.15495681678771689, -17.30800272034635867 ) ) ;
#25943=CARTESIAN_POINT ( 'NONE',  ( 33.48796008207983022, -12.92717959506727965, -19.73506838908087246 ) ) ;
#25945=CARTESIAN_POINT ( 'NONE',  ( 8.944585970659694851, 16.95158685720792846, -17.91243444582771005 ) ) ;
#25949=CARTESIAN_POINT ( 'NONE',  ( 17.33713706444265412, 0.9871066061555996418, -18.79342181739402307 ) ) ;
#25950=CARTESIAN_POINT ( 'NONE',  ( 11.31663841827600692, 16.49142094814642334, -16.76779895092377615 ) ) ;
#25955=CARTESIAN_POINT ( 'NONE',  ( 9.641350810849047548, 17.66889113945805789, -17.91928203681695564 ) ) ;
#25957=CARTESIAN_POINT ( 'NONE',  ( 9.695397291186985456, 17.42102709130404747, -17.08803885907851594 ) ) ;
#25959=ORIENTED_EDGE ( 'NONE', *, *, #10730, .F. ) ;
#25962=CARTESIAN_POINT ( 'NONE',  ( 10.35866308580767026, 16.97206128008099313, -17.90676409391864610 ) ) ;
#25964=CARTESIAN_POINT ( 'NONE',  ( 31.49515780845362301, -9.451207104696591088, -14.88922074032172205 ) ) ;
#25965=CARTESIAN_POINT ( 'NONE',  ( 26.08768104250457753, -11.87935956797728210, -17.28510650846989805 ) ) ;
#25966=CARTESIAN_POINT ( 'NONE',  ( 15.23264752967198099, 8.612683518626374379, -20.21708921969009154 ) ) ;
#25971=CARTESIAN_POINT ( 'NONE',  ( 32.83462640711407232, -10.30445905196369516, -16.67331141712644538 ) ) ;
#25975=CARTESIAN_POINT ( 'NONE',  ( 17.75014749421169213, 9.747325538739326944, -14.55496937630740639 ) ) ;
#25977=CARTESIAN_POINT ( 'NONE',  ( 17.17204249742301059, 10.23148044644768362, -15.96021614775051667 ) ) ;
#25988=CARTESIAN_POINT ( 'NONE',  ( 10.35722669462089840, 18.29854973974792998, -17.31575102165233915 ) ) ;
#25993=CARTESIAN_POINT ( 'NONE',  ( 9.981537699549546616, 16.10875070413535681, -16.47763325427154868 ) ) ;
#25995=CARTESIAN_POINT ( 'NONE',  ( 9.669138625804738041, 16.22155169136211583, -17.88455067742322413 ) ) ;
#25997=CARTESIAN_POINT ( 'NONE',  ( 20.09928279393940898, 2.810699353624661168, -13.58730878818371401 ) ) ;
#26000=CARTESIAN_POINT ( 'NONE',  ( 29.22485947447185595, -8.910266539455653501, -18.36689805200119707 ) ) ;
#26003=CARTESIAN_POINT ( 'NONE',  ( 11.27146506517978786, 16.69859170370891377, -16.78668372539920739 ) ) ;
#26005=CARTESIAN_POINT ( 'NONE',  ( 33.40448403937627830, -11.94904316976568914, -18.43672998654903239 ) ) ;
#26009=CARTESIAN_POINT ( 'NONE',  ( 9.111869836743295537, 16.18440172361536611, -17.05500387803421702 ) ) ;
#26010=CARTESIAN_POINT ( 'NONE',  ( 22.59934115267691368, -6.304331921927718518, -14.46034029096162143 ) ) ;
#26016=CARTESIAN_POINT ( 'NONE',  ( 16.03657434348277633, 2.746931742562784162, -16.83325620853174698 ) ) ;
#26017=CARTESIAN_POINT ( 'NONE',  ( 18.33619432801213023, 6.228962682262685568, -18.83744168170139233 ) ) ;
#26030=CARTESIAN_POINT ( 'NONE',  ( 9.826288910175632552, 16.82074144182198694, -16.60662094963572244 ) ) ;
#26031=CARTESIAN_POINT ( 'NONE',  ( 26.06970682676011464, -9.363093171025507644, -17.79562309782675911 ) ) ;
#26032=CARTESIAN_POINT ( 'NONE',  ( 20.29352232415978463, 1.537418251635638944, -14.27211978419980021 ) ) ;
#26033=CARTESIAN_POINT ( 'NONE',  ( 33.24414211882076842, -12.83183464011245967, -20.70368961610576264 ) ) ;
#26036=CARTESIAN_POINT ( 'NONE',  ( 12.50396148805030627, 8.572452836447732594, -15.12701763676990119 ) ) ;
#26041=CARTESIAN_POINT ( 'NONE',  ( 10.72335299953182286, 16.61944783517715862, -15.95314022879208693 ) ) ;
#26044=CARTESIAN_POINT ( 'NONE',  ( 16.21960234321935701, 7.070186740785398882, -14.59618053200276044 ) ) ;
#26046=CARTESIAN_POINT ( 'NONE',  ( 18.20609423209794642, 11.47008825724650549, -18.02705416172272734 ) ) ;
#26048=CARTESIAN_POINT ( 'NONE',  ( 33.43446274600908907, -12.68684440242773448, -19.71889742777951327 ) ) ;
#26049=CARTESIAN_POINT ( 'NONE',  ( 22.08234585817149664, -3.071498426668943793, -18.09723855971599704 ) ) ;
#26051=CARTESIAN_POINT ( 'NONE',  ( 18.46387099684246635, 2.251061286204190992, -18.51322769290417369 ) ) ;
#26055=CARTESIAN_POINT ( 'NONE',  ( 27.61097550864939265, -12.05054904645494673, -17.30446993171443637 ) ) ;
#26066=CARTESIAN_POINT ( 'NONE',  ( 36.54859390953724585, -21.18451583373416014, -16.94733705004010105 ) ) ;
#26067=CARTESIAN_POINT ( 'NONE',  ( 12.75768479220908169, 7.626547943635540783, -14.92479568483475028 ) ) ;
#26072=CARTESIAN_POINT ( 'NONE',  ( 12.02780084644370007, 9.317182744227245905, -16.69143457430396893 ) ) ;
#26075=ORIENTED_EDGE ( 'NONE', *, *, #6052, .F. ) ;
#26081=CARTESIAN_POINT ( 'NONE',  ( 13.37514969516658070, 7.623989538026159529, -15.71142857098959489 ) ) ;
#26082=CARTESIAN_POINT ( 'NONE',  ( 27.64917536653120678, -4.837437286474155052, -16.54522848743341967 ) ) ;
#26084=CARTESIAN_POINT ( 'NONE',  ( 22.75707610144304383, -3.504958924507949991, -13.40925247317622571 ) ) ;
#26097=CARTESIAN_POINT ( 'NONE',  ( 12.02710433905669341, 9.320377015888107408, -16.69172260460959478 ) ) ;
#26099=CARTESIAN_POINT ( 'NONE',  ( 33.54145741815126058, -13.16751478770765793, -19.75123935038191192 ) ) ;
#26101=CARTESIAN_POINT ( 'NONE',  ( 13.38095672321806795, 7.626547943635540783, -15.70680086385617358 ) ) ;
#26104=CARTESIAN_POINT ( 'NONE',  ( 21.64656857049893901, 5.639188926465734220, -17.17864421186117951 ) ) ;
#26105=CARTESIAN_POINT ( 'NONE',  ( 12.83231907764629476, 9.540323555994485005, -16.14101112307237074 ) ) ;
#26111=CARTESIAN_POINT ( 'NONE',  ( 11.50832337395308436, 9.139936167900076569, -15.84372008594036885 ) ) ;
#26113=CARTESIAN_POINT ( 'NONE',  ( 9.924804006935172396, 16.36893865032855899, -16.50109463189289016 ) ) ;
#26118=CARTESIAN_POINT ( 'NONE',  ( 10.47604570704546845, 16.43372961628045559, -17.33313991065496751 ) ) ;
#26121=CARTESIAN_POINT ( 'NONE',  ( 32.21775685856648153, -9.560954865089090760, -16.93152350858319366 ) ) ;
#26122=CARTESIAN_POINT ( 'NONE',  ( 28.01381056668970260, -10.10121741814351459, -18.82353034625045041 ) ) ;
#26123=CARTESIAN_POINT ( 'NONE',  ( 16.30094628073386076, 10.97451324635404291, -15.74372407192620216 ) ) ;
#26128=CARTESIAN_POINT ( 'NONE',  ( 33.97319001242765779, -11.13623552147873141, -19.50814438409551954 ) ) ;
#26130=CARTESIAN_POINT ( 'NONE',  ( 18.67986154365276619, -0.9315889389632653339, -17.94220784458306994 ) ) ;
#26132=CARTESIAN_POINT ( 'NONE',  ( 26.86129341093661793, -9.458291044957649163, -14.14057404834478682 ) ) ;
#26140=CARTESIAN_POINT ( 'NONE',  ( 12.27341590537944249, 9.504120828508773045, -15.31263355901650947 ) ) ;
#26146=CARTESIAN_POINT ( 'NONE',  ( 11.97192087863669663, 8.579774655713777065, -15.53257280409644991 ) ) ;
#26150=CARTESIAN_POINT ( 'NONE',  ( 16.42253358145367415, 4.166353156564198024, -16.06924993952044289 ) ) ;
#26157=CARTESIAN_POINT ( 'NONE',  ( 11.16343636398553052, 17.19402509784177369, -16.95964061678045454 ) ) ;
#26159=CARTESIAN_POINT ( 'NONE',  ( 33.23735339574943026, -11.79161913663336314, -18.04114522998021997 ) ) ;
#26160=CARTESIAN_POINT ( 'NONE',  ( 20.23291344124205793, 5.521974472852556381, -14.51730806008046137 ) ) ;
#26162=CARTESIAN_POINT ( 'NONE',  ( 10.14999423553203606, 11.42343090068832190, -16.62569685487721571 ) ) ;
#26163=CARTESIAN_POINT ( 'NONE',  ( 24.76964776845370864, -3.801875552749832909, -18.97459646659829247 ) ) ;
#26167=CARTESIAN_POINT ( 'NONE',  ( 20.73027244251523626, 3.305903845835247434, -19.25852547563239625 ) ) ;
#26168=CARTESIAN_POINT ( 'NONE',  ( 17.81918496738754953, 9.416330548141603529, -16.00206777915198586 ) ) ;
#26179=CARTESIAN_POINT ( 'NONE',  ( 9.641384570184822422, 17.66873631484086715, -17.89388817125738385 ) ) ;
#26180=CARTESIAN_POINT ( 'NONE',  ( 26.67280208910032258, -8.806626608708889137, -18.22016464309510653 ) ) ;
#26181=CARTESIAN_POINT ( 'NONE',  ( 24.00718893345771932, -1.002666751694005765, -18.91818096615087796 ) ) ;
#26183=CARTESIAN_POINT ( 'NONE',  ( 35.54859390953724585, -23.18451583373416014, -18.19919658220850422 ) ) ;
#26186=CARTESIAN_POINT ( 'NONE',  ( 12.55500454421123457, 8.595009676161804890, -15.08633542003848049 ) ) ;
#26192=CARTESIAN_POINT ( 'NONE',  ( 19.91209246711783010, 5.411768277715644615, -14.29674560697521457 ) ) ;
#26195=CARTESIAN_POINT ( 'NONE',  ( 10.61946839964472034, 17.09587585246520902, -16.05247762654136068 ) ) ;
#26199=CARTESIAN_POINT ( 'NONE',  ( 17.36512755686010934, 0.5347363583120325892, -15.24149349723765390 ) ) ;
#26200=CARTESIAN_POINT ( 'NONE',  ( 16.80873327975549003, 11.45062080556171757, -15.01659013532395370 ) ) ;
#26202=CARTESIAN_POINT ( 'NONE',  ( 35.37764311538968087, -21.41652447078215005, -19.89511094362359955 ) ) ;
#26203=CARTESIAN_POINT ( 'NONE',  ( 23.48045015178454165, 1.263488895044508897, -17.26779756161726098 ) ) ;
#26204=CARTESIAN_POINT ( 'NONE',  ( 19.81827328964134338, 3.502454073897792952, -18.79004964864563476 ) ) ;
#26205=CARTESIAN_POINT ( 'NONE',  ( 26.70980024742295456, -9.230482666323300833, -19.13350686062700134 ) ) ;
#26215=CARTESIAN_POINT ( 'NONE',  ( 33.49783966318349115, -10.45910432307822902, -18.51641766868578287 ) ) ;
#26217=CARTESIAN_POINT ( 'NONE',  ( 9.641350810849047548, 17.66889113945805789, -17.97192418671891190 ) ) ;
#26223=CARTESIAN_POINT ( 'NONE',  ( 11.99569818778800645, 9.464409628959467469, -16.70471015293584216 ) ) ;
#26233=CARTESIAN_POINT ( 'NONE',  ( 11.29844335826449964, 8.819016302236921234, -17.20546268888528374 ) ) ;
#26235=CARTESIAN_POINT ( 'NONE',  ( 26.11288949521356528, -6.777652795969290267, -18.96966820991230662 ) ) ;
#26236=CARTESIAN_POINT ( 'NONE',  ( 19.50876870223950377, -1.661710298099399630, -15.95382585723518432 ) ) ;
#26247=CARTESIAN_POINT ( 'NONE',  ( 10.47175433613752027, 16.45341039028688002, -17.33491556667247835 ) ) ;
#26249=CARTESIAN_POINT ( 'NONE',  ( 31.63980255171021483, -10.89810845426378982, -15.52824638758754183 ) ) ;
#26252=CARTESIAN_POINT ( 'NONE',  ( 13.37763225631166542, 7.625080029534266224, -15.70945042905673006 ) ) ;
#26255=CARTESIAN_POINT ( 'NONE',  ( 19.12501085131992085, -2.578449613843157184, -15.80510918775627438 ) ) ;
#26257=CARTESIAN_POINT ( 'NONE',  ( 12.82970573826865390, 9.552301347437191836, -16.14209238882153130 ) ) ;
#26262=CARTESIAN_POINT ( 'NONE',  ( 11.14863080475985591, 10.75631295387255548, -15.99499920034263489 ) ) ;
#26265=CARTESIAN_POINT ( 'NONE',  ( 9.917205744531459644, 16.40378525026516243, -16.50423678068149869 ) ) ;
#26270=CARTESIAN_POINT ( 'NONE',  ( 11.99569818778800645, 9.464409628959467469, -16.70471015293584216 ) ) ;
#26272=CARTESIAN_POINT ( 'NONE',  ( 34.10649047503919462, -12.21345526111254287, -20.89408644300621987 ) ) ;
#26273=CARTESIAN_POINT ( 'NONE',  ( 15.95367323521391256, 9.281262803959288377, -20.14168370736028280 ) ) ;
#26274=CARTESIAN_POINT ( 'NONE',  ( 16.07247723200118372, 10.90037199175087324, -15.55898442674143745 ) ) ;
#26279=CARTESIAN_POINT ( 'NONE',  ( 19.60537025999656890, 4.505197036469223981, -15.34927506990110047 ) ) ;
#26281=CARTESIAN_POINT ( 'NONE',  ( 15.44629794785920218, 3.545610805586186132, -16.71614555938632307 ) ) ;
#26290=CARTESIAN_POINT ( 'NONE',  ( 12.26883957244698387, 9.531649408071682927, -15.31402716519172635 ) ) ;
#26296=CARTESIAN_POINT ( 'NONE',  ( 12.49428694376680049, 8.568214790255201052, -15.13472557389765072 ) ) ;
#26298=CARTESIAN_POINT ( 'NONE',  ( 16.67011857490315307, 4.279483903030143921, -15.63504347475558198 ) ) ;
#26305=CARTESIAN_POINT ( 'NONE',  ( 12.86106464449595777, 9.514195438118767001, -16.12106201145810047 ) ) ;
#26308=CARTESIAN_POINT ( 'NONE',  ( 34.62340031318386480, -17.02811109401968181, -19.03596318374462726 ) ) ;
#26309=CARTESIAN_POINT ( 'NONE',  ( 14.18486973814142793, 6.324582201221724098, -17.68508340245422872 ) ) ;
#26311=CARTESIAN_POINT ( 'NONE',  ( 26.29067154119281824, -12.76617647537077538, -18.64558906701574514 ) ) ;
#26315=CARTESIAN_POINT ( 'NONE',  ( 20.61437924707763258, -4.384239709691692966, -16.09784705243023240 ) ) ;
#26316=CARTESIAN_POINT ( 'NONE',  ( 16.31265859067239532, 4.319332383768222705, -17.78589364095596892 ) ) ;
#26330=CARTESIAN_POINT ( 'NONE',  ( 11.49350937636955372, 9.187954247928445284, -15.85136552863131421 ) ) ;
#26331=CARTESIAN_POINT ( 'NONE',  ( 29.11570147443254797, -8.594497869595446815, -15.09001435577217087 ) ) ;
#26332=CARTESIAN_POINT ( 'NONE',  ( 24.27430760268559595, -10.23567508289028716, -17.26834523416827949 ) ) ;
#26333=CARTESIAN_POINT ( 'NONE',  ( 34.70640263809442416, -19.40099657226499019, -21.14569589167440000 ) ) ;
#26341=CARTESIAN_POINT ( 'NONE',  ( 17.33713706444265412, 0.9871066061555996418, -18.79342181739402307 ) ) ;
#26345=CARTESIAN_POINT ( 'NONE',  ( 12.27009251048667160, 9.509012028593735621, -15.31479730457434307 ) ) ;
#26350=CARTESIAN_POINT ( 'NONE',  ( 22.89472691350227507, 1.279074496056108901, -19.72372301458170796 ) ) ;
#26351=CARTESIAN_POINT ( 'NONE',  ( 26.88742137321887427, -10.86886578961255978, -19.57440296808016100 ) ) ;
#26353=CARTESIAN_POINT ( 'NONE',  ( 35.54287943964028784, -22.15884374752674546, -18.65915260879160797 ) ) ;
#26355=CARTESIAN_POINT ( 'NONE',  ( 28.41550859958678643, -4.728095322062062067, -17.81194336819277524 ) ) ;
#26356=CARTESIAN_POINT ( 'NONE',  ( 20.29079399015155616, 4.720006093641750944, -15.95989367155712202 ) ) ;
#26371=CARTESIAN_POINT ( 'NONE',  ( 35.34711162051457478, -16.78689235204268115, -20.22678452305727603 ) ) ;
#26372=CARTESIAN_POINT ( 'NONE',  ( 10.17605321708455257, 15.21667774575863419, -16.39719424528293246 ) ) ;
#26375=CARTESIAN_POINT ( 'NONE',  ( 12.84373479294319864, 8.511860559062048637, -16.13004233893675377 ) ) ;
#26387=CARTESIAN_POINT ( 'NONE',  ( 11.22373969136065242, 9.091953032947756697, -17.24166845096988609 ) ) ;
#26389=CARTESIAN_POINT ( 'NONE',  ( 24.01770293978927384, -9.123702295727731837, -14.45939194930751448 ) ) ;
#26390=CARTESIAN_POINT ( 'NONE',  ( 20.97149233804390533, -0.06858483505933390956, -19.21322127741759189 ) ) ;
#26402=CARTESIAN_POINT ( 'NONE',  ( 10.73134732381016576, 15.26288385841099249, -17.22756371135774245 ) ) ;
#26403=CARTESIAN_POINT ( 'NONE',  ( 35.12509383387676820, -20.28195432802065312, -20.22992657050740917 ) ) ;
#26405=CARTESIAN_POINT ( 'NONE',  ( 13.37841584274036855, 7.625425322794393779, -15.70882597216490240 ) ) ;
#26406=CARTESIAN_POINT ( 'NONE',  ( 26.31132954256896639, -3.159408024760113509, -14.81636702655834803 ) ) ;
#26407=CARTESIAN_POINT ( 'NONE',  ( 12.86479781618563045, 9.514843269526567227, -16.11816302316177030 ) ) ;
#26412=CARTESIAN_POINT ( 'NONE',  ( 11.47079713067724782, 9.278817116560638567, -15.86177209170659275 ) ) ;
#26414=CARTESIAN_POINT ( 'NONE',  ( 12.39803340617553928, 8.535179507765855433, -15.21071672276548625 ) ) ;
#26419=CARTESIAN_POINT ( 'NONE',  ( 12.02786405831828986, 9.316892843345049968, -16.69140843421181231 ) ) ;
#26421=CARTESIAN_POINT ( 'NONE',  ( 30.78206665311622459, -10.11802168058175511, -15.10569088962643036 ) ) ;
#26422=CARTESIAN_POINT ( 'NONE',  ( 27.89048517759004753, -11.43816616845083445, -12.79876095355805177 ) ) ;
#26423=CARTESIAN_POINT ( 'NONE',  ( 16.78426473046523526, 10.16049046829612479, -19.50779498702920378 ) ) ;
#26430=CARTESIAN_POINT ( 'NONE',  ( 22.11273855634006935, 3.201273238686522138, -15.95510540678940181 ) ) ;
#26431=CARTESIAN_POINT ( 'NONE',  ( 15.41431293496917121, 3.575304669039410133, -17.09800041271234150 ) ) ;
#26443=CARTESIAN_POINT ( 'NONE',  ( 12.01759036229752553, 10.68391031264169122, -15.41792755180196473 ) ) ;
#26447=CARTESIAN_POINT ( 'NONE',  ( 11.48890098693651396, 9.204103201752445784, -15.85365151319587440 ) ) ;
#26450=CARTESIAN_POINT ( 'NONE',  ( 16.24840684054896656, 4.149509756678782857, -16.79736725456322688 ) ) ;
#26458=CARTESIAN_POINT ( 'NONE',  ( 12.83227841057820484, 9.540504573332061256, -16.14102835882348330 ) ) ;
#26460=CARTESIAN_POINT ( 'NONE',  ( 36.51492826578181194, -21.03327392953103825, -18.93061234292109063 ) ) ;
#26461=CARTESIAN_POINT ( 'NONE',  ( 16.79143122783437292, 7.330551994622505063, -14.54187356113185103 ) ) ;
#26466=CARTESIAN_POINT ( 'NONE',  ( 18.00441060066494003, 9.543425513107552050, -19.87907960298149490 ) ) ;
#26470=CARTESIAN_POINT ( 'NONE',  ( 26.86433939054618492, -2.362129714094441724, -16.96571632802953644 ) ) ;
#26471=CARTESIAN_POINT ( 'NONE',  ( 18.18253756980838531, -1.899343836538245789, -17.94647550410194370 ) ) ;
#26477=APPLICATION_CONTEXT ( 'automotive_design' ) ;
#26483=CARTESIAN_POINT ( 'NONE',  ( 11.65548303173490652, 8.849831895876286936, -15.75351705932409985 ) ) ;
#26484=CARTESIAN_POINT ( 'NONE',  ( 25.51035504519657593, -9.958856436819656821, -16.28203429854516315 ) ) ;
#26485=CARTESIAN_POINT ( 'NONE',  ( 26.20148740379470453, -2.166401353139026487, -14.75472287570676322 ) ) ;
#26486=CARTESIAN_POINT ( 'NONE',  ( 31.63980255171021483, -10.89810845426378982, -15.52824638758754183 ) ) ;
#26494=CARTESIAN_POINT ( 'NONE',  ( 23.66601916330066402, 2.199037240492611733, -18.57254039386976885 ) ) ;
#26497=CARTESIAN_POINT ( 'NONE',  ( 12.26681336913932974, 9.540941834721429871, -15.31486507153535648 ) ) ;
#26499=DIRECTION ( 'NONE',  ( 0.000000000000000000, 0.000000000000000000, -1.000000000000000000 ) ) ;
#26501=CARTESIAN_POINT ( 'NONE',  ( 25.31619048431776875, -0.2099727537683927225, -15.56338435260822628 ) ) ;
#26502=CARTESIAN_POINT ( 'NONE',  ( 17.45108151888110726, 3.014897074772306507, -13.47014999590450479 ) ) ;
#26504=CARTESIAN_POINT ( 'NONE',  ( 34.75406370242679799, -18.61511248754081294, -20.11778113987843852 ) ) ;
#26506=CARTESIAN_POINT ( 'NONE',  ( 26.73315660230872837, -4.509142541826837380, -13.49646658189591619 ) ) ;
#26507=CARTESIAN_POINT ( 'NONE',  ( 24.91205307904067112, 1.131441846345163427, -15.76301496618838627 ) ) ;
#26510=CARTESIAN_POINT ( 'NONE',  ( 23.22413189157496305, -7.367447486509826504, -15.63851824576001981 ) ) ;
#26518=CARTESIAN_POINT ( 'NONE',  ( 18.47844294452917424, 10.16049799425131361, -18.92511192449534718 ) ) ;
#26519=CARTESIAN_POINT ( 'NONE',  ( 35.88208498122789791, -19.19024427843809733, -20.38849413606966010 ) ) ;
#26520=CARTESIAN_POINT ( 'NONE',  ( 9.926830210242822972, 16.35964622367879784, -16.50025672554925293 ) ) ;
#26524=CARTESIAN_POINT ( 'NONE',  ( 12.00785540763395254, 9.408655069060824161, -16.69968271487400813 ) ) ;
#26537=CARTESIAN_POINT ( 'NONE',  ( 11.86544027865023843, 7.919735734555668039, -16.84125344233394372 ) ) ;
#26539=CARTESIAN_POINT ( 'NONE',  ( 25.72097854023329688, -11.95459465090917917, -18.51508836554082293 ) ) ;
#26540=CARTESIAN_POINT ( 'NONE',  ( 19.39248696316839116, -1.610358169686434193, -16.91126230894791860 ) ) ;
#26552=CARTESIAN_POINT ( 'NONE',  ( 12.06596557120094992, 9.177570865404522493, -16.67295095431955332 ) ) ;
#26553=CARTESIAN_POINT ( 'NONE',  ( 35.54859390953723874, -22.18451583373416014, -15.00000000000000000 ) ) ;
#26555=CARTESIAN_POINT ( 'NONE',  ( 9.109746387114286748, 16.19414013429083710, -17.05597298747021640 ) ) ;
#26556=CARTESIAN_POINT ( 'NONE',  ( 25.77659985377941254, -6.250509680199615836, -13.67467641272277312 ) ) ;
#26557=CARTESIAN_POINT ( 'NONE',  ( 12.83236877538120524, 9.540106609504201529, -16.14098973436422568 ) ) ;
#26565=CARTESIAN_POINT ( 'NONE',  ( 11.50832337395308436, 9.139936167900076569, -15.84372008594036885 ) ) ;
#26571=CARTESIAN_POINT ( 'NONE',  ( 12.72883512080982804, 8.524354266104470668, -16.21679389071614352 ) ) ;
#26573=CARTESIAN_POINT ( 'NONE',  ( 19.13824544459052035, 4.841912194177635520, -12.94453987625427160 ) ) ;
#26574=CARTESIAN_POINT ( 'NONE',  ( 27.89048517759004753, -11.43816616845083445, -12.79876095355805177 ) ) ;
#26578=CARTESIAN_POINT ( 'NONE',  ( 36.54859390953724585, -22.18451583373416014, -17.22552805718784441 ) ) ;
#26581=CARTESIAN_POINT ( 'NONE',  ( 19.42159491456138554, 2.195880709831018684, -14.63272625841335106 ) ) ;
#26582=CARTESIAN_POINT ( 'NONE',  ( 15.87806330829146617, 7.947701475055697351, -19.83831759000646855 ) ) ;
#26588=CARTESIAN_POINT ( 'NONE',  ( 13.77718166750865869, 8.859676595473324312, -15.39100258941132182 ) ) ;
#26590=CARTESIAN_POINT ( 'NONE',  ( 12.27644674946102832, 9.496504630232381672, -15.31090095340427304 ) ) ;
#26595=CARTESIAN_POINT ( 'NONE',  ( 11.47327446659168615, 9.267463859335506982, -15.86074700677745852 ) ) ;
#26598=CARTESIAN_POINT ( 'NONE',  ( 10.76353862942338147, 8.717528283631100550, -16.36374602157236779 ) ) ;
#26609=CARTESIAN_POINT ( 'NONE',  ( 12.18385343395297049, 12.51426234204957844, -16.40917503585457737 ) ) ;
#26612=CARTESIAN_POINT ( 'NONE',  ( 34.52649160559821695, -12.12091213808323964, -18.92441241263726326 ) ) ;
#26613=CARTESIAN_POINT ( 'NONE',  ( 19.11618317516819587, 7.271703427217982352, -19.10559232466456692 ) ) ;
#26617=CARTESIAN_POINT ( 'NONE',  ( 19.14398323884976350, 7.495936751868839565, -14.71076302495156263 ) ) ;
#26622=CARTESIAN_POINT ( 'NONE',  ( 19.79269262995316936, -1.159804626089355084, -18.29502107036499581 ) ) ;
#26623=CARTESIAN_POINT ( 'NONE',  ( 18.89783927354708837, -1.194421563772924078, -19.46960211947776287 ) ) ;
#26636=CARTESIAN_POINT ( 'NONE',  ( 11.92109019680886206, 8.606374460406147620, -15.56934379943068336 ) ) ;
#26637=CARTESIAN_POINT ( 'NONE',  ( 27.28761988882141765, -9.265112451392095494, -14.04413049427448001 ) ) ;
#26638=CARTESIAN_POINT ( 'NONE',  ( 22.98083118076628040, -7.181321033737746440, -13.97658420854277850 ) ) ;
#26647=CARTESIAN_POINT ( 'NONE',  ( 20.22088415693689356, -1.238650738454883493, -19.72259765018230482 ) ) ;
#26651=CARTESIAN_POINT ( 'NONE',  ( 10.75323949831978432, 16.48238454209313630, -15.94078111022350619 ) ) ;
#26655=CARTESIAN_POINT ( 'NONE',  ( 24.52797215547132836, -1.897736678990579184, -19.26084780660264073 ) ) ;
#26657=CARTESIAN_POINT ( 'NONE',  ( 20.63001478507949926, 2.108136148055946180, -20.13827832349858937 ) ) ;
#26661=CARTESIAN_POINT ( 'NONE',  ( 31.26470888135608206, -7.466309307788507432, -16.51192723299172727 ) ) ;
#26663=CARTESIAN_POINT ( 'NONE',  ( 19.75542110462093959, -4.861139154975066212, -17.07234110396024818 ) ) ;
#26666=CARTESIAN_POINT ( 'NONE',  ( 25.07290406138036687, -9.006318079059196791, -17.79994936451110732 ) ) ;
#26677=CARTESIAN_POINT ( 'NONE',  ( 15.17188473929424930, 6.803351907998973935, -20.50413427079521256 ) ) ;
#26678=CARTESIAN_POINT ( 'NONE',  ( 33.54536560287652946, -10.49856191242287373, -18.63199441812703583 ) ) ;
#26680=CARTESIAN_POINT ( 'NONE',  ( 11.40798482813988635, 9.566882342703072695, -15.88774718835883348 ) ) ;
#26684=CARTESIAN_POINT ( 'NONE',  ( 9.661887760751893595, 16.25480508276471525, -17.91458275280492884 ) ) ;
#26695=CARTESIAN_POINT ( 'NONE',  ( 11.23176012633392595, 9.056260211165422902, -17.23826859254635835 ) ) ;
#26697=CARTESIAN_POINT ( 'NONE',  ( 32.47832896513632761, -9.914179286496517918, -13.92895715894296771 ) ) ;
#26698=CARTESIAN_POINT ( 'NONE',  ( 26.88053589187069292, -12.95240298029966119, -14.33176627689639382 ) ) ;
#26707=CARTESIAN_POINT ( 'NONE',  ( 31.84774147790582433, -10.54213090804960018, -15.00000000011102763 ) ) ;
#26713=CARTESIAN_POINT ( 'NONE',  ( 13.12468173219994760, 8.571325198882655982, -15.91105655537220009 ) ) ;
#26714=CARTESIAN_POINT ( 'NONE',  ( 35.54859390953724585, -22.18451583373416014, -17.78191007148576475 ) ) ;
#26716=CARTESIAN_POINT ( 'NONE',  ( 9.113844519079130180, 16.17534557870975576, -17.05418121134841414 ) ) ;
#26718=CARTESIAN_POINT ( 'NONE',  ( 24.95482030053459965, -6.624749414579512496, -13.76522253407564733 ) ) ;
#26719=CARTESIAN_POINT ( 'NONE',  ( 12.76739998655820685, 9.838043466917183011, -16.16785800888773394 ) ) ;
#26724=CARTESIAN_POINT ( 'NONE',  ( 12.49742530276927610, 8.569573706352677789, -15.13222638044318735 ) ) ;
#26729=CARTESIAN_POINT ( 'NONE',  ( 12.84373479294319864, 8.511860559062048637, -16.13004233893675377 ) ) ;
#26731=AXIS2_PLACEMENT_3D ( 'NONE', #44, #18654, #18798 ) ;
#26732=CARTESIAN_POINT ( 'NONE',  ( 14.66608887309643272, 3.149405488550426568, -18.09902814372540192 ) ) ;
#26733=CARTESIAN_POINT ( 'NONE',  ( 19.32227194923075331, 0.3423946635036635433, -13.32047942220886583 ) ) ;
#26736=CARTESIAN_POINT ( 'NONE',  ( 36.54460969663918490, -22.16661687567949457, -18.62492107750662029 ) ) ;
#26739=CARTESIAN_POINT ( 'NONE',  ( 17.12833724908345800, 9.171387755021909172, -19.38714867094073213 ) ) ;
#26748=EDGE_CURVE ( 'NONE', #23709, #22459, #22343, .T. ) ;
#26750=CARTESIAN_POINT ( 'NONE',  ( 33.35202879388211983, -12.33251541790028760, -19.68467382345759376 ) ) ;
#26754=CARTESIAN_POINT ( 'NONE',  ( 12.26073475921635669, 9.568819114670704451, -15.31737879056614737 ) ) ;
#26759=CARTESIAN_POINT ( 'NONE',  ( 12.50162201464318557, 8.571418981294288031, -15.12888223836978341 ) ) ;
#26761=CARTESIAN_POINT ( 'NONE',  ( 12.00353595525870887, 7.537035219234042849, -15.50727442731917272 ) ) ;
#26768=CARTESIAN_POINT ( 'NONE',  ( 12.86616790684404421, 9.515247448762703897, -16.11708638872277177 ) ) ;
#26771=CARTESIAN_POINT ( 'NONE',  ( 33.81279548071420038, -11.10283711904122050, -17.43625070980107594 ) ) ;
#26772=CARTESIAN_POINT ( 'NONE',  ( 19.38992137333195842, 2.881095379261479739, -20.30776781288435373 ) ) ;
#26775=CARTESIAN_POINT ( 'NONE',  ( 13.93479307118181509, 9.207276677253689812, -14.11477394318545286 ) ) ;
#26780=CARTESIAN_POINT ( 'NONE',  ( 24.70156281743647142, 0.04986695427254615731, -17.03102378627558977 ) ) ;
#26781=CARTESIAN_POINT ( 'NONE',  ( 22.70908579165946506, -0.2254420654732764706, -12.61778515557981528 ) ) ;
#26794=CARTESIAN_POINT ( 'NONE',  ( 10.82443827553465177, 12.24310121783546634, -16.12906421532448675 ) ) ;
#26796=CARTESIAN_POINT ( 'NONE',  ( 15.44629794785920218, 3.545610805586186132, -16.71614555938632307 ) ) ;
#26797=CARTESIAN_POINT ( 'NONE',  ( 24.19195398915606532, -10.47609993289601427, -15.85356615136800151 ) ) ;
#26805=CARTESIAN_POINT ( 'NONE',  ( 15.70491959545049987, 3.570626008024105680, -15.63470537622339229 ) ) ;
#26809=CARTESIAN_POINT ( 'NONE',  ( 12.27631119714397201, 9.497383584800669354, -15.31093738554958428 ) ) ;
#26812=CARTESIAN_POINT ( 'NONE',  ( 19.40121574091639189, 1.432572567346982240, -13.43353846741550406 ) ) ;
#26814=CARTESIAN_POINT ( 'NONE',  ( 22.56790106455553868, 4.272635385308135803, -18.10442882813315535 ) ) ;
#26819=CARTESIAN_POINT ( 'NONE',  ( 24.92984004655564334, -8.306894832562658593, -19.61321747044761921 ) ) ;
#26820=CARTESIAN_POINT ( 'NONE',  ( 24.74990718239607546, -5.907774739380937667, -20.30682099139976060 ) ) ;
#26822=CARTESIAN_POINT ( 'NONE',  ( 25.90632082398269276, -12.28056132945115841, -15.12647891527467969 ) ) ;
#26834=CARTESIAN_POINT ( 'NONE',  ( 25.61676826379006400, -5.274948970184475172, -14.00514367894158418 ) ) ;
#26836=CARTESIAN_POINT ( 'NONE',  ( 33.25614251967556356, -10.36847857886694868, -17.86465469861353483 ) ) ;
#26839=CARTESIAN_POINT ( 'NONE',  ( 9.695397291186985456, 17.42102709130404747, -17.08803885907851594 ) ) ;
#26843=CARTESIAN_POINT ( 'NONE',  ( 9.661883061612440926, 16.25482663361732705, -17.93331994345748726 ) ) ;
#26854=CARTESIAN_POINT ( 'NONE',  ( 8.944585005148796952, 16.95159128516397118, -17.91410349795882340 ) ) ;
#26857=CARTESIAN_POINT ( 'NONE',  ( 13.46306793452363770, 5.846312397186087750, -15.11995136480861746 ) ) ;
#26859=CARTESIAN_POINT ( 'NONE',  ( 28.50411217586706769, -6.135108760518566129, -18.55796808427148648 ) ) ;
#26873=CARTESIAN_POINT ( 'NONE',  ( 12.56022695423237145, 8.580358410770909217, -16.34122335808152826 ) ) ;
#26874=CARTESIAN_POINT ( 'NONE',  ( 35.24964364652129234, -20.84149066036063047, -20.16262864730545346 ) ) ;
#26877=CARTESIAN_POINT ( 'NONE',  ( 9.109039160554445402, 16.19738356544468516, -17.05632368146133615 ) ) ;
#26879=CARTESIAN_POINT ( 'NONE',  ( 23.84106988684860440, -4.080291168153947545, -13.50610408985603250 ) ) ;
#26880=CARTESIAN_POINT ( 'NONE',  ( 10.35864918915110877, 16.97212501191939538, -17.98596209335946128 ) ) ;
#26882=COLOUR_RGB ( '', 0.66274510, 0.83137255, 0.94901961) ;
#26886=CARTESIAN_POINT ( 'NONE',  ( 11.44040408106239326, 9.418203516307107392, -15.87434068686103394 ) ) ;
#26891=CARTESIAN_POINT ( 'NONE',  ( 9.661883061612440926, 16.25482663361732705, -17.91796598306941135 ) ) ;
#26894=CARTESIAN_POINT ( 'NONE',  ( 19.90219557808113038, 2.290409793443704878, -20.93543687874882053 ) ) ;
#26895=CARTESIAN_POINT ( 'NONE',  ( 16.51977620067554042, 7.986930271725532826, -13.83285890266734519 ) ) ;
#26903=CARTESIAN_POINT ( 'NONE',  ( 15.54217852991911997, 3.796156774867226247, -18.16774540469225485 ) ) ;
#26908=CARTESIAN_POINT ( 'NONE',  ( 32.00110207675911767, -10.95298233446834502, -16.54939777171900417 ) ) ;
#26911=CARTESIAN_POINT ( 'NONE',  ( 12.24518234991790955, 9.516123393600787850, -15.33326918312795328 ) ) ;
#26918=CARTESIAN_POINT ( 'NONE',  ( 12.33231149932895221, 7.515762311178675326, -15.25793818847554562 ) ) ;
#26925=CARTESIAN_POINT ( 'NONE',  ( 12.83220575256047802, 9.540835953717470730, -16.14105854569320542 ) ) ;
#26928=CARTESIAN_POINT ( 'NONE',  ( 35.28777801271252912, -15.52033788203570985, -19.16652784865743442 ) ) ;
#26929=CARTESIAN_POINT ( 'NONE',  ( 20.14386580841007657, 1.771853782379294140, -13.30505882909219295 ) ) ;
#26936=CARTESIAN_POINT ( 'NONE',  ( 17.25677449038176547, 8.733363079223632752, -20.54546673180767158 ) ) ;
#26940=CARTESIAN_POINT ( 'NONE',  ( 22.42023978564754927, -3.655767601918122445, -13.54521809681785172 ) ) ;
#26941=CARTESIAN_POINT ( 'NONE',  ( 16.80134558234102471, 1.491865220098682387, -17.16076555717535257 ) ) ;
#26952=CARTESIAN_POINT ( 'NONE',  ( 11.22348983819090407, 9.093098897663914215, -17.24177177356946800 ) ) ;
#26953=CARTESIAN_POINT ( 'NONE',  ( 12.50481220565295004, 8.572828783776230921, -15.12633959982445653 ) ) ;
#26954=CARTESIAN_POINT ( 'NONE',  ( 26.02348467347448491, -3.622150272347476108, -19.21400332953221124 ) ) ;
#26963=CARTESIAN_POINT ( 'NONE',  ( 25.23810427664335165, -6.496417100615061280, -13.69959235629456629 ) ) ;
#26966=CARTESIAN_POINT ( 'NONE',  ( 11.36920530384750805, 13.65748684056475426, -15.68605758175906040 ) ) ;
#26968=CARTESIAN_POINT ( 'NONE',  ( 32.58918748260075660, -11.04229556371213583, -18.21152344180378080 ) ) ;
#26972=CARTESIAN_POINT ( 'NONE',  ( 26.84970692451943819, -5.812874930055231815, -14.04107299160273037 ) ) ;
#26975=CARTESIAN_POINT ( 'NONE',  ( 16.44673144568935541, 3.517958023484313301, -20.47440421422559353 ) ) ;
#26978=CARTESIAN_POINT ( 'NONE',  ( 27.97271982581976957, -5.335442005784750918, -18.83880583778296725 ) ) ;
#26980=CARTESIAN_POINT ( 'NONE',  ( 24.47917272657372223, 1.093256025350008542, -14.89707007128618699 ) ) ;
#26981=CARTESIAN_POINT ( 'NONE',  ( 25.24878800877705487, -9.370948223588685622, -14.18615728435988288 ) ) ;
#26989=CARTESIAN_POINT ( 'NONE',  ( 25.59007283008577005, -3.201708215360036913, -15.56755918271449168 ) ) ;
#26990=CARTESIAN_POINT ( 'NONE',  ( 18.35279563442798079, 9.979516425631709708, -19.26739628155305439 ) ) ;
#26992=CARTESIAN_POINT ( 'NONE',  ( 32.68023997084922883, -9.631188006280016367, -18.23865791264771730 ) ) ;
#26994=CARTESIAN_POINT ( 'NONE',  ( 9.675370519060759733, 17.51287242109451014, -17.23928541814325399 ) ) ;
#26996=CARTESIAN_POINT ( 'NONE',  ( 13.77718166750865869, 8.859676595473324312, -15.39100258941132182 ) ) ;
#26997=CARTESIAN_POINT ( 'NONE',  ( 9.661883073086391605, 16.25482658099627642, -17.91571305590050400 ) ) ;
#27000=CARTESIAN_POINT ( 'NONE',  ( 11.21346931060482000, 10.45895530107994098, -15.96818619734747458 ) ) ;
#27012=CARTESIAN_POINT ( 'NONE',  ( 8.944584683310379702, 16.95159276115599667, -17.92279151347708677 ) ) ;
#27013=CARTESIAN_POINT ( 'NONE',  ( 31.86596522828317291, -10.28264332119880820, -18.16914504201997360 ) ) ;
#27015=CARTESIAN_POINT ( 'NONE',  ( 30.36731020202829612, -7.149780978071095028, -17.08985122409953306 ) ) ;
#27016=CARTESIAN_POINT ( 'NONE',  ( 24.79209089726652948, -9.725099617967893906, -18.44766554224525734 ) ) ;
#27027=CARTESIAN_POINT ( 'NONE',  ( 13.14084490070201738, 8.578467993704791184, -15.89817422466314945 ) ) ;
#27028=CARTESIAN_POINT ( 'NONE',  ( 33.57416420788476330, -12.34692739235205217, -18.69991813917680190 ) ) ;
#27030=CARTESIAN_POINT ( 'NONE',  ( 9.371932165391852365, 14.99172273419688750, -16.94745289082924344 ) ) ;
#27032=CARTESIAN_POINT ( 'NONE',  ( 26.36224721256908410, -8.875037662531589433, -13.49479840426202948 ) ) ;
#27033=CARTESIAN_POINT ( 'NONE',  ( 12.88201729092779857, 9.522117202545773651, -16.10446439827067167 ) ) ;
#27039=CARTESIAN_POINT ( 'NONE',  ( 12.44984726620633353, 8.550925603015029353, -15.16996558791898231 ) ) ;
#27046=CARTESIAN_POINT ( 'NONE',  ( 13.12468173219994760, 8.571325198882655982, -15.91105655537220009 ) ) ;
#27048=CARTESIAN_POINT ( 'NONE',  ( 13.25083620024415332, 6.663885870737293438, -17.30077526834593016 ) ) ;
#27049=CARTESIAN_POINT ( 'NONE',  ( 16.89391627328321732, 8.154734282165337689, -13.86877251323280014 ) ) ;
#27054=CARTESIAN_POINT ( 'NONE',  ( 25.36810815240369621, -0.9165050883202133791, -18.11329069065276443 ) ) ;
#27060=CARTESIAN_POINT ( 'NONE',  ( 33.29928106196997817, -12.14339677642331772, -19.64090527578606427 ) ) ;
#27066=CARTESIAN_POINT ( 'NONE',  ( 12.27916258238306746, 9.531139938431367753, -15.30618633255685879 ) ) ;
#27067=CARTESIAN_POINT ( 'NONE',  ( 35.28941737075538043, -22.02017293461823755, -20.69856730472309891 ) ) ;
#27072=CARTESIAN_POINT ( 'NONE',  ( 10.64844024921564092, 9.137493944846720950, -16.41957189434499753 ) ) ;
#27078=CARTESIAN_POINT ( 'NONE',  ( 12.86924247997729687, 9.516471784987144744, -16.11464614809275631 ) ) ;
#27079=CARTESIAN_POINT ( 'NONE',  ( 34.34130860390597206, -11.59244310827663149, -18.69197402374579653 ) ) ;
#27080=CARTESIAN_POINT ( 'NONE',  ( 19.71807001554888217, -1.708786246101231532, -19.21472004699903380 ) ) ;
#27086=CARTESIAN_POINT ( 'NONE',  ( 30.76698452600511402, -8.440788201038053273, -16.67119366161266925 ) ) ;
#27087=CARTESIAN_POINT ( 'NONE',  ( 20.64663396976543552, 5.620433075351431995, -17.27584747705915902 ) ) ;
#27089=EDGE_LOOP ( 'NONE', ( #23408, #18442, #13340, #15844, #18778 ) ) ;
#27100=CARTESIAN_POINT ( 'NONE',  ( 11.68823183152383471, 8.106166304734948369, -16.96230016324342671 ) ) ;
#27101=CARTESIAN_POINT ( 'NONE',  ( 12.50016782010997751, 8.570776461014483871, -15.13004124836345632 ) ) ;
#27107=CARTESIAN_POINT ( 'NONE',  ( 9.641350810849047548, 17.66889113945805789, -17.91928203681695564 ) ) ;
#27111=CARTESIAN_POINT ( 'NONE',  ( 23.84106988684860440, -4.080291168153947545, -13.50610408985603250 ) ) ;
#27114=CARTESIAN_POINT ( 'NONE',  ( 11.05541531668977662, 17.68942339022145305, -17.98596209335946128 ) ) ;
#27117=CARTESIAN_POINT ( 'NONE',  ( 23.21730923944814506, -4.364887171357101359, -13.63095412955673247 ) ) ;
#27119=CARTESIAN_POINT ( 'NONE',  ( 20.66677465483945397, 4.408179161683285052, -13.64328152160912033 ) ) ;
#27124=CARTESIAN_POINT ( 'NONE',  ( 18.51594006248351931, 7.284897756227690202, -14.24483590514913089 ) ) ;
#27125=CARTESIAN_POINT ( 'NONE',  ( 24.79321154704742725, 0.1008434151899674086, -19.04223803188042652 ) ) ;
#27128=CARTESIAN_POINT ( 'NONE',  ( 26.07968421886551980, -9.001936657367064498, -13.61655714643126913 ) ) ;
#27137=FACE_OUTER_BOUND ( 'NONE', #9013, .T. ) ;
#27138=CARTESIAN_POINT ( 'NONE',  ( 24.61983070264756890, -3.485318192270607351, -14.59657465048590907 ) ) ;
#27140=CARTESIAN_POINT ( 'NONE',  ( 36.54859390953724585, -22.18451583373416014, -16.94733705004010460 ) ) ;
#27142=CARTESIAN_POINT ( 'NONE',  ( 11.92109019680886206, 8.606374460406147620, -15.56934379943068336 ) ) ;
#27145=CARTESIAN_POINT ( 'NONE',  ( 13.40933447225908992, 7.914523595725266425, -14.40541938743684902 ) ) ;
#27146=CARTESIAN_POINT ( 'NONE',  ( 9.661930010240627809, 16.25461132122415364, -17.91197252329769185 ) ) ;
#27150=CARTESIAN_POINT ( 'NONE',  ( 9.921764701973689426, 16.38287729030320250, -16.50235149140834778 ) ) ;
#27159=CARTESIAN_POINT ( 'NONE',  ( 8.944716491630211763, 16.95098827139963049, -17.88239910762268181 ) ) ;
#27160=CARTESIAN_POINT ( 'NONE',  ( 32.08869746025642655, -10.33200466608398216, -18.78962723441388150 ) ) ;
#27162=CARTESIAN_POINT ( 'NONE',  ( 22.38244025736702625, 4.876565640102752397, -15.59977576251379539 ) ) ;
#27163=CARTESIAN_POINT ( 'NONE',  ( 28.92999000670439713, -5.550862855971650411, -17.57004703619191943 ) ) ;
#27167=CARTESIAN_POINT ( 'NONE',  ( 22.33718609693395862, 3.185771058179875492, -16.53122240148476152 ) ) ;
#27185=CARTESIAN_POINT ( 'NONE',  ( 12.03623766312057519, 9.280706639558555793, -16.68777662621714342 ) ) ;
#27186=CARTESIAN_POINT ( 'NONE',  ( 35.35024494905714221, -20.29343902266242239, -19.25407150246939736 ) ) ;
#27189=CARTESIAN_POINT ( 'NONE',  ( 9.117643650280985668, 16.15792227874146292, -17.05261013695411165 ) ) ;
#27191=CARTESIAN_POINT ( 'NONE',  ( 26.08768104250457753, -11.87935956797728210, -17.28510650846989805 ) ) ;
#27192=CARTESIAN_POINT ( 'NONE',  ( 12.88542016133816048, 9.523620991859985452, -16.10175225048900671 ) ) ;
#27203=CARTESIAN_POINT ( 'NONE',  ( 13.13744203029165369, 8.576964204390579383, -15.90088637244482150 ) ) ;
#27205=CARTESIAN_POINT ( 'NONE',  ( 14.98730560944732559, 2.974898859484017333, -15.20016081292634169 ) ) ;
#27206=CARTESIAN_POINT ( 'NONE',  ( 20.25609397779747312, 2.611002146465201346, -20.92159891259701610 ) ) ;
#27212=CARTESIAN_POINT ( 'NONE',  ( 25.55230692589818631, -0.5649882819070038975, -17.32853901032857280 ) ) ;
#27221=CARTESIAN_POINT ( 'NONE',  ( 33.37634376253905089, -12.42895282922877342, -19.69946502924221932 ) ) ;
#27227=CARTESIAN_POINT ( 'NONE',  ( 11.05541531668977662, 17.68942339022145305, -17.91752729848688830 ) ) ;
#27228=CARTESIAN_POINT ( 'NONE',  ( 32.68951927270060764, -11.07419627511998605, -18.48540492261787449 ) ) ;
#27231=CARTESIAN_POINT ( 'NONE',  ( 10.66860827010606094, 9.045000281972594536, -16.41123175006880075 ) ) ;
#27237=CARTESIAN_POINT ( 'NONE',  ( 12.88542016133816048, 9.523620991859985452, -16.10175225048900671 ) ) ;
#27239=CARTESIAN_POINT ( 'NONE',  ( 36.54006368622684420, -21.14619405898047688, -18.64381572867062076 ) ) ;
#27240=CARTESIAN_POINT ( 'NONE',  ( 20.50636976340433293, -0.9757509181830721356, -19.91080244439677571 ) ) ;
#27248=CARTESIAN_POINT ( 'NONE',  ( 25.05301747714807448, -9.477991407908255894, -18.78921932654604632 ) ) ;
#27250=CARTESIAN_POINT ( 'NONE',  ( 23.05283280155556724, -4.691836721735100468, -12.69353859562758124 ) ) ;
#27262=CARTESIAN_POINT ( 'NONE',  ( 13.10901043280714084, 7.538357286119017786, -15.92110722978107873 ) ) ;
#27263=CARTESIAN_POINT ( 'NONE',  ( 12.43696608443014284, 8.546664718661613591, -15.18012293544581226 ) ) ;
#27264=CARTESIAN_POINT ( 'NONE',  ( 30.02037170576755187, -9.505783518442527225, -18.49971606337314967 ) ) ;
#27267=AXIS2_PLACEMENT_3D ( 'NONE', #25035, #25332, #4423 ) ;
#27270=CARTESIAN_POINT ( 'NONE',  ( 9.643509238790151983, 17.65899231378470446, -17.74106871770035099 ) ) ;
#27274=CARTESIAN_POINT ( 'NONE',  ( 25.36810815240369621, -0.9165050883202133791, -18.11329069065276443 ) ) ;
#27279=CARTESIAN_POINT ( 'NONE',  ( 11.05541531668977662, 17.68942339022145305, -19.66666666666843000 ) ) ;
#27280=CARTESIAN_POINT ( 'NONE',  ( 33.06959603162382422, -11.76507887159725030, -17.56762491042838903 ) ) ;
#27282=CARTESIAN_POINT ( 'NONE',  ( 24.95482030053459965, -6.624749414579512496, -13.76522253407564733 ) ) ;
#27284=CARTESIAN_POINT ( 'NONE',  ( 23.98539618923253514, -1.204509296099786297, -17.73462021633622143 ) ) ;
#27288=CARTESIAN_POINT ( 'NONE',  ( 18.55888777153046121, 10.80885496093247689, -16.87139299526244685 ) ) ;
#27290=CARTESIAN_POINT ( 'NONE',  ( 25.07031029108804887, -10.85539403410516535, -16.40584363908930499 ) ) ;
#27292=CARTESIAN_POINT ( 'NONE',  ( 24.87127057246125972, -9.548149280147088191, -14.79180087847266556 ) ) ;
#27301=CARTESIAN_POINT ( 'NONE',  ( 25.37470919123784086, -4.075530507763302168, -17.99687124876041011 ) ) ;
#27302=CARTESIAN_POINT ( 'NONE',  ( 20.01918758985507196, 7.682949113293006782, -15.97060347488303123 ) ) ;
#27303=CARTESIAN_POINT ( 'NONE',  ( 31.49515780845362301, -9.451207104696591088, -14.88922074032172205 ) ) ;
#27306=CARTESIAN_POINT ( 'NONE',  ( 11.50832337395308436, 9.139936167900076569, -15.84372008594036885 ) ) ;
#27309=CARTESIAN_POINT ( 'NONE',  ( 13.12299649507002464, 8.570581087883812899, -15.91239967140973022 ) ) ;
#27312=CARTESIAN_POINT ( 'NONE',  ( 10.33811693838771717, 18.38618951776012267, -17.92279151347708677 ) ) ;
#27320=CARTESIAN_POINT ( 'NONE',  ( 8.949836677108400806, 16.92750644812532457, -17.70396109330303958 ) ) ;
#27321=CARTESIAN_POINT ( 'NONE',  ( 32.19500574710832552, -10.39459394146955518, -19.06308269698291014 ) ) ;
#27324=CARTESIAN_POINT ( 'NONE',  ( 18.39217644224905257, 0.04847210594158309072, -18.71474297224575878 ) ) ;
#27326=CARTESIAN_POINT ( 'NONE',  ( 27.20456514074317056, -5.347416052021189081, -13.22196079581408235 ) ) ;
#27330=CARTESIAN_POINT ( 'NONE',  ( 26.10879525372914145, -2.341005984040549937, -13.07697618282131913 ) ) ;
#27340=CARTESIAN_POINT ( 'NONE',  ( 32.72889690553877529, -10.93821547844579634, -14.37279655741261486 ) ) ;
#27342=CARTESIAN_POINT ( 'NONE',  ( 10.66860827010606094, 9.045000281972594536, -16.41123175006880075 ) ) ;
#27344=CARTESIAN_POINT ( 'NONE',  ( 25.90632082398269276, -12.28056132945115841, -15.12647891527467969 ) ) ;
#27346=CARTESIAN_POINT ( 'NONE',  ( 12.86835069890237548, 9.516077773083457814, -16.11535690708815594 ) ) ;
#27356=CARTESIAN_POINT ( 'NONE',  ( 13.12278719711289732, 8.570488965836000617, -15.91256645732111430 ) ) ;
#27358=CARTESIAN_POINT ( 'NONE',  ( 22.87580194831562252, -0.07614860672512525908, -19.74465839296685132 ) ) ;
#27359=CARTESIAN_POINT ( 'NONE',  ( 22.64650317123243894, 5.657944777580039997, -17.08144094666319646 ) ) ;
#27366=CARTESIAN_POINT ( 'NONE',  ( 20.39549844898813191, -2.061726703908969505, -13.85117726305786512 ) ) ;
#27374=CARTESIAN_POINT ( 'NONE',  ( 35.12509383387676820, -20.28195432802065312, -20.22992657050740917 ) ) ;
#27379=CARTESIAN_POINT ( 'NONE',  ( 16.01392728624657025, 9.853228751548474662, -15.03783782146776105 ) ) ;
#27380=CARTESIAN_POINT ( 'NONE',  ( 12.24523703128252983, 9.516147632761573050, -15.33322559543412034 ) ) ;
#27381=CARTESIAN_POINT ( 'NONE',  ( 33.54145741815126058, -13.16751478770765793, -19.75123935038191192 ) ) ;
#27384=CARTESIAN_POINT ( 'NONE',  ( 9.641350810849047548, 17.66889113945805789, -17.92015940598198753 ) ) ;
#27391=CARTESIAN_POINT ( 'NONE',  ( 12.87521155010636242, 9.519109623917222152, -16.10988869383489686 ) ) ;
#27393=CARTESIAN_POINT ( 'NONE',  ( 33.33685173283005554, -10.38074443705513161, -18.09276096107157628 ) ) ;
#27395=CARTESIAN_POINT ( 'NONE',  ( 19.61192361542596529, -2.405681417800469291, -14.70675912396028906 ) ) ;
#27401=CARTESIAN_POINT ( 'NONE',  ( 30.68845550234816244, -8.154108532121835395, -15.50657635367809917 ) ) ;
#27402=CARTESIAN_POINT ( 'NONE',  ( 23.39714218815755231, -8.028440028060597200, -17.83143846932372512 ) ) ;
#27410=CARTESIAN_POINT ( 'NONE',  ( 11.24427277393626134, 9.004760228429224966, -17.23264536074314179 ) ) ;
#27411=CARTESIAN_POINT ( 'NONE',  ( 10.33811689237846743, 18.38618972876440338, -17.91642382710546855 ) ) ;
#27416=CARTESIAN_POINT ( 'NONE',  ( 9.641350944112486943, 17.66889052829492002, -17.91441860517739215 ) ) ;
#27418=CARTESIAN_POINT ( 'NONE',  ( 17.88967384018823026, 7.017424582044266224, -15.49508032100559696 ) ) ;
#27421=CARTESIAN_POINT ( 'NONE',  ( 26.31132954256896639, -3.159408024760113509, -14.81636702655834803 ) ) ;
#27425=CARTESIAN_POINT ( 'NONE',  ( 12.24611073458536836, 9.516504178424655791, -15.33253149294119311 ) ) ;
#27426=CARTESIAN_POINT ( 'NONE',  ( 33.75544676243647757, -14.12885555826641593, -19.81592319558764004 ) ) ;
#27428=CARTESIAN_POINT ( 'NONE',  ( 27.91615220763155847, -6.225400021157185826, -17.67258836524805332 ) ) ;
#27430=CARTESIAN_POINT ( 'NONE',  ( 23.60892706051935619, -2.861763136178346212, -14.25286661070829908 ) ) ;
#27435=CARTESIAN_POINT ( 'NONE',  ( 30.28780241637438664, -8.987295266975118935, -19.34112676082218840 ) ) ;
#27436=CARTESIAN_POINT ( 'NONE',  ( 29.37945295281542712, -10.41679561567529433, -17.92877087918597212 ) ) ;
#27448=CARTESIAN_POINT ( 'NONE',  ( 23.79992313191835507, -8.927985498448517632, -17.01055530912027791 ) ) ;
#27449=CARTESIAN_POINT ( 'NONE',  ( 16.38240814442996651, 6.370603895193741373, -13.89573738210111919 ) ) ;
#27451=CARTESIAN_POINT ( 'NONE',  ( 32.21775685856648153, -9.560954865089090760, -16.93152350858319366 ) ) ;
#27454=CARTESIAN_POINT ( 'NONE',  ( 12.50016782010997751, 8.570776461014483871, -15.13004124836345632 ) ) ;
#27458=CARTESIAN_POINT ( 'NONE',  ( 9.708396314890595846, 16.04151092502291931, -17.86831624201546020 ) ) ;
#27462=CARTESIAN_POINT ( 'NONE',  ( 12.71834232392635045, 8.667191563245470576, -14.95615232649864090 ) ) ;
#27468=CARTESIAN_POINT ( 'NONE',  ( 13.81482270056995532, 7.818281081198240834, -15.36100202165747675 ) ) ;
#27469=CARTESIAN_POINT ( 'NONE',  ( 36.01637063434644404, -20.79351858480864124, -21.36424221831693870 ) ) ;
#27470=CARTESIAN_POINT ( 'NONE',  ( 21.98221344960014889, 4.819993630401092410, -14.81438138791982162 ) ) ;
#27471=CARTESIAN_POINT ( 'NONE',  ( 17.37262532792671976, 6.041285449496323068, -14.53661901313261495 ) ) ;
#27474=CARTESIAN_POINT ( 'NONE',  ( 21.92900763033978251, 0.1816185532145172810, -13.27135403042708717 ) ) ;
#27477=DIRECTION ( 'NONE',  ( 0.3331260486002958765, -0.05059491534325381845, -0.9415238660200613285 ) ) ;
#27484=CARTESIAN_POINT ( 'NONE',  ( 34.00275312277798889, -11.14511497259480244, -17.96532559481354596 ) ) ;
#27486=CARTESIAN_POINT ( 'NONE',  ( 10.71071464234916348, 8.878904022500222482, -16.39175934796422851 ) ) ;
#27492=CARTESIAN_POINT ( 'NONE',  ( 10.79618582965528439, 14.96552620561766567, -17.20075070836251996 ) ) ;
#27503=CARTESIAN_POINT ( 'NONE',  ( 13.55939796120610019, 8.763434079353435990, -15.56458004748339619 ) ) ;
#27504=ORIENTED_EDGE ( 'NONE', *, *, #1169, .T. ) ;
#27505=CARTESIAN_POINT ( 'NONE',  ( 19.73194482477335399, 0.5267938184197646923, -13.16654652480547583 ) ) ;
#27506=CARTESIAN_POINT ( 'NONE',  ( 22.00422591904570879, -4.533096263764313072, -16.84388275221259690 ) ) ;
#27507=CARTESIAN_POINT ( 'NONE',  ( 18.75392633456350922, 0.8452085672475394551, -14.97946080469353447 ) ) ;
#27510=CARTESIAN_POINT ( 'NONE',  ( 23.36212950203212557, 2.915605996956767587, -15.34809340432955693 ) ) ;
#27524=CARTESIAN_POINT ( 'NONE',  ( 14.33367420948735393, 6.252843122977492563, -16.41390433006782956 ) ) ;
#27525=CARTESIAN_POINT ( 'NONE',  ( 11.05541531668977662, 17.68942339022145305, -19.66666666666843000 ) ) ;
#27526=CARTESIAN_POINT ( 'NONE',  ( 35.02155038278115740, -19.81678845073966500, -20.19863594638463411 ) ) ;
#27527=EDGE_LOOP ( 'NONE', ( #28744, #4345, #12053, #13789 ) ) ;
#27530=CARTESIAN_POINT ( 'NONE',  ( 12.75517096047518173, 7.625437268557950787, -14.92679923539383680 ) ) ;
#27536=CARTESIAN_POINT ( 'NONE',  ( 12.86751881037522871, 9.515731068868671372, -16.11601834121851340 ) ) ;
#27537=CARTESIAN_POINT ( 'NONE',  ( 33.36027191889437660, -10.38700102556154903, -18.15738432823107473 ) ) ;
#27538=CARTESIAN_POINT ( 'NONE',  ( 21.16681283796276603, -5.103637247178538061, -17.00692323485822754 ) ) ;
#27543=CARTESIAN_POINT ( 'NONE',  ( 24.79209089726652948, -9.725099617967893906, -18.44766554224525734 ) ) ;
#27544=CARTESIAN_POINT ( 'NONE',  ( 25.61803826562323394, -0.4625480611756047078, -19.10237625710802334 ) ) ;
#27555=CARTESIAN_POINT ( 'NONE',  ( 12.51757296969303290, 8.578467993704791184, -15.11616904564172792 ) ) ;
#27561=CARTESIAN_POINT ( 'NONE',  ( 9.879812780108833792, 16.57527415160161510, -16.52987074417163527 ) ) ;
#27562=CARTESIAN_POINT ( 'NONE',  ( 16.99436549934495133, 9.190724047982882894, -15.08166918603070528 ) ) ;
#27565=CARTESIAN_POINT ( 'NONE',  ( 22.97938783112199701, -3.359759438970757017, -19.62490732200095067 ) ) ;
#27568=CARTESIAN_POINT ( 'NONE',  ( 12.24525513380350539, 9.516155168367477657, -15.33321120281095773 ) ) ;
#27569=CARTESIAN_POINT ( 'NONE',  ( 34.96805304670973413, -19.57645325810014114, -20.18246498508359466 ) ) ;
#27571=CARTESIAN_POINT ( 'NONE',  ( 25.23810427664335165, -6.496417100615061280, -13.69959235629456629 ) ) ;
#27574=CARTESIAN_POINT ( 'NONE',  ( 23.40821609032294859, 1.473297984346819245, -16.37969033120859308 ) ) ;
#27577=CARTESIAN_POINT ( 'NONE',  ( 15.33641899704135980, 5.898237403637139664, -14.35162154369138676 ) ) ;
#27578=CARTESIAN_POINT ( 'NONE',  ( 30.58694070296994028, -11.15840821071237698, -14.58880109071565556 ) ) ;
#27591=CARTESIAN_POINT ( 'NONE',  ( 27.87740037347163735, -3.310382910926334521, -16.69022314910379734 ) ) ;
#27592=CARTESIAN_POINT ( 'NONE',  ( 18.25949499138229726, 0.6315596619015936275, -15.69045325149238934 ) ) ;
#27593=CARTESIAN_POINT ( 'NONE',  ( 36.26977878907645447, -21.93194718998534753, -20.87741241889870736 ) ) ;
#27595=CARTESIAN_POINT ( 'NONE',  ( 11.47395765415086188, 9.264374527449886543, -15.86046114005151075 ) ) ;
#27598=CARTESIAN_POINT ( 'NONE',  ( 9.675977061968080051, 16.19018975141917593, -17.88172274351348889 ) ) ;
#27602=CARTESIAN_POINT ( 'NONE',  ( 11.97192087863669663, 8.579774655713777065, -15.53257280409644991 ) ) ;
#27609=CARTESIAN_POINT ( 'NONE',  ( 9.436770671236972774, 14.69436508140356246, -16.92063988783295159 ) ) ;
#27610=CARTESIAN_POINT ( 'NONE',  ( 34.92716911317440065, -20.39278340154575631, -21.20741747040485592 ) ) ;
#27611=CARTESIAN_POINT ( 'NONE',  ( 15.25645860304719292, 2.347722246533389789, -18.19294613283020112 ) ) ;
#27613=CARTESIAN_POINT ( 'NONE',  ( 19.59003110916602708, 6.792398362604423312, -16.15450529561476500 ) ) ;
#27616=CARTESIAN_POINT ( 'NONE',  ( 24.28706804496593463, -0.4963248009486594392, -19.74393692370418307 ) ) ;
#27626=CARTESIAN_POINT ( 'NONE',  ( 35.30103323675335503, -20.07235686745416103, -19.24079536022738068 ) ) ;
#27628=CARTESIAN_POINT ( 'NONE',  ( 10.68833914101186444, 8.961267084878116407, -16.40255713880337751 ) ) ;
#27631=CARTESIAN_POINT ( 'NONE',  ( 29.30346499805017757, -7.722527705200430859, -14.56292402596598556 ) ) ;
#27633=CARTESIAN_POINT ( 'NONE',  ( 10.45680941692980959, 16.52194969480735764, -17.34528143170414083 ) ) ;
#27634=CARTESIAN_POINT ( 'NONE',  ( 13.15390973649967599, 8.859676595473322536, -14.60899741038990562 ) ) ;
#27638=CARTESIAN_POINT ( 'NONE',  ( 12.50226005284522657, 8.571700941790735939, -15.12837371066060221 ) ) ;
#27643=CARTESIAN_POINT ( 'NONE',  ( 9.661930010240627809, 16.25461132122415364, -17.91197252329769185 ) ) ;
#27644=CARTESIAN_POINT ( 'NONE',  ( 17.51795708650258732, -0.4494001013054305660, -15.13702969726144509 ) ) ;
#27645=CARTESIAN_POINT ( 'NONE',  ( 24.91993355315554837, -1.627520125476753510, -17.55906114018776876 ) ) ;
#27646=CARTESIAN_POINT ( 'NONE',  ( 21.65198393244800812, 4.573788442230395823, -17.29480057625502454 ) ) ;
#27654=CARTESIAN_POINT ( 'NONE',  ( 23.76365953361780470, 2.837943588559999508, -16.54419024451982168 ) ) ;
#27659=CARTESIAN_POINT ( 'NONE',  ( 10.45306510330410177, 16.53912159438435125, -17.34933906371858114 ) ) ;
#27666=CARTESIAN_POINT ( 'NONE',  ( 15.22033579473957410, 7.355362781181614018, -19.64495939069069763 ) ) ;
#27667=CARTESIAN_POINT ( 'NONE',  ( 11.60030688134799171, 15.19048121717941768, -16.65049206281727479 ) ) ;
#27668=CARTESIAN_POINT ( 'NONE',  ( 34.54007435814109783, -17.65377171698271752, -20.05309729467257540 ) ) ;
#27673=CARTESIAN_POINT ( 'NONE',  ( 9.916775705961365261, 16.40575746196480011, -16.50441451066904364 ) ) ;
#27675=CARTESIAN_POINT ( 'NONE',  ( 12.76278909782508997, 7.628803627606831839, -14.92072746316176790 ) ) ;
#27681=CARTESIAN_POINT ( 'NONE',  ( 12.87265939729807762, 9.517981781931423413, -16.11192280467173532 ) ) ;
#27683=CARTESIAN_POINT ( 'NONE',  ( 35.70376052765831787, -18.38912696963886617, -20.33459093173238941 ) ) ;
#27684=CARTESIAN_POINT ( 'NONE',  ( 26.85315702054868936, -3.432285194908070380, -17.01323758698984889 ) ) ;
#27692=CARTESIAN_POINT ( 'NONE',  ( 18.51435942584036454, 8.743714487506315081, -19.56092670885941587 ) ) ;
#27694=CARTESIAN_POINT ( 'NONE',  ( 20.69116929084294298, -5.269815114589342819, -18.46063674707264468 ) ) ;
#27704=CARTESIAN_POINT ( 'NONE',  ( 10.72892505862787971, 16.59389366189031634, -15.95083598634710320 ) ) ;
#27705=CARTESIAN_POINT ( 'NONE',  ( 26.64416741123070054, -12.70369174447049332, -17.39020166599120643 ) ) ;
#27709=CARTESIAN_POINT ( 'NONE',  ( 9.695397291186985456, 17.42102709130404747, -17.08803885907851594 ) ) ;
#27711=CARTESIAN_POINT ( 'NONE',  ( 18.48188012193690710, 6.385789046977964567, -18.71539758422269628 ) ) ;
#27714=CARTESIAN_POINT ( 'NONE',  ( 26.48263329513011755, -12.06126822337667903, -13.95730679897583038 ) ) ;
#27718=CARTESIAN_POINT ( 'NONE',  ( 12.29957980484737767, 9.540162674316999158, -15.28991344586433421 ) ) ;
#27720=CARTESIAN_POINT ( 'NONE',  ( 33.44337896868773186, -12.72690026786775341, -19.72159258799634074 ) ) ;
#27721=CARTESIAN_POINT ( 'NONE',  ( 14.39533340154967433, 6.572929804808670617, -18.54476805420031837 ) ) ;
#27723=CARTESIAN_POINT ( 'NONE',  ( 21.76348650023563636, -1.483442554740824537, -14.70963264896640155 ) ) ;
#27728=CARTESIAN_POINT ( 'NONE',  ( 14.06424326207706699, 5.752694757912038881, -19.02294901845717945 ) ) ;
#27729=CARTESIAN_POINT ( 'NONE',  ( 25.37029659992048281, -10.87484012800900501, -14.78472363349550811 ) ) ;
#27743=CARTESIAN_POINT ( 'NONE',  ( 25.74978097135661770, 0.6894738977563982241, -15.43585696046938160 ) ) ;
#27744=CARTESIAN_POINT ( 'NONE',  ( 13.98191416104776685, 5.331502061239655532, -16.22335970869868760 ) ) ;
#27745=CARTESIAN_POINT ( 'NONE',  ( 34.31408884023914396, -17.63853849290766362, -21.02710884213126263 ) ) ;
#27747=CARTESIAN_POINT ( 'NONE',  ( 11.47748818427356987, 9.248962635895034978, -15.85894168489154765 ) ) ;
#27750=CARTESIAN_POINT ( 'NONE',  ( 9.667846996725693032, 16.22747526696303666, -17.88508502774671882 ) ) ;
#27754=CARTESIAN_POINT ( 'NONE',  ( 12.48799528366842360, 8.565546312597838607, -15.13973160209665991 ) ) ;
#27760=CARTESIAN_POINT ( 'NONE',  ( 9.101278670497288559, 16.23297416207913813, -17.06093009358445300 ) ) ;
#27761=CARTESIAN_POINT ( 'NONE',  ( 35.54317590287104167, -23.16017559978188345, -18.72806989825276247 ) ) ;
#27763=CARTESIAN_POINT ( 'NONE',  ( 20.51677437365689372, 7.544110930723523012, -19.48516728630390915 ) ) ;
#27765=CARTESIAN_POINT ( 'NONE',  ( 19.16431125762126442, 9.782083453288988650, -17.54400000489614087 ) ) ;
#27768=CIRCLE ( 'NONE', #14548, 0.4999999999999986677 ) ;
#27771=CARTESIAN_POINT ( 'NONE',  ( 22.91777464530744268, -8.256078323855359002, -14.14386909076557686 ) ) ;
#27779=CARTESIAN_POINT ( 'NONE',  ( 35.44226431226860541, -20.70683327756191616, -19.15799893943290755 ) ) ;
#27781=CARTESIAN_POINT ( 'NONE',  ( 11.38288633050183307, 7.831121701799675705, -15.95859485361821939 ) ) ;
#27786=CARTESIAN_POINT ( 'NONE',  ( 10.47401950373780899, 16.44302204293020964, -17.33397781699859053 ) ) ;
#27797=CARTESIAN_POINT ( 'NONE',  ( 9.684081875198721434, 16.15302004482010645, -17.87837111813898616 ) ) ;
#27798=CARTESIAN_POINT ( 'NONE',  ( 17.49129197179432538, 0.06586305242593921971, -19.15772692538415356 ) ) ;
#27799=CARTESIAN_POINT ( 'NONE',  ( 22.28228072301589080, -4.238876526682920698, -17.70252831752424427 ) ) ;
#27800=CARTESIAN_POINT ( 'NONE',  ( 22.98323032518889519, 2.094654362561221284, -17.51695658672324640 ) ) ;
#27807=CARTESIAN_POINT ( 'NONE',  ( 27.83100014064079275, -5.545984359997562230, -15.13782040115233052 ) ) ;
#27814=CARTESIAN_POINT ( 'NONE',  ( 10.41412541532089620, 16.71770396712979689, -17.42473314453425814 ) ) ;
#27820=CARTESIAN_POINT ( 'NONE',  ( 14.73401617531889229, 6.408058468588501810, -15.60580005407095960 ) ) ;
#27821=CARTESIAN_POINT ( 'NONE',  ( 11.05541802266494855, 17.68941098027438841, -17.91029082024824959 ) ) ;
#27822=CARTESIAN_POINT ( 'NONE',  ( 33.96943610671532809, -15.09019632882451134, -19.88060704079178720 ) ) ;
#27827=CARTESIAN_POINT ( 'NONE',  ( 9.695397291186985456, 17.42102709130404747, -17.08803885907851594 ) ) ;
#27829=CARTESIAN_POINT ( 'NONE',  ( 12.75399582221978889, 7.624919616107145970, -14.92773571455457216 ) ) ;
#27837=CARTESIAN_POINT ( 'NONE',  ( 10.99070134719017311, 14.07345324724201063, -17.12031169937328201 ) ) ;
#27839=CARTESIAN_POINT ( 'NONE',  ( 33.24108837279852224, -10.36619216719171632, -17.82210672427467912 ) ) ;
#27840=CARTESIAN_POINT ( 'NONE',  ( 23.60870351872479844, -7.222488552757559077, -14.83554404960226947 ) ) ;
#27846=CARTESIAN_POINT ( 'NONE',  ( 14.70507544977879100, 5.024503852999842479, -17.88552553980999704 ) ) ;
#27848=CARTESIAN_POINT ( 'NONE',  ( 27.00045552667489446, -4.635344809676953837, -19.07524480842047510 ) ) ;
#27856=CARTESIAN_POINT ( 'NONE',  ( 10.48326151898216452, 17.72053796952357985, -16.40639007392780258 ) ) ;
#27865=CARTESIAN_POINT ( 'NONE',  ( 11.47231678315799464, 9.271847796573304379, -15.86114366194887815 ) ) ;
#27868=CARTESIAN_POINT ( 'NONE',  ( 18.99253871878172717, 7.061292173911923875, -17.66947577672478431 ) ) ;
#27872=CARTESIAN_POINT ( 'NONE',  ( 29.30346499805017757, -7.722527705200430859, -14.56292402596598556 ) ) ;
#27876=CARTESIAN_POINT ( 'NONE',  ( 11.27624053946810889, 16.67669076989127674, -16.78450489582619554 ) ) ;
#27877=CARTESIAN_POINT ( 'NONE',  ( 35.24964364652129234, -20.84149066036063047, -20.16262864730545346 ) ) ;
#27880=CARTESIAN_POINT ( 'NONE',  ( 21.93691487550926311, -3.207747311472892271, -17.94368141530714311 ) ) ;
#27884=CARTESIAN_POINT ( 'NONE',  ( 20.51209521231993094, 3.083376493849706801, -19.38174501956431683 ) ) ;
#27885=CARTESIAN_POINT ( 'NONE',  ( 29.44447141382201139, -6.373630389881236091, -17.32815070419105297 ) ) ;
#27893=CARTESIAN_POINT ( 'NONE',  ( 9.641350777746193756, 17.66889129127197577, -17.91630266473768884 ) ) ;
#27894=CARTESIAN_POINT ( 'NONE',  ( 26.42757832573366983, -5.232593867482060013, -19.46531670327460617 ) ) ;
#27895=CARTESIAN_POINT ( 'NONE',  ( 20.13607245741800611, 4.456688099076253629, -14.49627829575511129 ) ) ;
#27897=CARTESIAN_POINT ( 'NONE',  ( 33.02439791605519304, -11.93986616049457261, -20.58189241239533374 ) ) ;
#27905=CARTESIAN_POINT ( 'NONE',  ( 16.79143122783437292, 7.330551994622505063, -14.54187356113185103 ) ) ;
#27908=CARTESIAN_POINT ( 'NONE',  ( 12.49428694376680049, 8.568214790255201052, -15.13472557389765072 ) ) ;
#27912=CARTESIAN_POINT ( 'NONE',  ( 17.08157517049449581, 7.460725202527481947, -14.57009041681831896 ) ) ;
#27915=CARTESIAN_POINT ( 'NONE',  ( 35.54859390953724585, -23.18451583373416014, -17.64281456791166391 ) ) ;
#27916=CARTESIAN_POINT ( 'NONE',  ( 21.93691487550926311, -3.207747311472892271, -17.94368141530714311 ) ) ;
#27917=CARTESIAN_POINT ( 'NONE',  ( 17.81745789538532776, 7.988559130291253751, -20.18242036267038841 ) ) ;
#27918=CARTESIAN_POINT ( 'NONE',  ( 25.20714760837546464, -2.665945389627573991, -12.53535894516201665 ) ) ;
#27927=CARTESIAN_POINT ( 'NONE',  ( 32.35289370704636980, -10.23129387835982129, -15.31177623828282108 ) ) ;
#27928=CARTESIAN_POINT ( 'NONE',  ( 11.68234546060339163, 7.643720436761259229, -15.74430661255668262 ) ) ;
#27936=CARTESIAN_POINT ( 'NONE',  ( 10.47169460192958645, 16.45368433897878191, -17.33494088278173351 ) ) ;
#27948=CARTESIAN_POINT ( 'NONE',  ( 9.664814466656260095, 16.24138283641780944, -17.88982567228806175 ) ) ;
#27949=CARTESIAN_POINT ( 'NONE',  ( 19.32227194923075331, 0.3423946635036635433, -13.32047942220886583 ) ) ;
#27950=CARTESIAN_POINT ( 'NONE',  ( 22.18457322443145330, -2.050108300791262828, -13.94172724511641448 ) ) ;
#27951=CARTESIAN_POINT ( 'NONE',  ( 21.84445237452005628, 0.7298858868756038509, -19.18266460542251295 ) ) ;
#27955=CARTESIAN_POINT ( 'NONE',  ( 22.90372073960079646, -4.505259139820817715, -13.75793632099288111 ) ) ;
#27962=CARTESIAN_POINT ( 'NONE',  ( 10.35864918915110877, 16.97212501191939538, -17.93331994345748370 ) ) ;
#27965=CARTESIAN_POINT ( 'NONE',  ( 11.22273001195053155, 9.096583557657577757, -17.24208598844832352 ) ) ;
#27969=CARTESIAN_POINT ( 'NONE',  ( 21.10023079691774228, -0.4353598523292347422, -20.14113737667230097 ) ) ;
#27971=CARTESIAN_POINT ( 'NONE',  ( 11.29232397858413250, 16.60293006794363535, -16.77785382704750461 ) ) ;
#27972=CARTESIAN_POINT ( 'NONE',  ( 35.54859390953724585, -22.18451583373416014, -18.19919658220850778 ) ) ;
#27976=CARTESIAN_POINT ( 'NONE',  ( 9.910898653440767703, 16.43271037397421708, -16.50709950392603531 ) ) ;
#27978=CARTESIAN_POINT ( 'NONE',  ( 9.641350777746193756, 17.66889129127197577, -17.91630266473768884 ) ) ;
#27984=CARTESIAN_POINT ( 'NONE',  ( 10.46247360472336041, 16.49597300757040230, -17.34042816522791952 ) ) ;
#27986=CARTESIAN_POINT ( 'NONE',  ( 35.98907965336992731, -19.67091466371804742, -20.42083605867238205 ) ) ;
#27987=CARTESIAN_POINT ( 'NONE',  ( 27.20760296572909809, -8.488227175050779394, -13.35743234967312354 ) ) ;
#27993=CARTESIAN_POINT ( 'NONE',  ( 31.37220973900873489, -11.08107799475175348, -13.94606079199652982 ) ) ;
#27994=CARTESIAN_POINT ( 'NONE',  ( 27.46788175125265141, -10.83975311022233079, -17.61709057740623408 ) ) ;
#28004=CARTESIAN_POINT ( 'NONE',  ( 10.71759363061643100, 16.64586103517192939, -15.95557720612771746 ) ) ;
#28009=CARTESIAN_POINT ( 'NONE',  ( 9.921764701973689426, 16.38287729030320250, -16.50235149140834778 ) ) ;
#28011=CARTESIAN_POINT ( 'NONE',  ( 27.90801785101615096, -12.26699769840798204, -14.39122685649866717 ) ) ;
#28014=CARTESIAN_POINT ( 'NONE',  ( 26.57062215293289498, -11.41726559881178638, -18.09730928560479057 ) ) ;
#28017=CARTESIAN_POINT ( 'NONE',  ( 11.20364811077027767, 17.00960890128215297, -16.86645280501126365 ) ) ;
#28018=CARTESIAN_POINT ( 'NONE',  ( 35.54170021948790748, -21.15354613602950096, -18.58520066250327929 ) ) ;
#28019=CARTESIAN_POINT ( 'NONE',  ( 16.01392728624657025, 9.853228751548474662, -15.03783782146776105 ) ) ;
#28024=CARTESIAN_POINT ( 'NONE',  ( 26.06151603483908019, -7.281686956891486595, -19.93845510724469960 ) ) ;
#28028=CARTESIAN_POINT ( 'NONE',  ( 17.90640022563237110, 0.6078909361919438981, -17.24624654394265377 ) ) ;
#28029=CARTESIAN_POINT ( 'NONE',  ( 17.47084574460127371, 4.633898707001591788, -15.02533140066315198 ) ) ;
#28040=CARTESIAN_POINT ( 'NONE',  ( 9.907423389235603395, 16.44864837861227969, -16.50891839478055090 ) ) ;
#28041=CARTESIAN_POINT ( 'NONE',  ( 24.43881766525553090, -7.056818123010307531, -19.17719463634885102 ) ) ;
#28042=CARTESIAN_POINT ( 'NONE',  ( 19.79269262995316936, -1.159804626089355084, -18.29502107036499581 ) ) ;
#28043=CARTESIAN_POINT ( 'NONE',  ( 36.54859390953724585, -23.18451583373416014, -17.99055332684694974 ) ) ;
#28046=CARTESIAN_POINT ( 'NONE',  ( 12.71834232392635045, 8.667191563245470576, -14.95615232649864090 ) ) ;
#28053=CARTESIAN_POINT ( 'NONE',  ( 10.71759363061643100, 16.64586103517192939, -15.95557720612771746 ) ) ;
#28058=APPLICATION_CONTEXT ( 'automotive_design' ) ;
#28059=CARTESIAN_POINT ( 'NONE',  ( 15.46244301724551740, 3.702889819443702990, -17.82701508041758842 ) ) ;
#28061=CARTESIAN_POINT ( 'NONE',  ( 30.07451494818246474, -7.670792865742884992, -18.22619146169064663 ) ) ;
#28063=CARTESIAN_POINT ( 'NONE',  ( 33.45813146310553066, -13.79317541067231723, -20.76837346131055639 ) ) ;
#28064=CARTESIAN_POINT ( 'NONE',  ( 20.68391251823057075, 0.6588762160484964436, -13.99488169736409304 ) ) ;
#28065=CARTESIAN_POINT ( 'NONE',  ( 19.52759782329482263, 6.073010510103808990, -18.47256557099433394 ) ) ;
#28066=CARTESIAN_POINT ( 'NONE',  ( 24.92117679868390923, -7.366661744264540346, -12.55155079749028779 ) ) ;
#28077=CARTESIAN_POINT ( 'NONE',  ( 36.10807049912983757, -19.20547750251314767, -19.41448258861096932 ) ) ;
#28078=CARTESIAN_POINT ( 'NONE',  ( 12.86487521014348623, 7.673917307032582791, -14.83936302970355037 ) ) ;
#28082=CARTESIAN_POINT ( 'NONE',  ( 10.47230989469697882, 16.45086252791593751, -17.33468480047602256 ) ) ;
#28090=CARTESIAN_POINT ( 'NONE',  ( 9.667469407758799704, 16.22920693809672343, -17.88529630510330293 ) ) ;
#28093=CARTESIAN_POINT ( 'NONE',  ( 26.57181397551241275, -7.970695015363167713, -12.68872038106934852 ) ) ;
#28094=CARTESIAN_POINT ( 'NONE',  ( 20.73027244251523626, 3.305903845835247434, -19.25852547563239625 ) ) ;
#28099=CARTESIAN_POINT ( 'NONE',  ( 26.47511176763426377, -7.718147522161595830, -18.64721581247919602 ) ) ;
#28113=CARTESIAN_POINT ( 'NONE',  ( 10.35864927600819740, 16.97212461358170188, -17.91506874352199574 ) ) ;
#28114=CARTESIAN_POINT ( 'NONE',  ( 35.54859390953724585, -22.18451583373416014, -17.64281456791166036 ) ) ;
#28115=CARTESIAN_POINT ( 'NONE',  ( 33.47012763672258728, -12.84706786418751534, -19.72967806864707541 ) ) ;
#28118=CARTESIAN_POINT ( 'NONE',  ( 13.59703899429919005, 7.722038565090276308, -15.53457947969411634 ) ) ;
#28121=CARTESIAN_POINT ( 'NONE',  ( 18.98200677837107264, -2.562081333921657933, -16.63161468174866187 ) ) ;
#28122=CARTESIAN_POINT ( 'NONE',  ( 11.13911793526871463, 17.30555251181618814, -17.04533519337964975 ) ) ;
#28126=CARTESIAN_POINT ( 'NONE',  ( 9.641890818133653340, 17.66641459721583374, -17.82828029666912073 ) ) ;
#28129=CARTESIAN_POINT ( 'NONE',  ( 11.31072706937237982, 10.01291882189198112, -15.92796669285280764 ) ) ;
#28135=CARTESIAN_POINT ( 'NONE',  ( 10.47262648896379922, 16.44941058625191133, -17.33455387760982447 ) ) ;
#28138=CARTESIAN_POINT ( 'NONE',  ( 32.66938126488236804, -9.629547215342803668, -18.20796273874843507 ) ) ;
#28139=CARTESIAN_POINT ( 'NONE',  ( 13.52175692814481067, 9.804829593628518580, -15.59458061523717909 ) ) ;
#28140=CARTESIAN_POINT ( 'NONE',  ( 23.56138260001205964, -6.829566487537672259, -18.05074380722902916 ) ) ;
#28147=CARTESIAN_POINT ( 'NONE',  ( 19.85629768685782537, 6.556105584440964584, -17.58075288388961965 ) ) ;
#28148=CARTESIAN_POINT ( 'NONE',  ( 30.87383483136289541, -10.13329766739009052, -15.36655316835725138 ) ) ;
#28161=CARTESIAN_POINT ( 'NONE',  ( 10.34291491886349235, 18.36418536769788901, -17.61263766090776528 ) ) ;
#28166=CARTESIAN_POINT ( 'NONE',  ( 11.46471852075427478, 9.306694396509932687, -15.86428581073749378 ) ) ;
#28167=CARTESIAN_POINT ( 'NONE',  ( 22.65897993816424716, 3.718266075228530365, -15.21131701836175232 ) ) ;
#28170=CARTESIAN_POINT ( 'NONE',  ( 29.76939623719675510, -8.219725197086590995, -17.35520659559267287 ) ) ;
#28171=ORIENTED_EDGE ( 'NONE', *, *, #26748, .F. ) ;
#28173=CARTESIAN_POINT ( 'NONE',  ( 11.24654891281740987, 16.81286035451327265, -16.80493547870787197 ) ) ;
#28175=CARTESIAN_POINT ( 'NONE',  ( 35.44226431226860541, -20.70683327756191616, -19.15799893943290755 ) ) ;
#28179=CARTESIAN_POINT ( 'NONE',  ( 28.48873154519036888, -4.568419848414010609, -17.42663535687301035 ) ) ;
#28184=CARTESIAN_POINT ( 'NONE',  ( 18.25949499138229726, 0.6315596619015936275, -15.69045325149238934 ) ) ;
#28186=CARTESIAN_POINT ( 'NONE',  ( 15.27107031639597423, 6.121678041989828678, -18.36639460046777828 ) ) ;
#28198=CARTESIAN_POINT ( 'NONE',  ( 9.675370519060759733, 17.51287242109451014, -17.23928541814325399 ) ) ;
#28199=CARTESIAN_POINT ( 'NONE',  ( 20.13453040791782911, -1.388291987844697317, -13.01173725324373009 ) ) ;
#28200=CARTESIAN_POINT ( 'NONE',  ( 19.47299019774181161, -1.479546722229555744, -17.51644493673600067 ) ) ;
#28201=CARTESIAN_POINT ( 'NONE',  ( 36.54276536429808431, -23.15833126744076509, -18.75760452913613463 ) ) ;
#28208=CARTESIAN_POINT ( 'NONE',  ( 15.87806330829146617, 7.947701475055697351, -19.83831759000646855 ) ) ;
#28211=CARTESIAN_POINT ( 'NONE',  ( 10.72284644870490489, 16.62177094183959980, -15.95334970537801134 ) ) ;
#28215=CARTESIAN_POINT ( 'NONE',  ( 36.04859390953723874, -22.18451583373416014, -15.00000000000000000 ) ) ;
#28219=CARTESIAN_POINT ( 'NONE',  ( 15.87806330829146617, 7.947701475055697351, -19.83831759000646855 ) ) ;
#28220=CARTESIAN_POINT ( 'NONE',  ( 30.36731020202829612, -7.149780978071095028, -17.08985122409953306 ) ) ;
#28222=CARTESIAN_POINT ( 'NONE',  ( 35.54502023521215648, -22.16846120802060938, -18.59538644662325524 ) ) ;
#28223=CARTESIAN_POINT ( 'NONE',  ( 23.04877348721027630, -0.9239720737610787049, -14.85003467231304342 ) ) ;
#28224=CARTESIAN_POINT ( 'NONE',  ( 18.37740474667574730, 3.980509343919368614, -15.11632106699347844 ) ) ;
#28226=CARTESIAN_POINT ( 'NONE',  ( 29.75294099516071711, -10.02427176990993196, -17.65830536592410738 ) ) ;
#28233=CARTESIAN_POINT ( 'NONE',  ( 34.52649160559821695, -12.12091213808323964, -18.92441241263726326 ) ) ;
#28234=CARTESIAN_POINT ( 'NONE',  ( 9.641350835837977584, 17.66889102485563612, -17.91507476468484938 ) ) ;
#28238=CARTESIAN_POINT ( 'NONE',  ( 12.03206445085756116, 9.298183410334813104, -16.68962916345529024 ) ) ;
#28252=CARTESIAN_POINT ( 'NONE',  ( 9.675977061968080051, 16.19018975141917593, -17.88172274351348889 ) ) ;
#28253=CARTESIAN_POINT ( 'NONE',  ( 23.44948677240984480, -6.246615351793893822, -14.99377964970044808 ) ) ;
#28254=CARTESIAN_POINT ( 'NONE',  ( 26.78588127033857091, -2.187643107580064861, -16.18476928258297676 ) ) ;
#28257=PLANE ( 'NONE',  #15185 ) ;
#28258=CARTESIAN_POINT ( 'NONE',  ( 27.91615220763155847, -6.225400021157185826, -17.67258836524805332 ) ) ;
#28267=CARTESIAN_POINT ( 'NONE',  ( 10.47224519147693478, 16.45115926513079074, -17.33471155705291977 ) ) ;
#28270=CARTESIAN_POINT ( 'NONE',  ( 32.74314609665832165, -11.10724048739539782, -18.62249297335446840 ) ) ;
#28272=CARTESIAN_POINT ( 'NONE',  ( 13.38012098442259834, 7.626178612778168109, -15.70746696265163145 ) ) ;
#28274=CARTESIAN_POINT ( 'NONE',  ( 17.21692058948253035, 4.245457944912791604, -14.13226496128363863 ) ) ;
#28275=CARTESIAN_POINT ( 'NONE',  ( 11.27864710625743427, 16.66565394782951515, -16.78350969486689692 ) ) ;
#28280=CARTESIAN_POINT ( 'NONE',  ( 9.641566850259106758, 17.66790035518494051, -17.86107206016944460 ) ) ;
#28283=CARTESIAN_POINT ( 'NONE',  ( 9.642214727206800617, 17.66492910891761525, -17.80644250212319690 ) ) ;
#28289=CARTESIAN_POINT ( 'NONE',  ( 10.47008273352651564, 16.46107657294071203, -17.33567129194344858 ) ) ;
#28292=CARTESIAN_POINT ( 'NONE',  ( 36.09161981528372110, -20.13157329416283048, -20.44814669990763889 ) ) ;
#28293=CARTESIAN_POINT ( 'NONE',  ( 27.76312469413510442, -10.32446017237915648, -18.80420148706337358 ) ) ;
#28294=CARTESIAN_POINT ( 'NONE',  ( 26.72358035960067824, -3.685970424986596772, -17.59444040205794835 ) ) ;
#28297=CARTESIAN_POINT ( 'NONE',  ( 35.06179249480944549, -15.50510465796065596, -20.14053939611612520 ) ) ;
#28299=CARTESIAN_POINT ( 'NONE',  ( 19.04375517570889187, 9.961537237715642590, -16.65452713690489617 ) ) ;
#28300=CARTESIAN_POINT ( 'NONE',  ( 29.74223563811278481, -10.39579538818624549, -13.90533736129563813 ) ) ;
#28311=CARTESIAN_POINT ( 'NONE',  ( 10.69507909363156628, 16.74911557172037391, -15.96836912279556309 ) ) ;
#28315=CARTESIAN_POINT ( 'NONE',  ( 9.917332382238186028, 16.40320447359955125, -16.50418441153501448 ) ) ;
#28319=CARTESIAN_POINT ( 'NONE',  ( 9.667809135389937580, 16.22764890387498227, -17.88510185254740747 ) ) ;
#28320=CARTESIAN_POINT ( 'NONE',  ( 23.36829581039676640, 3.373260575288004937, -18.04565522708177738 ) ) ;
#28324=CARTESIAN_POINT ( 'NONE',  ( 27.44219139316946965, -6.774709612358828181, -18.29578255718776703 ) ) ;
#28328=CARTESIAN_POINT ( 'NONE',  ( 11.21766632152761822, 16.94531959984159641, -16.84123939818963223 ) ) ;
#28332=CARTESIAN_POINT ( 'NONE',  ( 33.36629945566365052, -11.89386221509426633, -18.35752312617820081 ) ) ;
#28334=CARTESIAN_POINT ( 'NONE',  ( 15.73644607668725826, 9.740111719757674535, -14.94734896276200153 ) ) ;
#28336=CARTESIAN_POINT ( 'NONE',  ( 9.084523633786250940, 16.30981489620654301, -17.07623073379102507 ) ) ;
#28337=CARTESIAN_POINT ( 'NONE',  ( 25.50153931649120764, -9.195696458170099064, -12.32940773450113170 ) ) ;
#28341=CARTESIAN_POINT ( 'NONE',  ( 20.38603433104324480, 7.363110203939331022, -17.91596102798271062 ) ) ;
#28342=CARTESIAN_POINT ( 'NONE',  ( 17.06308625499319831, 6.674173717519480853, -15.25088821959635865 ) ) ;
#28353=CARTESIAN_POINT ( 'NONE',  ( 9.641404825192898542, 17.66864342279195199, -17.88841768828662282 ) ) ;
#28354=CARTESIAN_POINT ( 'NONE',  ( 28.66609726738115071, -6.663921799113727396, -16.65640135049372006 ) ) ;
#28355=CARTESIAN_POINT ( 'NONE',  ( 20.31878617967674217, -0.6648838724932636390, -18.90140657046049455 ) ) ;
#28356=CARTESIAN_POINT ( 'NONE',  ( 32.98128152813007574, -11.80310687477359188, -20.53574887303233609 ) ) ;
#28363=CARTESIAN_POINT ( 'NONE',  ( 15.22033579473957410, 7.355362781181614018, -19.64495939069069763 ) ) ;
#28366=CARTESIAN_POINT ( 'NONE',  ( 10.33811712360892443, 18.38618866831204102, -17.91390369733608523 ) ) ;
#28369=CARTESIAN_POINT ( 'NONE',  ( 14.33367420948735393, 6.252843122977492563, -16.41390433006782956 ) ) ;
#28370=CARTESIAN_POINT ( 'NONE',  ( 14.32916401545863039, 6.225515681311286187, -14.04012878508491369 ) ) ;
#28372=CARTESIAN_POINT ( 'NONE',  ( 35.54787733059053778, -22.18129662410796854, -18.46719521006932396 ) ) ;
#28374=CARTESIAN_POINT ( 'NONE',  ( 24.19805618307960060, -0.7920880973371497991, -16.79971198345035432 ) ) ;
#28377=CARTESIAN_POINT ( 'NONE',  ( 21.44849557978440657, 3.047722651366359781, -15.04725200041975341 ) ) ;
#28378=CARTESIAN_POINT ( 'NONE',  ( 27.75006011364712322, -11.91879133414019698, -17.49150313904273801 ) ) ;
#28386=CARTESIAN_POINT ( 'NONE',  ( 34.66364242521329686, -12.71642730124038501, -18.97786663347613256 ) ) ;
#28388=CARTESIAN_POINT ( 'NONE',  ( 9.641350810849047548, 17.66889113945805789, -17.92015940598198753 ) ) ;
#28392=CARTESIAN_POINT ( 'NONE',  ( 12.14965596459611774, 8.983642127099937369, -16.62385966901067391 ) ) ;
#28402=CARTESIAN_POINT ( 'NONE',  ( 13.37103985619203783, 7.622196798368539028, -15.71470239503888422 ) ) ;
#28403=CARTESIAN_POINT ( 'NONE',  ( 25.76376746566330311, -3.589579415956118069, -17.31313795625071350 ) ) ;
#28405=CARTESIAN_POINT ( 'NONE',  ( 21.34960977245966873, -3.524359730468174412, -18.69795900347392248 ) ) ;
#28410=EDGE_CURVE ( 'NONE', #24264, #29043, #11299, .T. ) ;
#28416=CARTESIAN_POINT ( 'NONE',  ( 12.02685106364323531, 9.321538569219327997, -16.69182734290254899 ) ) ;
#28418=CARTESIAN_POINT ( 'NONE',  ( 33.33926371295168423, -12.28475995124076903, -19.67523791759492013 ) ) ;
#28420=CARTESIAN_POINT ( 'NONE',  ( 8.944584683310379702, 16.95159276115599667, -17.92279151347708677 ) ) ;
#28424=CARTESIAN_POINT ( 'NONE',  ( 21.48529164538665981, 5.106035544247377267, -18.65531623833433628 ) ) ;
#28425=CARTESIAN_POINT ( 'NONE',  ( 12.75119036009696316, 9.912382880115339745, -16.17456125963731850 ) ) ;
#28428=CARTESIAN_POINT ( 'NONE',  ( 11.46775782571576130, 9.292755756535285627, -15.86302895122203616 ) ) ;
#28430=CARTESIAN_POINT ( 'NONE',  ( 10.43540724046455992, 14.02724713458965233, -16.28994223329847202 ) ) ;
#28435=CARTESIAN_POINT ( 'NONE',  ( 10.36430886937160167, 16.94616899698690204, -17.73806594831300032 ) ) ;
#28437=CARTESIAN_POINT ( 'NONE',  ( 36.54859390953724585, -22.18451583373416014, -17.78191007148576475 ) ) ;
#28438=CARTESIAN_POINT ( 'NONE',  ( 13.75440121443578079, 9.907639265912045801, -15.40915901261088905 ) ) ;
#28439=CARTESIAN_POINT ( 'NONE',  ( 25.97851742199650005, -11.98992670343847244, -16.97112261376066655 ) ) ;
#28445=CARTESIAN_POINT ( 'NONE',  ( 18.58892183794801056, 4.077935791202882854, -15.09018232067737841 ) ) ;
#28446=CARTESIAN_POINT ( 'NONE',  ( 25.52642221012979462, -9.988304178644780151, -15.98026830291908773 ) ) ;
#28459=CARTESIAN_POINT ( 'NONE',  ( 12.27631119714397201, 9.497383584800669354, -15.31093738554958428 ) ) ;
#28464=CARTESIAN_POINT ( 'NONE',  ( 11.46775782571576130, 9.292755756535285627, -15.86302895122203616 ) ) ;
#28467=CARTESIAN_POINT ( 'NONE',  ( 19.45720675144774603, -0.6714082060231494342, -20.03460252700725519 ) ) ;
#28473=CARTESIAN_POINT ( 'NONE',  ( 11.28421916535349112, 16.64009977454265865, -16.78120545242191142 ) ) ;
#28475=CARTESIAN_POINT ( 'NONE',  ( 33.59450136257035524, -12.41883169790769692, -18.71738141962731561 ) ) ;
#28476=CARTESIAN_POINT ( 'NONE',  ( 18.47369133221681281, 7.987600538477567014, -15.27093437040897861 ) ) ;
#28480=CARTESIAN_POINT ( 'NONE',  ( 9.116630548627156827, 16.16256849206635238, -17.05302909012592494 ) ) ;
#28481=CARTESIAN_POINT ( 'NONE',  ( 28.41550859958678643, -4.728095322062062067, -17.81194336819277524 ) ) ;
#28484=CARTESIAN_POINT ( 'NONE',  ( 18.39996379557756256, 0.6904185378075045065, -15.43317298867526866 ) ) ;
#28485=CARTESIAN_POINT ( 'NONE',  ( 15.41580380672748163, 5.935325531760808460, -16.22756139702874023 ) ) ;
#28500=CARTESIAN_POINT ( 'NONE',  ( 9.649959050778257108, 17.62941265384766254, -17.56860460898032628 ) ) ;
#28501=CARTESIAN_POINT ( 'NONE',  ( 26.72351632055398696, -11.69804524575189397, -15.34103589027250791 ) ) ;
#28502=CARTESIAN_POINT ( 'NONE',  ( 22.90957683611224738, 2.308586283387667581, -16.61139769879808625 ) ) ;
#28503=CARTESIAN_POINT ( 'NONE',  ( 35.05385823632300912, -20.96193052275466329, -21.15110683048779805 ) ) ;
#28506=CARTESIAN_POINT ( 'NONE',  ( 15.61762486822808604, 9.948436389806387226, -12.64537296286936829 ) ) ;
#28509=CARTESIAN_POINT ( 'NONE',  ( 16.57956996521092918, 4.788269978297743812, -19.71382457362092566 ) ) ;
#28512=CARTESIAN_POINT ( 'NONE',  ( 10.33841720888800531, 18.38481243897025053, -17.83974501271621449 ) ) ;
#28515=CARTESIAN_POINT ( 'NONE',  ( 19.52227536296714305, 7.868296793410291201, -18.00468392081665669 ) ) ;
#28517=CARTESIAN_POINT ( 'NONE',  ( 28.46611200899306127, -11.40119892829609327, -11.67154496650716666 ) ) ;
#28519=CARTESIAN_POINT ( 'NONE',  ( 35.03938282813840743, -19.89690018161999419, -20.20402626681843117 ) ) ;
#28520=CARTESIAN_POINT ( 'NONE',  ( 21.68595642006795288, -3.720678421232956445, -15.48850127590278980 ) ) ;
#28521=CARTESIAN_POINT ( 'NONE',  ( 19.13053735399196142, -0.4946192386601480084, -18.78456443592403602 ) ) ;
#28523=CARTESIAN_POINT ( 'NONE',  ( 26.51887141003594195, -6.641914482010843557, -12.47546034222045819 ) ) ;
#28533=CARTESIAN_POINT ( 'NONE',  ( 35.28777801271252912, -15.52033788203570985, -19.16652784865743442 ) ) ;
#28534=CARTESIAN_POINT ( 'NONE',  ( 12.75811015101040446, 7.626735917299793499, -14.92445666636202617 ) ) ;
#28537=CARTESIAN_POINT ( 'NONE',  ( 12.26413032053702779, 8.815164712426300397, -16.54932944099246228 ) ) ;
#28545=CARTESIAN_POINT ( 'NONE',  ( 11.22494245711612848, 9.086454032755447940, -17.24116976563960435 ) ) ;
#28547=CARTESIAN_POINT ( 'NONE',  ( 23.18962843369624949, -6.128656054388458507, -17.19981796389819095 ) ) ;
#28548=CARTESIAN_POINT ( 'NONE',  ( 23.72517123929712213, -5.798560033841243744, -19.46542475990168342 ) ) ;
#28560=CARTESIAN_POINT ( 'NONE',  ( 10.47262648896379922, 16.44941058625191133, -17.33455387760982447 ) ) ;
#28564=CARTESIAN_POINT ( 'NONE',  ( 13.37514969516658070, 7.623989538026159529, -15.71142857098959489 ) ) ;
#28567=CARTESIAN_POINT ( 'NONE',  ( 20.99533150354982070, 4.487273811465053441, -19.54336078777620500 ) ) ;
#28568=CARTESIAN_POINT ( 'NONE',  ( 12.86616790684404421, 9.515247448762703897, -16.11708638872277177 ) ) ;
#28572=CARTESIAN_POINT ( 'NONE',  ( 9.997747326010761881, 16.03441129093729245, -16.47093000352221637 ) ) ;
#28574=CARTESIAN_POINT ( 'NONE',  ( 9.916824447075894611, 16.40553392900050156, -16.50439446175997205 ) ) ;
#28579=CARTESIAN_POINT ( 'NONE',  ( 13.11546866977305825, 8.567317423965196355, -15.91839467484043880 ) ) ;
#28582=CARTESIAN_POINT ( 'NONE',  ( 33.60507142094932931, -10.68002793468083134, -20.32431474444524255 ) ) ;
#28583=CARTESIAN_POINT ( 'NONE',  ( 16.78426473046523526, 10.16049046829612479, -19.50779498702920378 ) ) ;
#28584=CARTESIAN_POINT ( 'NONE',  ( 29.62588713853392264, -10.65184931322849060, -12.76488833982454629 ) ) ;
#28592=CARTESIAN_POINT ( 'NONE',  ( 18.08386662754633534, 1.890959213400748684, -17.98613275626550134 ) ) ;
#28594=CARTESIAN_POINT ( 'NONE',  ( 28.49100808714443289, -10.93160309251996765, -13.65156567797833631 ) ) ;
#28602=CARTESIAN_POINT ( 'NONE',  ( 12.27690927615027583, 9.494639109526119114, -15.31069018153633721 ) ) ;
#28607=CARTESIAN_POINT ( 'NONE',  ( 12.47535353872619446, 8.560407331872438519, -15.14977315560688176 ) ) ;
#28609=CARTESIAN_POINT ( 'NONE',  ( 18.31109272121128484, -1.763409964857557188, -18.37077502410619090 ) ) ;
#28615=CARTESIAN_POINT ( 'NONE',  ( 12.84801357566967717, 9.517348710814296453, -16.13078356789775469 ) ) ;
#28619=CARTESIAN_POINT ( 'NONE',  ( 35.54686456755326418, -21.17674681625933530, -18.46270299499373735 ) ) ;
#28620=CARTESIAN_POINT ( 'NONE',  ( 15.44629794785920218, 3.545610805586186132, -16.71614555938632307 ) ) ;
#28624=CARTESIAN_POINT ( 'NONE',  ( 27.18523481531828168, -13.05407500640787077, -12.66260957699712186 ) ) ;
#28627=CARTESIAN_POINT ( 'NONE',  ( 24.00718893345771932, -1.002666751694005765, -18.91818096615087796 ) ) ;
#28628=CARTESIAN_POINT ( 'NONE',  ( 18.26355027798676645, 7.143056880744947712, -15.77244846760033958 ) ) ;
#28643=CARTESIAN_POINT ( 'NONE',  ( 11.47304865262203499, 9.268493388164605662, -15.86084085272616484 ) ) ;
#28644=CARTESIAN_POINT ( 'NONE',  ( 26.45169718342334164, -9.008644514675534509, -18.11399877363951205 ) ) ;
#28645=CARTESIAN_POINT ( 'NONE',  ( 21.00058363250239069, -3.857595149258782996, -18.17417979037076847 ) ) ;
#28647=CARTESIAN_POINT ( 'NONE',  ( 32.36240160181304759, -11.00785621467150044, -17.57054915585148436 ) ) ;
#28656=CARTESIAN_POINT ( 'NONE',  ( 19.07848178107829540, -2.338951347401693859, -17.85627120065723616 ) ) ;
#28659=CARTESIAN_POINT ( 'NONE',  ( 10.72091424521701519, 16.63063227333373462, -15.95414859203816782 ) ) ;
#28664=CARTESIAN_POINT ( 'NONE',  ( 19.07848178107829540, -2.338951347401693859, -17.85627120065723616 ) ) ;
#28667=CARTESIAN_POINT ( 'NONE',  ( 14.35528768574272895, 10.45889919667044410, -14.17515447063821910 ) ) ;
#28669=CARTESIAN_POINT ( 'NONE',  ( 33.17819505895439391, -11.78846528140086924, -19.49437495119144259 ) ) ;
#28671=CARTESIAN_POINT ( 'NONE',  ( 28.52362724998032917, -7.841767518281756111, -12.14325827080317666 ) ) ;
#28672=CARTESIAN_POINT ( 'NONE',  ( 18.53362878050275597, 1.800236982614616510, -15.18126852959267481 ) ) ;
#28682=CARTESIAN_POINT ( 'NONE',  ( 36.54859390953724585, -22.18451583373416014, -18.19919658220850778 ) ) ;
#28683=CARTESIAN_POINT ( 'NONE',  ( 9.641350810849047548, 17.66889113945805789, -17.91664992932186351 ) ) ;
#28686=CARTESIAN_POINT ( 'NONE',  ( 12.02406503409520333, 9.334315655862766903, -16.69297946412503819 ) ) ;
#28702=CARTESIAN_POINT ( 'NONE',  ( 11.40026617402801179, 8.559985368287675200, -17.14749594687102174 ) ) ;
#28704=CARTESIAN_POINT ( 'NONE',  ( 24.36960067559809318, -5.041758482997499513, -18.26785210147486538 ) ) ;
#28705=CARTESIAN_POINT ( 'NONE',  ( 21.00058363250239069, -3.857595149258782996, -18.17417979037076847 ) ) ;
#28715=CARTESIAN_POINT ( 'NONE',  ( 12.02558468657594659, 9.327346335875439820, -16.69235103436730938 ) ) ;
#28717=CARTESIAN_POINT ( 'NONE',  ( 33.76744293605320024, -13.18274801178271005, -18.77722780292321758 ) ) ;
#28720=CARTESIAN_POINT ( 'NONE',  ( 17.72817910449685996, 9.547663288818908356, -12.24198789229035533 ) ) ;
#28722=CARTESIAN_POINT ( 'NONE',  ( 22.34083945069921739, -4.755659482961629436, -14.12236044035638116 ) ) ;
#28723=CARTESIAN_POINT ( 'NONE',  ( 12.84461350077944886, 9.519659821018855439, -16.13320262440205966 ) ) ;
#28730=CARTESIAN_POINT ( 'NONE',  ( 11.48249212886396897, 9.228508165798535501, -15.85668214399537845 ) ) ;
#28732=CARTESIAN_POINT ( 'NONE',  ( 9.949118446627077006, 16.25742953053141804, -16.49103975576934644 ) ) ;
#28735=ADVANCED_FACE ( 'NONE', ( #21505 ), #17879, .F. ) ;
#28739=CARTESIAN_POINT ( 'NONE',  ( 12.22285885739602662, 8.868278133530205665, -16.57678160000113721 ) ) ;
#28741=CARTESIAN_POINT ( 'NONE',  ( 36.54859390953724585, -23.18451583373416014, -16.11276402859391510 ) ) ;
#28742=CARTESIAN_POINT ( 'NONE',  ( 26.92971693216691165, -8.617903733377630715, -13.36642543767191427 ) ) ;
#28743=CARTESIAN_POINT ( 'NONE',  ( 30.24922550192677306, -10.40856591028444278, -13.02298783260255988 ) ) ;
#28744=ORIENTED_EDGE ( 'NONE', *, *, #9238, .F. ) ;
#28749=CARTESIAN_POINT ( 'NONE',  ( 36.12281451779777797, -20.27171456826661355, -20.44288436412734100 ) ) ;
#28753=CARTESIAN_POINT ( 'NONE',  ( 20.29079399015155616, 4.720006093641750944, -15.95989367155712202 ) ) ;
#28755=CARTESIAN_POINT ( 'NONE',  ( 19.25048709941964376, 7.441878894999256921, -18.84525011105569803 ) ) ;
#28766=CARTESIAN_POINT ( 'NONE',  ( 12.27664511671607883, 9.495749246718952818, -15.31080714918738295 ) ) ;
#28771=CARTESIAN_POINT ( 'NONE',  ( 12.51417009928267099, 8.576964204390579383, -15.11888119342340353 ) ) ;
#28773=CARTESIAN_POINT ( 'NONE',  ( 18.63699955181457923, 5.162464354397502397, -14.86688106074863569 ) ) ;
#28781=CARTESIAN_POINT ( 'NONE',  ( 12.83122539074939894, 9.545332027449857648, -16.14146395906381670 ) ) ;
#28783=CARTESIAN_POINT ( 'NONE',  ( 36.41702210941816986, -20.59343343131470050, -19.35259392719279603 ) ) ;
#28784=CARTESIAN_POINT ( 'NONE',  ( 16.34386185847872142, 4.569898679961749366, -19.52586945278800812 ) ) ;
#28786=CARTESIAN_POINT ( 'NONE',  ( 25.74126694659371495, -13.30326880535473322, -17.45270501867052104 ) ) ;
#28789=CARTESIAN_POINT ( 'NONE',  ( 26.20148740379470453, -2.166401353139026487, -14.75472287570676322 ) ) ;
#28790=CARTESIAN_POINT ( 'NONE',  ( 19.07173961884560498, -1.856618079973750390, -13.92706601484911033 ) ) ;
#28807=CARTESIAN_POINT ( 'NONE',  ( 11.47079713067724782, 9.278817116560638567, -15.86177209170659275 ) ) ;
#28808=CARTESIAN_POINT ( 'NONE',  ( 27.00739300205740889, -11.59555048707680847, -14.72185353022491050 ) ) ;
#28809=CARTESIAN_POINT ( 'NONE',  ( 25.01196530022370368, -10.21768535905550124, -13.66937216179565517 ) ) ;
#28810=CARTESIAN_POINT ( 'NONE',  ( 35.54317590287104167, -23.16017559978188345, -18.72806989825276247 ) ) ;
#28818=CARTESIAN_POINT ( 'NONE',  ( 17.18819971663578272, 0.8441372818425427749, -18.45219435416397502 ) ) ;
#28821=CARTESIAN_POINT ( 'NONE',  ( 11.75823633891744535, 11.87334092381181883, -15.52517956378672359 ) ) ;
#28825=CARTESIAN_POINT ( 'NONE',  ( 20.72626264887238534, -1.914771856900582714, -13.62749948506543518 ) ) ;
#28826=CARTESIAN_POINT ( 'NONE',  ( 16.77192278198516107, 3.819237988068143075, -20.73389043596634806 ) ) ;
#28828=CARTESIAN_POINT ( 'NONE',  ( 33.75544676243647757, -14.12885555826641593, -19.81592319558764004 ) ) ;
#28829=CARTESIAN_POINT ( 'NONE',  ( 24.76964776845370864, -3.801875552749832909, -18.97459646659829247 ) ) ;
#28830=CARTESIAN_POINT ( 'NONE',  ( 19.18059203083059217, 2.087369379035357575, -14.72322290489779917 ) ) ;
#28831=CARTESIAN_POINT ( 'NONE',  ( 26.72358035960067824, -3.685970424986596772, -17.59444040205794835 ) ) ;
#28845=CARTESIAN_POINT ( 'NONE',  ( 18.68520274485960542, 10.62608585526774441, -17.78552708330943588 ) ) ;
#28846=CARTESIAN_POINT ( 'NONE',  ( 33.40535544545146251, -10.40465400369240356, -18.27852168438239389 ) ) ;
#28847=CARTESIAN_POINT ( 'NONE',  ( 9.916637298967875935, 16.40639221407973380, -16.50447193873893781 ) ) ;
#28850=CARTESIAN_POINT ( 'NONE',  ( 13.12216094266758581, 8.570213704404382682, -15.91306547940487448 ) ) ;
#28863=CARTESIAN_POINT ( 'NONE',  ( 11.22367979475099631, 9.092227732665495665, -17.24169321984975056 ) ) ;
#28865=CARTESIAN_POINT ( 'NONE',  ( 29.49229018507869071, -8.391778287988243434, -19.20830874944899236 ) ) ;
#28866=CARTESIAN_POINT ( 'NONE',  ( 22.34648740292275093, -2.602002351270185532, -19.46322174391540116 ) ) ;
#28882=CARTESIAN_POINT ( 'NONE',  ( 13.12425544150138279, 8.571136816377206813, -15.91139631635614471 ) ) ;
#28883=CARTESIAN_POINT ( 'NONE',  ( 33.64261581855389949, -12.62196589562294591, -18.73949555988700055 ) ) ;
#28885=CARTESIAN_POINT ( 'NONE',  ( 9.115110896146415342, 16.16953781205366170, -17.05365751988364309 ) ) ;
#28887=CARTESIAN_POINT ( 'NONE',  ( 24.18219217278060995, -6.970120066757704791, -14.18070892486464629 ) ) ;
#28888=CARTESIAN_POINT ( 'NONE',  ( 12.83097211533594439, 9.546493580781078236, -16.14156869735677446 ) ) ;
#28893=CARTESIAN_POINT ( 'NONE',  ( 11.47219014545126647, 9.272428573238919114, -15.86119603109536058 ) ) ;
#28898=CARTESIAN_POINT ( 'NONE',  ( 11.94706930840425407, 9.687427868553587729, -16.72481990518296158 ) ) ;
#28900=CARTESIAN_POINT ( 'NONE',  ( 14.77169846916584461, 3.272981165966227568, -18.54959716842853723 ) ) ;
#28901=CARTESIAN_POINT ( 'NONE',  ( 27.76312469413510442, -10.32446017237915648, -18.80420148706337358 ) ) ;
#28904=CARTESIAN_POINT ( 'NONE',  ( 36.09161981528372110, -20.13157329416283048, -20.44814669990763889 ) ) ;
#28907=CARTESIAN_POINT ( 'NONE',  ( 17.99585798733817299, 1.806717527199089401, -17.78491074480216838 ) ) ;
#28908=CARTESIAN_POINT ( 'NONE',  ( 21.58242789233717573, 5.264303332692052528, -18.32037006577847293 ) ) ;
#28915=DIRECTION ( 'NONE',  ( -1.000000000000000000, 0.000000000000000000, 0.000000000000000000 ) ) ;
#28918=CARTESIAN_POINT ( 'NONE',  ( 11.62855932722735908, 12.46805622939721836, -15.57880556977976916 ) ) ;
#28922=CARTESIAN_POINT ( 'NONE',  ( 12.56861602585598980, 8.601024833420110483, -15.07548682890769243 ) ) ;
#28924=CARTESIAN_POINT ( 'NONE',  ( 10.67817636951947868, 9.002809132723193386, -16.40714615800424880 ) ) ;
#28930=CARTESIAN_POINT ( 'NONE',  ( 12.83160530386958342, 9.543589697453029430, -16.14130685162439249 ) ) ;
#28932=CARTESIAN_POINT ( 'NONE',  ( 33.98852084862024725, -11.13792163938717472, -17.92802646347312034 ) ) ;
#28933=CARTESIAN_POINT ( 'NONE',  ( 19.52227536296714305, 7.868296793410291201, -18.00468392081665669 ) ) ;
#28937=CARTESIAN_POINT ( 'NONE',  ( 32.15747877504752950, -11.00374777879112642, -13.30332049327740052 ) ) ;
#28941=CARTESIAN_POINT ( 'NONE',  ( 23.74924978780510898, -3.048960050427876656, -13.27477993493952191 ) ) ;
#28942=CARTESIAN_POINT ( 'NONE',  ( 20.14260469057294500, 4.737385465944226048, -19.07682320266127718 ) ) ;
#28953=CARTESIAN_POINT ( 'NONE',  ( 11.51951884677450266, 9.108496074915260365, -15.83757232928968683 ) ) ;
#28954=CARTESIAN_POINT ( 'NONE',  ( 28.35258904315412920, -6.370284285516064848, -14.91745349193007364 ) ) ;
#28955=CARTESIAN_POINT ( 'NONE',  ( 24.16496757332932788, -10.42823604606268617, -16.34834267607407909 ) ) ;
#28963=CARTESIAN_POINT ( 'NONE',  ( 19.68115760211910725, 3.144890361740488860, -20.29587546762095940 ) ) ;
#28967=CARTESIAN_POINT ( 'NONE',  ( 12.27593128402378753, 9.499125914797495795, -15.31109449298900671 ) ) ;
#28969=CARTESIAN_POINT ( 'NONE',  ( 33.27037009343090546, -12.05169513820189309, -19.60996450177851713 ) ) ;
#28971=CARTESIAN_POINT ( 'NONE',  ( 24.00918528248616468, -0.5066965781341161712, -13.81223085940890627 ) ) ;
#28973=CARTESIAN_POINT ( 'NONE',  ( 22.45977841265724351, 4.097634946112983734, -18.47195213137534964 ) ) ;
#28978=CARTESIAN_POINT ( 'NONE',  ( 31.14759003376246582, -7.259970019232452998, -15.53234487094253069 ) ) ;
#28980=CARTESIAN_POINT ( 'NONE',  ( 23.73516035876120611, -6.831976609072074602, -19.85773546425274105 ) ) ;
#28983=CARTESIAN_POINT ( 'NONE',  ( 30.24922550192677306, -10.40856591028444278, -13.02298783260255988 ) ) ;
#28988=CARTESIAN_POINT ( 'NONE',  ( 36.04209255463945993, -19.90907354740926394, -20.43687144983462289 ) ) ;
#28989=CARTESIAN_POINT ( 'NONE',  ( 11.34314632229486364, 9.864239995495806212, -15.91456019135469013 ) ) ;
#28993=CARTESIAN_POINT ( 'NONE',  ( 9.661883355341293722, 16.25482528653935077, -17.91547504436015004 ) ) ;
#29003=CARTESIAN_POINT ( 'NONE',  ( 13.32639783386816212, 7.603689066773378968, -15.75018979827038912 ) ) ;
#29005=CARTESIAN_POINT ( 'NONE',  ( 13.18850634723077242, 6.203946520731500769, -19.20132247218941401 ) ) ;
#29007=CARTESIAN_POINT ( 'NONE',  ( 25.01196530022370368, -10.21768535905550124, -13.66937216179565517 ) ) ;
#29020=CARTESIAN_POINT ( 'NONE',  ( 13.01452397926061089, 8.532813591658360508, -15.99807864679971026 ) ) ;
#29021=CARTESIAN_POINT ( 'NONE',  ( 35.49237112349044310, -21.93193663806729887, -19.32748734164077931 ) ) ;
#29023=CARTESIAN_POINT ( 'NONE',  ( 8.949836677108400806, 16.92750644812532457, -17.70396109330303958 ) ) ;
#29024=CARTESIAN_POINT ( 'NONE',  ( 22.16846437878366061, -4.107540447007581363, -19.06500358040360865 ) ) ;
#29025=CARTESIAN_POINT ( 'NONE',  ( 12.83160530386958342, 9.543589697453029430, -16.14130685162439249 ) ) ;
#29031=CARTESIAN_POINT ( 'NONE',  ( 11.97192087863669663, 8.579774655713777065, -15.53257280409644991 ) ) ;
#29036=CARTESIAN_POINT ( 'NONE',  ( 12.02406503409520333, 9.334315655862766903, -16.69297946412503819 ) ) ;
#29038=CARTESIAN_POINT ( 'NONE',  ( 15.46132241025727083, 3.192341012408233869, -14.38206433644783111 ) ) ;
#29039=CARTESIAN_POINT ( 'NONE',  ( 17.73099166324444553, -0.3602181158183791476, -14.74723639357852178 ) ) ;
#29043=VERTEX_POINT ( 'NONE', #27634 ) ;
#29046=CARTESIAN_POINT ( 'NONE',  ( 35.88208498122789791, -19.19024427843809733, -20.38849413606966010 ) ) ;
#29048=CARTESIAN_POINT ( 'NONE',  ( 20.14628369065288993, 2.528829491441240584, -14.55248280469624866 ) ) ;
#29049=CARTESIAN_POINT ( 'NONE',  ( 21.64656857049893901, 5.639188926465734220, -17.17864421186117951 ) ) ;
#29058=CARTESIAN_POINT ( 'NONE',  ( 10.98017426877725811, 15.44163275732038443, -15.84693559973663035 ) ) ;
#29065=CARTESIAN_POINT ( 'NONE',  ( 11.58682163191119230, 8.958038730125363003, -15.79767441425272345 ) ) ;
#29067=CARTESIAN_POINT ( 'NONE',  ( 10.66961851098191083, 9.040384230280389843, -16.41081268017797257 ) ) ;
#29072=CARTESIAN_POINT ( 'NONE',  ( 12.83519646890166577, 9.531778640408997916, -16.13946648208032641 ) ) ;
#29075=CARTESIAN_POINT ( 'NONE',  ( 36.00107582698698394, -18.72480711723410352, -19.38214066600889751 ) ) ;
#29076=CARTESIAN_POINT ( 'NONE',  ( 21.48529164538665981, 5.106035544247377267, -18.65531623833433628 ) ) ;
#29082=CARTESIAN_POINT ( 'NONE',  ( 30.28288205714520132, -11.65814127372701670, -12.00898047443557459 ) ) ;
#29088=CARTESIAN_POINT ( 'NONE',  ( 22.16683763302808430, -0.5050174593055701822, -13.96310542101677044 ) ) ;
#29089=CARTESIAN_POINT ( 'NONE',  ( 22.85609869791697335, 3.752015377681134467, -15.55886478590537969 ) ) ;
#29099=CARTESIAN_POINT ( 'NONE',  ( 11.39177520167864266, 9.641221755901229429, -15.89445043910815336 ) ) ;
#29100=CARTESIAN_POINT ( 'NONE',  ( 14.18486973814142793, 6.324582201221724098, -17.68508340245422872 ) ) ;
#29101=CARTESIAN_POINT ( 'NONE',  ( 28.92999000670439713, -5.550862855971650411, -17.57004703619191943 ) ) ;
#29110=CARTESIAN_POINT ( 'NONE',  ( 23.86551563699305234, 2.542095107771292106, -17.79649620197707094 ) ) ;
#29113=CARTESIAN_POINT ( 'NONE',  ( 12.27584558688950978, 9.498490731067679604, -15.31120835137462244 ) ) ;
#29114=CARTESIAN_POINT ( 'NONE',  ( 31.63980255171021483, -10.89810845426378982, -15.52824638758754183 ) ) ;
#29117=CARTESIAN_POINT ( 'NONE',  ( 17.55424633453837302, 0.6138019359854992585, -14.89346452969079060 ) ) ;
#29119=CARTESIAN_POINT ( 'NONE',  ( 18.14419664895403272, 7.915595134365798202, -13.41836860846829538 ) ) ;
#29123=CARTESIAN_POINT ( 'NONE',  ( 23.31581686446907398, -5.989474659622321617, -13.63887547363156827 ) ) ;
#29125=CARTESIAN_POINT ( 'NONE',  ( 23.96443177966278881, -0.8440764653970969089, -20.02211457469898548 ) ) ;
#29127=CARTESIAN_POINT ( 'NONE',  ( 28.75197783424699693, -9.407057218516385433, -18.70835418409691542 ) ) ;
#29134=CARTESIAN_POINT ( 'NONE',  ( 13.76974871631934860, 5.358497188706473402, -17.46738557873778674 ) ) ;
#29136=CARTESIAN_POINT ( 'NONE',  ( 34.52681913409613657, -13.10175273156466069, -19.97882978310374469 ) ) ;
#29138=CARTESIAN_POINT ( 'NONE',  ( 11.44040408106239326, 9.418203516307107392, -15.87434068686103394 ) ) ;
#29141=CARTESIAN_POINT ( 'NONE',  ( 14.03260640326807085, 7.914523595725262872, -15.18742456645827588 ) ) ;
#29142=CARTESIAN_POINT ( 'NONE',  ( 13.12362514754451759, 8.570858352459396201, -15.91189866610160841 ) ) ;
#29152=CARTESIAN_POINT ( 'NONE',  ( 8.944584812045984989, 16.95159217075808655, -17.91472939532503261 ) ) ;
#29153=CARTESIAN_POINT ( 'NONE',  ( 18.07402036735202699, 11.65617268414930940, -17.08825885362000108 ) ) ;
#29154=CARTESIAN_POINT ( 'NONE',  ( 25.71810023473615203, -5.953606672203104466, -12.71518937071605038 ) ) ;
#29166=CARTESIAN_POINT ( 'NONE',  ( 13.09695832212169364, 8.559710067821024282, -15.93310406974445392 ) ) ;
#29169=CARTESIAN_POINT ( 'NONE',  ( 33.66936448658974257, -12.74213349194280553, -18.74758104053764995 ) ) ;
#29172=CARTESIAN_POINT ( 'NONE',  ( 9.177416647856844634, 15.88379569257361190, -17.02789189981719176 ) ) ;
#29177=CARTESIAN_POINT ( 'NONE',  ( 22.09544204423535874, -4.864148257255451746, -14.35781331922719772 ) ) ;
#29178=CARTESIAN_POINT ( 'NONE',  ( 10.35867142355733783, 16.97202304209818990, -17.90451223021000260 ) ) ;
#29184=CARTESIAN_POINT ( 'NONE',  ( 12.49271550807400999, 8.567542729147559655, -15.13597632865050535 ) ) ;
#29189=CARTESIAN_POINT ( 'NONE',  ( 12.03206445085756116, 9.298183410334813104, -16.68962916345529024 ) ) ;
#29191=CARTESIAN_POINT ( 'NONE',  ( 18.26434493437671946, 4.448125397982363616, -12.89349226661579273 ) ) ;
#29192=CARTESIAN_POINT ( 'NONE',  ( 15.46132241025727083, 3.192341012408233869, -14.38206433644783111 ) ) ;
#29196=CARTESIAN_POINT ( 'NONE',  ( 36.21530066971708095, -20.68720585756345187, -20.37220581101806971 ) ) ;
#29197=CARTESIAN_POINT ( 'NONE',  ( 14.18486973814142793, 6.324582201221724098, -17.68508340245422872 ) ) ;
#29211=CARTESIAN_POINT ( 'NONE',  ( 11.05541531668977662, 17.68942339022145305, -21.33333333332589632 ) ) ;
#29215=CARTESIAN_POINT ( 'NONE',  ( 12.50481220565295004, 8.572828783776230921, -15.12633959982445653 ) ) ;
#29218=CARTESIAN_POINT ( 'NONE',  ( 10.66806909375856627, 9.047473561677174203, -16.41145467664113156 ) ) ;
#29225=CARTESIAN_POINT ( 'NONE',  ( 12.82717298413408358, 9.563916880749394167, -16.14313977175105919 ) ) ;
#29227=CARTESIAN_POINT ( 'NONE',  ( 34.61906131182126245, -12.51614797404085877, -18.96439083239160439 ) ) ;
#29228=CARTESIAN_POINT ( 'NONE',  ( 19.07848178107829540, -2.338951347401693859, -17.85627120065723616 ) ) ;
#29233=CARTESIAN_POINT ( 'NONE',  ( 13.15390973649967599, 8.859676595473322536, -14.60899741038990562 ) ) ;
#29237=CARTESIAN_POINT ( 'NONE',  ( 22.28231863826031756, 1.183864898644814811, -18.90614694914491167 ) ) ;
#29238=CARTESIAN_POINT ( 'NONE',  ( 18.31109272121128484, -1.763409964857557188, -18.37077502410619090 ) ) ;
#29251=CARTESIAN_POINT ( 'NONE',  ( 11.21893088074867073, 9.114006857625895464, -17.24365706284262600 ) ) ;
#29254=B_SPLINE_CURVE_WITH_KNOTS ( 'NONE', 3,
 ( #16251, #396, #2241, #11513, #11967, #18703, #21286, #14104, #23746, #23283, #13804, #4965, #7104, #25729, #19005, #23132, #23586, #4515, #16561, #555, #28208, #28363, #4658, #248, #18847, #2843, #4810, #7418, #2395, #16718, #23438, #9681, #5114, #12129, #20828, #27905, #2550, #11821, #11669, #14406, #21443, #9839, #21138, #9524, #16861, #7262, #25887, #14255, #19152, #30211, #9220, #28509, #7558, #18548, #20984, #25564, #9376, #21893, #17308, #26805, #19449, #7856, #7709, #12876, #845, #10135, #24494, #26192, #12729, #3002, #5271, #24052, #21597, #22050, #19595, #12279, #1152, #695, #10432, #28963, #17018, #22190, #29266, #10286, #19741, #26341, #28818, #1008, #14710, #5424, #17164, #5878, #8300, #7999, #3436, #15158, #10589, #5575, #3152, #24340, #19298, #23905, #9983, #29110, #26494, #8150, #14856, #3586, #12425, #14558, #26647, #24197, #3299, #17457, #28656, #15009, #21743, #5727, #1299, #19897, #12574, #17754, #13328, #1752, #6619, #10884, #1909, #6172, #20497, #17894, #25089, #8892, #15911, #3734, #10746, #27274, #24953, #15465, #11188, #4179, #27565, #6324, #15620, #30025, #20343, #11042, #29733, #8741, #17607, #13032, #4034, #8595, #29883, #27111, #18058, #3886, #22652, #27421, #18206, #20195, #29579, #29428, #4328, #22508, #15306, #25241, #13625, #1609, #20054, #22956, #24796, #2057, #6475, #15765, #13473, #13184, #22804, #11336, #22349, #20641, #26963, #6023, #8448, #24639, #1455, #9034, #9648, #2516, #14368, #11477, #6771, #7227, #23248, #25850, #18669, #28324, #18512, #18357, #9489, #2361, #58, #18813, #2204, #23704, #23551, #20793, #4779, #23399, #2654, #9186, #14069, #11784, #7382, #11632, #11929, #27872, #21251, #9342, #16525, #363, #16677, #28170, #23101, #26000, #20946, #6927, #4626, #13773, #4929, #28014, #7073, #21407, #21104, #210, #14221, #18967, #27714, #25391, #16368, #25689, #5076, #2807, #12090, #16220, #25534, #13918 ),
 .UNSPECIFIED., .F., .F.,
 ( 4, 2, 2, 2, 2, 2, 2, 2, 2, 2, 2, 2, 2, 2, 2, 2, 2, 2, 2, 2, 2, 2, 2, 2, 2, 2, 2, 2, 2, 2, 2, 2, 2, 2, 2, 2, 2, 2, 2, 2, 2, 2, 2, 2, 2, 2, 2, 2, 2, 2, 2, 2, 2, 2, 2, 2, 2, 2, 2, 2, 2, 2, 2, 2, 2, 2, 2, 2, 2, 2, 2, 2, 2, 2, 2, 2, 2, 2, 2, 2, 2, 2, 2, 2, 2, 2, 2, 2, 2, 2, 2, 2, 2, 2, 2, 2, 2, 2, 2, 2, 2, 2, 2, 2, 2, 2, 2, 2, 2, 2, 2, 2, 2, 2, 2, 2, 2, 2, 2, 2, 2, 2, 4 ),
 ( 0.000000000000000000, 0.007812500000000000000, 0.01464843750000000000, 0.02148437500000000000, 0.02832031250000000000, 0.03515625000000000000, 0.04882812500000000000, 0.05566406250000000000, 0.06250000000000000000, 0.06933593750000000000, 0.07617187500000000000, 0.08984375000000000000, 0.09667968750000000000, 0.1035156250000000000, 0.1103515625000000000, 0.1171875000000000000, 0.1240234375000000000, 0.1308593750000000000, 0.1376953125000000000, 0.1445312500000000000, 0.1513671875000000000, 0.1582031250000000000, 0.1718750000000000000, 0.1787109375000000000, 0.1855468750000000000, 0.1992187500000000000, 0.2060546875000000000, 0.2128906250000000000, 0.2197265625000000000, 0.2265625000000000000, 0.2402343750000000000, 0.2470703125000000000, 0.2539062500000000000, 0.2607421875000000000, 0.2675781250000000000, 0.2812500000000000000, 0.2880859375000000000, 0.2949218750000000000, 0.3017578125000000000, 0.3085937500000000000, 0.3154296875000000000, 0.3222656250000000000, 0.3291015625000000000, 0.3359375000000000000, 0.3496093750000000000, 0.3564453125000000000, 0.3632812500000000000, 0.3701171875000000000, 0.3769531250000000000, 0.3906250000000000000, 0.3974609375000000000, 0.4042968750000000000, 0.4179687500000000000, 0.4316406250000000000, 0.4384765625000000000, 0.4453125000000000000, 0.4521484375000000000, 0.4589843750000000000, 0.4658203125000000000, 0.4726562500000000000, 0.4794921875000000000, 0.4863281250000000000, 0.4931640625000000000, 0.5000000000000000000, 0.5078125000000000000, 0.5156250000000000000, 0.5234375000000000000, 0.5312500000000000000, 0.5390625000000000000, 0.5468750000000000000, 0.5625000000000000000, 0.5693359375000000000, 0.5761718750000000000, 0.5898437500000000000, 0.5966796875000000000, 0.6035156250000000000, 0.6103515625000000000, 0.6171875000000000000, 0.6308593750000000000, 0.6376953125000000000, 0.6445312500000000000, 0.6513671875000000000, 0.6582031250000000000, 0.6718750000000000000, 0.6787109375000000000, 0.6855468750000000000, 0.6992187500000000000, 0.7128906250000000000, 0.7197265625000000000, 0.7265625000000000000, 0.7333984375000000000, 0.7402343750000000000, 0.7470703125000000000, 0.7539062500000000000, 0.7607421875000000000, 0.7675781250000000000, 0.7744140625000000000, 0.7812500000000000000, 0.7890625000000000000, 0.7968750000000000000, 0.8046875000000000000, 0.8125000000000000000, 0.8203125000000000000, 0.8281250000000000000, 0.8437500000000000000, 0.8505859375000000000, 0.8574218750000000000, 0.8710937500000000000, 0.8779296875000000000, 0.8847656250000000000, 0.8916015625000000000, 0.8984375000000000000, 0.9121093750000000000, 0.9189453125000000000, 0.9257812500000000000, 0.9326171875000000000, 0.9394531250000000000, 0.9531250000000000000, 0.9589843750000000000, 0.9648437500000000000, 0.9765625000000000000, 0.9882812500000000000, 1.000000000000000000 ),
 .UNSPECIFIED. ) ;
#29255=CARTESIAN_POINT ( 'NONE',  ( 11.47029057985033340, 9.281140223223081520, -15.86198156829250117 ) ) ;
#29258=CARTESIAN_POINT ( 'NONE',  ( 27.15293434934692129, -9.258526923162836653, -12.62629486378885701 ) ) ;
#29266=CARTESIAN_POINT ( 'NONE',  ( 18.50902107916489570, 2.085137940960992697, -20.06823964296112450 ) ) ;
#29269=CARTESIAN_POINT ( 'NONE',  ( 12.27682979692750997, 9.494989133591600350, -15.31072415319233215 ) ) ;
#29272=CARTESIAN_POINT ( 'NONE',  ( 21.42923412144385509, -1.598955984811285536, -13.33006947543598741 ) ) ;
#29274=CARTESIAN_POINT ( 'NONE',  ( 18.57953865233433532, 8.080199298666570940, -13.63460617990120838 ) ) ;
#29276=CARTESIAN_POINT ( 'NONE',  ( 35.54859390953724585, -22.18451583373416014, -16.11276402859391865 ) ) ;
#29278=CARTESIAN_POINT ( 'NONE',  ( 24.62608015258945215, -5.401662417846991637, -13.04198456947205820 ) ) ;
#29279=CARTESIAN_POINT ( 'NONE',  ( 22.90368100322821121, -1.908636692139587199, -20.53213217155426662 ) ) ;
#29294=CARTESIAN_POINT ( 'NONE',  ( 23.95332181684718975, -6.025008234661991757, -14.41687206698971124 ) ) ;
#29296=CARTESIAN_POINT ( 'NONE',  ( 34.15817405333866219, -12.44562566045073204, -20.90971876709214783 ) ) ;
#29299=CARTESIAN_POINT ( 'NONE',  ( 9.919231947839115549, 16.39449282361540483, -16.50339887433786501 ) ) ;
#29304=CARTESIAN_POINT ( 'NONE',  ( 9.661883062155979474, 16.25482663112457971, -17.91578995581314260 ) ) ;
#29307=CARTESIAN_POINT ( 'NONE',  ( 11.47276097331165623, 9.269810413962238371, -15.86095999428340697 ) ) ;
#29314=CARTESIAN_POINT ( 'NONE',  ( 13.38606102883407445, 7.628803627606831839, -15.70273264218319120 ) ) ;
#29315=CARTESIAN_POINT ( 'NONE',  ( 31.50466570323033011, -10.22776944099620877, -17.14799365788790553 ) ) ;
#29318=CARTESIAN_POINT ( 'NONE',  ( 26.55477173981947914, -11.17418396328012342, -19.38009549175560053 ) ) ;
#29320=CARTESIAN_POINT ( 'NONE',  ( 30.02037170576755187, -9.505783518442527225, -18.49971606337314967 ) ) ;
#29335=CARTESIAN_POINT ( 'NONE',  ( 13.12808413666193275, 8.572828783776230921, -15.90834477884588516 ) ) ;
#29337=CARTESIAN_POINT ( 'NONE',  ( 33.30991885831043220, -11.83535627117299960, -18.22721479198959926 ) ) ;
#29340=CARTESIAN_POINT ( 'NONE',  ( 9.760963200462100531, 13.20757681744125911, -16.78657487285272509 ) ) ;
#29342=CARTESIAN_POINT ( 'NONE',  ( 26.85315702054868936, -3.432285194908070380, -17.01323758698984889 ) ) ;
#29343=CARTESIAN_POINT ( 'NONE',  ( 15.98547205987755149, 10.89358938796158149, -13.63095616771664709 ) ) ;
#29350=CARTESIAN_POINT ( 'NONE',  ( 11.47231678315799464, 9.271847796573304379, -15.86114366194887815 ) ) ;
#29355=CARTESIAN_POINT ( 'NONE',  ( 9.661883066202028303, 16.25482661256886630, -17.91573536996246929 ) ) ;
#29357=CARTESIAN_POINT ( 'NONE',  ( 18.01687101988986583, 8.608027666922664523, -14.27462087050975015 ) ) ;
#29358=CARTESIAN_POINT ( 'NONE',  ( 20.85347709306256547, 5.504344946561741558, -13.72608531385973407 ) ) ;
#29361=CARTESIAN_POINT ( 'NONE',  ( 36.54859390953724585, -22.18451583373416014, -18.19919658220850778 ) ) ;
#29366=CARTESIAN_POINT ( 'NONE',  ( 14.73401617531889229, 6.408058468588501810, -15.60580005407095960 ) ) ;
#29372=CARTESIAN_POINT ( 'NONE',  ( 31.75084456790824206, -10.91497342604502307, -15.84208767625797165 ) ) ;
#29376=CARTESIAN_POINT ( 'NONE',  ( 12.24611073458536836, 9.516504178424655791, -15.33253149294119311 ) ) ;
#29377=CARTESIAN_POINT ( 'NONE',  ( 34.81339731023632567, -19.88166695754494384, -21.17803781427711840 ) ) ;
#29381=CARTESIAN_POINT ( 'NONE',  ( 9.641350810849047548, 17.66889113945805789, -21.33333333332589277 ) ) ;
#29383=CARTESIAN_POINT ( 'NONE',  ( 12.70479305047265761, 7.604386330824797646, -14.96685888413283294 ) ) ;
#29388=CARTESIAN_POINT ( 'NONE',  ( 12.86840956200995301, 9.516103707707461723, -16.11530999810414500 ) ) ;
#29389=CARTESIAN_POINT ( 'NONE',  ( 34.61014508914255572, -12.47609210860084161, -18.96169567217477692 ) ) ;
#29390=CARTESIAN_POINT ( 'NONE',  ( 19.02541433733466647, 1.263421280649871248, -13.57496312174407826 ) ) ;
#29402=CARTESIAN_POINT ( 'NONE',  ( 24.59975295023496855, -6.462932407320696626, -12.83695652901824147 ) ) ;
#29404=CARTESIAN_POINT ( 'NONE',  ( 18.63699955181457923, 5.162464354397502397, -14.86688106074863569 ) ) ;
#29417=CARTESIAN_POINT ( 'NONE',  ( 11.20778676255656059, 9.165115204199564047, -17.24826554773256149 ) ) ;
#29418=CARTESIAN_POINT ( 'NONE',  ( 12.07641845611955489, 8.540206757827041528, -15.45582622123028216 ) ) ;
#29424=CARTESIAN_POINT ( 'NONE',  ( 9.912057827679275235, 16.42739425315605928, -16.50652470164456531 ) ) ;
#29428=CARTESIAN_POINT ( 'NONE',  ( 26.87257363757477435, -3.324124212371978082, -16.68573618535388547 ) ) ;
#29431=CARTESIAN_POINT ( 'NONE',  ( 12.27341590537944249, 9.504120828508773045, -15.31263355901650947 ) ) ;
#29432=CARTESIAN_POINT ( 'NONE',  ( 32.36240160181304759, -11.00785621467150044, -17.57054915585148436 ) ) ;
#29435=CARTESIAN_POINT ( 'NONE',  ( 23.11440248821028831, -7.346120041196752659, -16.32852059634029018 ) ) ;
#29437=CARTESIAN_POINT ( 'NONE',  ( 17.27385296224481337, 7.553222137591894203, -13.16260341916398069 ) ) ;
#29442=CARTESIAN_POINT ( 'NONE',  ( 13.76974871631934860, 5.358497188706473402, -17.46738557873778674 ) ) ;
#29444=CARTESIAN_POINT ( 'NONE',  ( 20.85427418779519826, -0.3072727129311651484, -13.36207100503020584 ) ) ;
#29451=CARTESIAN_POINT ( 'NONE',  ( 28.01381056668970260, -10.10121741814351459, -18.82353034625045041 ) ) ;
#29459=CARTESIAN_POINT ( 'NONE',  ( 27.39421632154990505, -5.413734532252513887, -17.93514013592066902 ) ) ;
#29461=CARTESIAN_POINT ( 'NONE',  ( 34.21167138940940333, -12.68596085309027899, -20.92588972839351058 ) ) ;
#29463=CARTESIAN_POINT ( 'NONE',  ( 12.48799528366842360, 8.565546312597838607, -15.13973160209665991 ) ) ;
#29466=CARTESIAN_POINT ( 'NONE',  ( 13.39606018151479461, 8.691252192278360766, -15.69476314099692971 ) ) ;
#29470=CARTESIAN_POINT ( 'NONE',  ( 9.949118446627077006, 16.25742953053141804, -16.49103975576934644 ) ) ;
#29474=DIRECTION ( 'NONE',  ( 0.000000000000000000, 0.000000000000000000, -1.000000000000000000 ) ) ;
#29478=CARTESIAN_POINT ( 'NONE',  ( 8.944667066222118379, 16.95121494262130213, -17.88907156968992496 ) ) ;
#29479=CARTESIAN_POINT ( 'NONE',  ( 36.54859390953724585, -23.18451583373416014, -17.99055332684694974 ) ) ;
#29480=CARTESIAN_POINT ( 'NONE',  ( 17.34455430865552472, 11.59597468841007384, -15.61519298676701695 ) ) ;
#29482=CARTESIAN_POINT ( 'NONE',  ( 28.40444427461093113, -11.06999723682266179, -18.98653349803348078 ) ) ;
#29495=CARTESIAN_POINT ( 'NONE',  ( 12.40302661446015264, 8.678734247659738443, -16.45371344743900366 ) ) ;
#29496=CARTESIAN_POINT ( 'NONE',  ( 35.54859477393411993, -21.18451971701249548, -18.28760485896911803 ) ) ;
#29497=CARTESIAN_POINT ( 'NONE',  ( 9.026809008904539411, 16.57450152281700184, -17.18797639273109112 ) ) ;
#29500=CARTESIAN_POINT ( 'NONE',  ( 12.86884521499632150, 9.516296226583106588, -16.11496277528728527 ) ) ;
#29506=CARTESIAN_POINT ( 'NONE',  ( 11.65548303173490652, 8.849831895876286936, -15.75351705932409985 ) ) ;
#29510=CARTESIAN_POINT ( 'NONE',  ( 9.661883245193708447, 16.25482579169019459, -17.91553454599451101 ) ) ;
#29511=CARTESIAN_POINT ( 'NONE',  ( 19.63206833423595299, 9.033623817254925470, -16.13982763006638166 ) ) ;
#29512=CARTESIAN_POINT ( 'NONE',  ( 15.79264427988833219, 7.655968387373099482, -13.90199225654327897 ) ) ;
#29519=CARTESIAN_POINT ( 'NONE',  ( 21.19279910686179846, 4.720633506281588510, -19.26595127233560234 ) ) ;
#29525=CARTESIAN_POINT ( 'NONE',  ( 34.54007435814109783, -17.65377171698271752, -20.05309729467257540 ) ) ;
#29531=CARTESIAN_POINT ( 'NONE',  ( 12.24591402697972775, 9.516428332920080280, -15.33268742708093235 ) ) ;
#29532=CARTESIAN_POINT ( 'NONE',  ( 35.54859390953724585, -23.18451583373416014, -18.06010107863414405 ) ) ;
#29536=CARTESIAN_POINT ( 'NONE',  ( 10.66768918063838179, 9.049215891674000645, -16.41161178408055932 ) ) ;
#29542=CARTESIAN_POINT ( 'NONE',  ( 12.86662121207793241, 9.515397394723519753, -16.11672893869402756 ) ) ;
#29544=CARTESIAN_POINT ( 'NONE',  ( 34.52681913409613657, -13.10175273156466069, -19.97882978310374469 ) ) ;
#29545=CARTESIAN_POINT ( 'NONE',  ( 21.43917814492346707, -4.799604530101110988, -17.97822123721208243 ) ) ;
#29553=CARTESIAN_POINT ( 'NONE',  ( 28.56881743257453721, -8.627791766613455593, -12.78522491232925873 ) ) ;
#29554=CARTESIAN_POINT ( 'NONE',  ( 20.87485249991972580, -5.094386175754089585, -18.86169636093909219 ) ) ;
#29564=CARTESIAN_POINT ( 'NONE',  ( 10.89980385979276356, 10.57756405496316710, -17.37562731196375410 ) ) ;
#29565=CARTESIAN_POINT ( 'NONE',  ( 12.23783994716398560, 8.515526397163364791, -15.33449341356891615 ) ) ;
#29572=CARTESIAN_POINT ( 'NONE',  ( 9.641351338355821810, 17.66888872024471624, -17.91303689663363130 ) ) ;
#29579=CARTESIAN_POINT ( 'NONE',  ( 26.80628776457338347, -3.176708023846821494, -16.02594779711905559 ) ) ;
#29582=CARTESIAN_POINT ( 'NONE',  ( 12.24683531348137144, 9.516853939945930208, -15.33195173648645593 ) ) ;
#29585=CARTESIAN_POINT ( 'NONE',  ( 22.90372073960079646, -4.505259139820817715, -13.75793632099288111 ) ) ;
#29587=CARTESIAN_POINT ( 'NONE',  ( 23.04877348721027630, -0.9239720737610787049, -14.85003467231304342 ) ) ;
#29593=CARTESIAN_POINT ( 'NONE',  ( 17.25677449038176547, 8.733363079223632752, -20.54546673180767158 ) ) ;
#29594=CARTESIAN_POINT ( 'NONE',  ( 30.09709056228524204, -9.598102759715754217, -17.07777997130633807 ) ) ;
#29599=CARTESIAN_POINT ( 'NONE',  ( 28.67486520862709654, -7.888541471525570614, -13.83454100519475105 ) ) ;
#29608=CARTESIAN_POINT ( 'NONE',  ( 9.641350810849047548, 17.66889113945805789, -17.98596209335946128 ) ) ;
#29609=CARTESIAN_POINT ( 'NONE',  ( 27.64917536653120678, -4.837437286474155052, -16.54522848743341967 ) ) ;
#29610=CARTESIAN_POINT ( 'NONE',  ( 17.70500667399921824, 3.403337836861581867, -14.36321643528369663 ) ) ;
#29611=CARTESIAN_POINT ( 'NONE',  ( 35.47777500975636400, -18.37389374556380517, -21.30860247919107664 ) ) ;
#29613=CARTESIAN_POINT ( 'NONE',  ( 11.47276097331165623, 9.269810413962238371, -15.86095999428340697 ) ) ;
#29619=CARTESIAN_POINT ( 'NONE',  ( 13.12595734265553205, 8.571888915454989544, -15.91003987120930319 ) ) ;
#29622=CARTESIAN_POINT ( 'NONE',  ( 10.33811693838771717, 18.38618951776012267, -17.92454625180715411 ) ) ;
#29630=CARTESIAN_POINT ( 'NONE',  ( 8.944605280299260386, 16.95149830073946617, -17.90242062344065843 ) ) ;
#29631=CARTESIAN_POINT ( 'NONE',  ( 36.54742519285235858, -23.17926540875556896, -18.54852884019370762 ) ) ;
#29632=CARTESIAN_POINT ( 'NONE',  ( 17.05458169553830317, 2.837819561348359887, -13.69156784695313611 ) ) ;
#29633=CARTESIAN_POINT ( 'NONE',  ( 30.50670359208957905, -8.903545733563623443, -17.67935522427464079 ) ) ;
#29636=CARTESIAN_POINT ( 'NONE',  ( 27.48568275346891809, -3.109927088581168952, -18.71928346135984711 ) ) ;
#29645=CARTESIAN_POINT ( 'NONE',  ( 35.32370156268159178, -20.17419364810216109, -19.24765216636316723 ) ) ;
#29647=CARTESIAN_POINT ( 'NONE',  ( 10.83941243988239833, 8.530520621650927282, -16.32009337531726345 ) ) ;
#29650=EDGE_CURVE ( 'NONE', #24264, #22459, #29254, .T. ) ;
#29651=CARTESIAN_POINT ( 'NONE',  ( 28.75197783424699693, -9.407057218516385433, -18.70835418409691542 ) ) ;
#29653=CARTESIAN_POINT ( 'NONE',  ( 10.35864918915110877, 16.97212501191939538, -17.91752729848689185 ) ) ;
#29659=CARTESIAN_POINT ( 'NONE',  ( 12.50396148805030627, 8.572452836447732594, -15.12701763676990119 ) ) ;
#29662=ORIENTED_EDGE ( 'NONE', *, *, #29650, .F. ) ;
#29663=CARTESIAN_POINT ( 'NONE',  ( 9.661883062008595147, 16.25482663180050835, -17.91564816060341769 ) ) ;
#29665=CARTESIAN_POINT ( 'NONE',  ( 22.00422591904570879, -4.533096263764313072, -16.84388275221259690 ) ) ;
#29666=CARTESIAN_POINT ( 'NONE',  ( 19.13824544459052035, 4.841912194177635520, -12.94453987625427160 ) ) ;
#29671=CARTESIAN_POINT ( 'NONE',  ( 20.24985932600369409, 3.694099309552050237, -20.13309853732883781 ) ) ;
#29678=CARTESIAN_POINT ( 'NONE',  ( 33.38708106686501509, -12.47399286361455850, -19.70456970583452616 ) ) ;
#29684=CARTESIAN_POINT ( 'NONE',  ( 17.78594395145776019, 10.14170102421038422, -17.68001733040774681 ) ) ;
#29685=CARTESIAN_POINT ( 'NONE',  ( 12.24853674868645292, 9.517605834602926862, -15.33059566259575668 ) ) ;
#29686=CARTESIAN_POINT ( 'NONE',  ( 35.54859215833182873, -22.18450796649496226, -18.40462262104107083 ) ) ;
#29690=CARTESIAN_POINT ( 'NONE',  ( 9.641350810849047548, 17.66889113945805789, -17.97192418671891190 ) ) ;
#29691=CARTESIAN_POINT ( 'NONE',  ( 12.78320632028979809, 7.637826363492710158, -14.90445457646871574 ) ) ;
#29697=CARTESIAN_POINT ( 'NONE',  ( 10.35864918915110877, 16.97212501191939538, -23.00000000000000711 ) ) ;
#29698=CARTESIAN_POINT ( 'NONE',  ( 36.54859497913844990, -21.18452063888661385, -18.28382709584098720 ) ) ;
#29699=CARTESIAN_POINT ( 'NONE',  ( 21.10023079691774228, -0.4353598523292347422, -20.14113737667230097 ) ) ;
#29706=CARTESIAN_POINT ( 'NONE',  ( 25.66600519952783799, -8.909200411882650883, -19.30012332941604924 ) ) ;
#29708=CARTESIAN_POINT ( 'NONE',  ( 21.64995824428719828, -4.359751022247916552, -19.89060884261010287 ) ) ;
#29719=UNCERTAINTY_MEASURE_WITH_UNIT (LENGTH_MEASURE( 1.000000000000000082E-05 ), #12587, 'distance_accuracy_value', 'NONE');
#29720=CARTESIAN_POINT ( 'NONE',  ( 11.22336320048417591, 9.093679674329528950, -17.24182414271593800 ) ) ;
#29721=CARTESIAN_POINT ( 'NONE',  ( 10.33811693838771717, 18.38618951776012267, -17.95086732675816776 ) ) ;
#29728=CARTESIAN_POINT ( 'NONE',  ( 9.776119957569173735, 17.05082265352876547, -16.72288386497739765 ) ) ;
#29730=CARTESIAN_POINT ( 'NONE',  ( 15.83821057800014920, 6.120979864746498578, -15.70533851924537672 ) ) ;
#29733=CARTESIAN_POINT ( 'NONE',  ( 21.18945582756405344, -5.194394521544061227, -16.21196392551894405 ) ) ;
#29738=CARTESIAN_POINT ( 'NONE',  ( 11.05541531668977662, 17.68942339022145305, -17.91664992932185996 ) ) ;
#29740=CARTESIAN_POINT ( 'NONE',  ( 35.54287943964028784, -22.15884374752674546, -18.65915260879160797 ) ) ;
#29742=CARTESIAN_POINT ( 'NONE',  ( 23.56138260001205964, -6.829566487537672259, -18.05074380722902916 ) ) ;
#29744=CARTESIAN_POINT ( 'NONE',  ( 21.68595642006795288, -3.720678421232956445, -15.48850127590278980 ) ) ;
#29748=CARTESIAN_POINT ( 'NONE',  ( 14.50439321891314925, 5.533609182599570353, -15.17065254761420512 ) ) ;
#29749=CARTESIAN_POINT ( 'NONE',  ( 29.53935142057454755, -5.962610374456907003, -16.12847026952743690 ) ) ;
#29762=CARTESIAN_POINT ( 'NONE',  ( 26.11288949521356528, -6.777652795969290267, -18.96966820991230662 ) ) ;
#29763=CARTESIAN_POINT ( 'NONE',  ( 14.30110556002302680, 5.443193088601498530, -15.49285935407157666 ) ) ;
#29764=CARTESIAN_POINT ( 'NONE',  ( 35.74526169011073762, -19.57556970876266433, -21.38945728569726867 ) ) ;
#29766=CARTESIAN_POINT ( 'NONE',  ( 12.49957999542663600, 8.570517509188613658, -15.13050969259218981 ) ) ;
#29769=CARTESIAN_POINT ( 'NONE',  ( 9.684081875198721434, 16.15302004482010645, -17.87837111813898616 ) ) ;
#29773=CARTESIAN_POINT ( 'NONE',  ( 12.49899259368311988, 8.570259324921714494, -15.13097775544467005 ) ) ;
#29781=CARTESIAN_POINT ( 'NONE',  ( 13.38776246403941350, 7.629555522264023892, -15.70137656829213491 ) ) ;
#29782=CARTESIAN_POINT ( 'NONE',  ( 35.79875902618127270, -19.81590490140210647, -21.40562824699871314 ) ) ;
#29783=CARTESIAN_POINT ( 'NONE',  ( 21.20591713499851849, 2.664298913801621538, -19.97344039048299891 ) ) ;
#29784=CARTESIAN_POINT ( 'NONE',  ( 30.50415327504139285, -11.36213899161910135, -13.19862950667920565 ) ) ;
#29787=CARTESIAN_POINT ( 'NONE',  ( 21.21264933382939333, -0.1440395243212932441, -13.28659446924270959 ) ) ;
#29796=CARTESIAN_POINT ( 'NONE',  ( 31.84774147790582433, -10.54213090804960018, -15.00000000011102763 ) ) ;
#29803=CARTESIAN_POINT ( 'NONE',  ( 33.33106278064285277, -11.02967194543584029, -16.07471553095689742 ) ) ;
#29805=CARTESIAN_POINT ( 'NONE',  ( 10.66844579733420062, 9.045745945026473223, -16.41129889692150812 ) ) ;
#29807=CARTESIAN_POINT ( 'NONE',  ( 31.81434894052502571, -10.04473835610349575, -15.03854332269495764 ) ) ;
#29809=CARTESIAN_POINT ( 'NONE',  ( 10.35864918915110877, 16.97212501191939538, -17.92279151347709032 ) ) ;
#29820=CARTESIAN_POINT ( 'NONE',  ( 13.12808413666193275, 8.572828783776230921, -15.90834477884588516 ) ) ;
#29822=CARTESIAN_POINT ( 'NONE',  ( 22.09051738352356153, 1.573095004317974333, -13.27920415769822426 ) ) ;
#29823=CARTESIAN_POINT ( 'NONE',  ( 22.68697051328012293, -3.855329871767240402, -18.23939831819710733 ) ) ;
#29825=CARTESIAN_POINT ( 'NONE',  ( 17.94193213664724951, 0.5400182743772068417, -16.55803501089447849 ) ) ;
#29828=CARTESIAN_POINT ( 'NONE',  ( 18.98200677837107264, -2.562081333921657933, -16.63161468174866187 ) ) ;
#29838=CARTESIAN_POINT ( 'NONE',  ( 10.35864940629342890, 16.97212401607702148, -17.91464645457531191 ) ) ;
#29843=CARTESIAN_POINT ( 'NONE',  ( 18.76632379254337835, 6.868107169226369102, -19.55161205380106892 ) ) ;
#29844=CARTESIAN_POINT ( 'NONE',  ( 12.25193961909737794, 9.519109623917222152, -15.32788351481347355 ) ) ;
#29845=CARTESIAN_POINT ( 'NONE',  ( 35.54859390953724585, -22.18451583373416014, -17.64281456791166036 ) ) ;
#29848=CARTESIAN_POINT ( 'NONE',  ( 9.641350810849047548, 17.66889113945805789, -17.91752729848689185 ) ) ;
#29854=CARTESIAN_POINT ( 'NONE',  ( 10.35864918915110877, 16.97212501191939538, -17.95086732675817132 ) ) ;
#29855=CARTESIAN_POINT ( 'NONE',  ( 36.54859390953724585, -21.18451583373416014, -17.78191007148576119 ) ) ;
#29857=CARTESIAN_POINT ( 'NONE',  ( 22.97938783112199701, -3.359759438970757017, -19.62490732200095067 ) ) ;
#29862=CARTESIAN_POINT ( 'NONE',  ( 23.72517123929712213, -5.798560033841243744, -19.46542475990168342 ) ) ;
#29863=CARTESIAN_POINT ( 'NONE',  ( 27.35978538551520245, -3.059420540688277956, -14.62525642202852971 ) ) ;
#29874=CARTESIAN_POINT ( 'NONE',  ( 12.50736435846123484, 8.573956625762026107, -15.12430548898761806 ) ) ;
#29879=CARTESIAN_POINT ( 'NONE',  ( 9.870716668364401869, 16.61699007954640805, -16.53972800451630931 ) ) ;
#29880=CARTESIAN_POINT ( 'NONE',  ( 17.26923406770577074, 6.766716122889627094, -15.27140832040383422 ) ) ;
#29883=CARTESIAN_POINT ( 'NONE',  ( 23.21730923944814506, -4.364887171357101359, -13.63095412955673247 ) ) ;
#29887=CARTESIAN_POINT ( 'NONE',  ( 11.05541529015696156, 17.68942351190433726, -17.91624098666951070 ) ) ;
#29889=CARTESIAN_POINT ( 'NONE',  ( 32.01580575020638975, -11.60503005433848500, -14.58926670671732673 ) ) ;
#29891=CARTESIAN_POINT ( 'NONE',  ( 26.80628776457338347, -3.176708023846821494, -16.02594779711905559 ) ) ;
#29893=CARTESIAN_POINT ( 'NONE',  ( 21.61496389699315657, -3.514534563429178249, -17.40323974765788506 ) ) ;
#29897=CARTESIAN_POINT ( 'NONE',  ( 18.47844294452917424, 10.16049799425131361, -18.92511192449534718 ) ) ;
#29898=CARTESIAN_POINT ( 'NONE',  ( 28.24905293252005123, -11.45655955306129314, -17.88756844200554141 ) ) ;
#29910=CARTESIAN_POINT ( 'NONE',  ( 25.51539342332723947, -8.447981945391376257, -12.99903862581394876 ) ) ;
#29911=CARTESIAN_POINT ( 'NONE',  ( 20.41927524488895429, 4.553956414902842198, -14.69105443414393264 ) ) ;
#29912=CARTESIAN_POINT ( 'NONE',  ( 35.81175537756147520, -19.87429062379433731, -21.40957262365663993 ) ) ;
#29914=CARTESIAN_POINT ( 'NONE',  ( 12.49860086554322436, 8.570087612320898884, -15.13128986298120537 ) ) ;
#29917=CARTESIAN_POINT ( 'NONE',  ( 9.668505437271095460, 16.22445557469016464, -17.88481252315560965 ) ) ;
#29922=CARTESIAN_POINT ( 'NONE',  ( 10.33811693838771717, 18.38618951776012267, -17.98596209335946128 ) ) ;
#29929=CARTESIAN_POINT ( 'NONE',  ( 14.93287775521291394, 9.378568215907955974, -14.88591063491414168 ) ) ;
#29931=CARTESIAN_POINT ( 'NONE',  ( 9.242255153701981030, 15.58643803978083753, -17.00107889682120899 ) ) ;
#29932=CARTESIAN_POINT ( 'NONE',  ( 34.70640263809442416, -19.40099657226499019, -21.14569589167440000 ) ) ;
#29933=CARTESIAN_POINT ( 'NONE',  ( 22.65699622776610411, 4.567421951779635947, -17.29570926971318556 ) ) ;
#29934=CARTESIAN_POINT ( 'NONE',  ( 18.96102019896426683, 9.324696518442671334, -18.66317648627137515 ) ) ;
#29937=CARTESIAN_POINT ( 'NONE',  ( 27.86916612644401425, -2.348388412649441648, -16.97020329177912501 ) ) ;
#29944=CARTESIAN_POINT ( 'NONE',  ( 33.94960473074984009, -11.12362044852780407, -17.82291586202971700 ) ) ;
#29945=CARTESIAN_POINT ( 'NONE',  ( 10.65857126575392400, 9.091031811597934720, -16.41538236262689310 ) ) ;
#29948=CARTESIAN_POINT ( 'NONE',  ( 26.92971693216691165, -8.617903733377630715, -13.36642543767191427 ) ) ;
#29950=CARTESIAN_POINT ( 'NONE',  ( 11.12037835888041393, 13.47873794165536410, -17.06668569338069830 ) ) ;
#29964=CARTESIAN_POINT ( 'NONE',  ( 9.661883061612440926, 16.25482663361732705, -17.92015940598198753 ) ) ;
#29965=CARTESIAN_POINT ( 'NONE',  ( 20.01442678821067034, -2.980627454636011198, -16.03144472681325183 ) ) ;
#29966=CARTESIAN_POINT ( 'NONE',  ( 20.35037346166061312, -2.402462631129500092, -18.68063351227773694 ) ) ;
#29967=CARTESIAN_POINT ( 'NONE',  ( 16.95656709563420250, 3.789241241613106048, -19.64973185778705655 ) ) ;
#29970=CARTESIAN_POINT ( 'NONE',  ( 18.97268594440662426, -2.511067197207834667, -17.06021009607598415 ) ) ;
#29976=CARTESIAN_POINT ( 'NONE',  ( 10.36219267574928260, 16.95587413069128857, -17.77286471925143019 ) ) ;
#29977=CARTESIAN_POINT ( 'NONE',  ( 35.54502023521215648, -22.16846120802060938, -18.59538644662325524 ) ) ;
#29982=CARTESIAN_POINT ( 'NONE',  ( 17.32695330507268494, 5.471673316493076200, -20.08600194542987794 ) ) ;
#29983=CARTESIAN_POINT ( 'NONE',  ( 11.79482239888288042, 14.29840825880376265, -16.57005305382644877 ) ) ;
#29984=CARTESIAN_POINT ( 'NONE',  ( 35.54859390953723874, -22.18451583373416014, -15.00000000000000000 ) ) ;
#29987=CARTESIAN_POINT ( 'NONE',  ( 9.914377700407460026, 16.41675502110963336, -16.50544604630902867 ) ) ;
#29990=CARTESIAN_POINT ( 'NONE',  ( 9.641350829061996919, 17.66889105593114806, -17.91548090047172437 ) ) ;
#29999=CARTESIAN_POINT ( 'NONE',  ( 12.86835069890237548, 9.516077773083457814, -16.11535690708815594 ) ) ;
#30000=CARTESIAN_POINT ( 'NONE',  ( 35.88208498122789791, -19.19024427843809733, -20.38849413606966010 ) ) ;
#30001=CARTESIAN_POINT ( 'NONE',  ( 25.04992766293576878, -3.547109489677171101, -13.67097983722207033 ) ) ;
#30004=CARTESIAN_POINT ( 'NONE',  ( 26.83671086236671144, -5.482767762337403816, -13.01846673106422436 ) ) ;
#30005=CARTESIAN_POINT ( 'NONE',  ( 20.82548126942529976, -5.669333895406754031, -14.77195412306030420 ) ) ;
#30013=CARTESIAN_POINT ( 'NONE',  ( 10.33811693838771717, 18.38618951776012267, -21.33333333332589632 ) ) ;
#30021=CARTESIAN_POINT ( 'NONE',  ( 18.26355027798676645, 7.143056880744947712, -15.77244846760033958 ) ) ;
#30025=CARTESIAN_POINT ( 'NONE',  ( 21.57856661146780652, -4.666631351218505586, -18.28211233923166645 ) ) ;
#30030=CARTESIAN_POINT ( 'NONE',  ( 12.24532799939971284, 9.516186676127107447, -15.33315318048745013 ) ) ;
#30032=CARTESIAN_POINT ( 'NONE',  ( 34.54007435814109783, -17.65377171698271752, -20.05309729467257540 ) ) ;
#30033=CARTESIAN_POINT ( 'NONE',  ( 15.22033579473957410, 7.355362781181614018, -19.64495939069069763 ) ) ;
#30037=CARTESIAN_POINT ( 'NONE',  ( 20.30498772102510685, -2.023023832184298154, -16.94527736422809028 ) ) ;
#30040=( NAMED_UNIT ( * ) SI_UNIT ( $, .STERADIAN. ) SOLID_ANGLE_UNIT ( ) );
#30041=CARTESIAN_POINT ( 'NONE',  ( 17.46151185945609186, 6.859213057953727599, -13.86392132274949418 ) ) ;
#30042=CARTESIAN_POINT ( 'NONE',  ( 28.79879967665997142, -10.96283228269853893, -18.01937015232834938 ) ) ;
#30053=CARTESIAN_POINT ( 'NONE',  ( 18.06018518654990856, -2.098401534709970928, -17.02619504079518364 ) ) ;
#30054=CARTESIAN_POINT ( 'NONE',  ( 21.13650371987585075, 4.769999862021419901, -15.38713752973847448 ) ) ;
#30055=CARTESIAN_POINT ( 'NONE',  ( 32.84381624265927968, -11.41053889131397980, -20.36336433681493929 ) ) ;
#30056=CARTESIAN_POINT ( 'NONE',  ( 11.47219014545126647, 9.272428573238919114, -15.86119603109536058 ) ) ;
#30059=CARTESIAN_POINT ( 'NONE',  ( 9.927226272117462003, 15.03792884684924402, -17.77782235690405344 ) ) ;
#30064=CARTESIAN_POINT ( 'NONE',  ( 12.47535353872619446, 8.560407331872438519, -15.14977315560688176 ) ) ;
#30070=CARTESIAN_POINT ( 'NONE',  ( 15.19603151210977821, 9.502094893032342782, -14.87270315361914896 ) ) ;
#30073=CARTESIAN_POINT ( 'NONE',  ( 9.112705230111354027, 16.18057050314154210, -17.05465234812585607 ) ) ;
#30074=CARTESIAN_POINT ( 'NONE',  ( 32.12153525177792091, -10.97127362787143312, -16.88978156643115724 ) ) ;
#30075=CARTESIAN_POINT ( 'NONE',  ( 16.77192278198516107, 3.819237988068143075, -20.73389043596634806 ) ) ;
#30077=CARTESIAN_POINT ( 'NONE',  ( 19.63213555404020383, 6.204410169219986670, -18.27402551702938638 ) ) ;
#30080=CARTESIAN_POINT ( 'NONE',  ( 22.33422182767193576, -8.475443503041637072, -15.36134680393336538 ) ) ;
#30091=CARTESIAN_POINT ( 'NONE',  ( 32.96976325559394638, -10.97479806523316448, -15.05356414682637833 ) ) ;
#30093=CARTESIAN_POINT ( 'NONE',  ( 10.68417091768239047, 8.977850322645869241, -16.40447401652228621 ) ) ;
#30095=CARTESIAN_POINT ( 'NONE',  ( 27.01132674553606350, -11.00696853675122711, -18.49859303458091730 ) ) ;
#30097=CARTESIAN_POINT ( 'NONE',  ( 10.36007019289729847, 16.96560810760319882, -17.82599398985513872 ) ) ;
#30107=CARTESIAN_POINT ( 'NONE',  ( 9.667859086210386366, 16.22741982304516739, -17.88507982571460531 ) ) ;
#30108=CARTESIAN_POINT ( 'NONE',  ( 22.53049847760648561, -4.001888697258268124, -18.07502562731026075 ) ) ;
#30109=CARTESIAN_POINT ( 'NONE',  ( 24.39898194048076974, -1.181968365584514791, -14.84216225329429051 ) ) ;
#30111=CARTESIAN_POINT ( 'NONE',  ( 20.05507840940144959, 2.642024363331392234, -19.51255487852252912 ) ) ;
#30117=CARTESIAN_POINT ( 'NONE',  ( 24.14158683625483803, -3.940216521628096658, -13.50644477367014673 ) ) ;
#30126=CARTESIAN_POINT ( 'NONE',  ( 10.35873811938078504, 16.97171716655003593, -17.89325570535168453 ) ) ;
#30127=CARTESIAN_POINT ( 'NONE',  ( 35.54859569580823830, -22.18452385850428499, -18.27063337037174762 ) ) ;
#30133=CARTESIAN_POINT ( 'NONE',  ( 14.79111372287554715, 6.954724682967856175, -19.27298399620107361 ) ) ;
#30134=CARTESIAN_POINT ( 'NONE',  ( 11.06231504941914423, 17.65778033641372957, -17.63750823492871334 ) ) ;
#30135=CARTESIAN_POINT ( 'NONE',  ( 35.18065281855160720, -20.53155141575438591, -20.22037173032050461 ) ) ;
#30139=CARTESIAN_POINT ( 'NONE',  ( 9.641352920869014298, 17.66888146263751125, -17.91030124961049097 ) ) ;
#30140=CARTESIAN_POINT ( 'NONE',  ( 12.89209817343266984, 7.685947621549766851, -14.81766584744191739 ) ) ;
#30146=CARTESIAN_POINT ( 'NONE',  ( 10.48009811366078381, 16.41514476298091907, -17.33146409796769660 ) ) ;
#30147=CARTESIAN_POINT ( 'NONE',  ( 34.27125395597954594, -11.98684039141630819, -19.88226891060491752 ) ) ;
#30148=CARTESIAN_POINT ( 'NONE',  ( 23.22413189157496305, -7.367447486509826504, -15.63851824576001981 ) ) ;
#30154=CARTESIAN_POINT ( 'NONE',  ( 18.96102019896426683, 9.324696518442671334, -18.66317648627137515 ) ) ;
#30155=CARTESIAN_POINT ( 'NONE',  ( 25.27624414898354388, -7.528478751523516088, -13.47981680254768655 ) ) ;
#30168=CARTESIAN_POINT ( 'NONE',  ( 10.33811811146757265, 18.38618413786636552, -17.91101973220562371 ) ) ;
#30173=CARTESIAN_POINT ( 'NONE',  ( 11.46269231744662420, 9.315986823159681407, -15.86512371708112212 ) ) ;
#30175=CARTESIAN_POINT ( 'NONE',  ( 17.51631511252498186, 5.448942031446791567, -19.07752241466814880 ) ) ;
#30182=CARTESIAN_POINT ( 'NONE',  ( 12.24853674868645292, 9.517605834602926862, -15.33059566259575668 ) ) ;
#30184=CARTESIAN_POINT ( 'NONE',  ( 34.93238815599637803, -19.41622979634004764, -20.17168434421570922 ) ) ;
#30187=CARTESIAN_POINT ( 'NONE',  ( 21.64008331710702038, -0.7226702609205537531, -18.85644019536628946 ) ) ;
#30191=CARTESIAN_POINT ( 'NONE',  ( 22.47820520476076567, 2.340993144345510313, -15.49451772223075707 ) ) ;
#30192=CARTESIAN_POINT ( 'NONE',  ( 27.79808892257030806, -9.771933472778439267, -13.29678235002263165 ) ) ;
#30202=CARTESIAN_POINT ( 'NONE',  ( 9.917712295358372288, 16.40146214360271770, -16.50402730409559027 ) ) ;
#30204=CARTESIAN_POINT ( 'NONE',  ( 21.41414477019618090, -0.8106431452899078849, -12.56463806509592018 ) ) ;
#30205=CARTESIAN_POINT ( 'NONE',  ( 14.50439321891314925, 5.533609182599570353, -15.17065254761420512 ) ) ;
#30206=CARTESIAN_POINT ( 'NONE',  ( 31.83585693452864973, -10.27807049784803972, -18.08404909334234745 ) ) ;
#30211=CARTESIAN_POINT ( 'NONE',  ( 17.85084670134855145, 5.929878015568476712, -20.08862479909851828 ) ) ;
#30214=CARTESIAN_POINT ( 'NONE',  ( 12.93612603019711571, 8.763434079353435990, -14.78257486846209545 ) ) ;
#30218=CARTESIAN_POINT ( 'NONE',  ( 14.24706144987486667, 6.238427219560604087, -16.72753349211556184 ) ) ;
#30220=CARTESIAN_POINT ( 'NONE',  ( 34.52807818452484412, -18.59987926346575549, -21.09179268733712576 ) ) ;
#30224=CARTESIAN_POINT ( 'NONE',  ( 19.88777865313588222, 4.107626486979258473, -13.29018489620430721 ) ) ;
#30225=CARTESIAN_POINT ( 'NONE',  ( 18.83884422780463552, 9.149888288241003309, -18.99120665306858768 ) ) ;
#30228=CARTESIAN_POINT ( 'NONE',  ( 22.29950228926167100, 0.3472756386405770335, -13.33132414558515677 ) ) ;
#30239=CARTESIAN_POINT ( 'NONE',  ( 34.58206770820681442, -12.34995000336197890, -18.95321163875382453 ) ) ;
#30241=CARTESIAN_POINT ( 'NONE',  ( 12.73046782819888989, 7.614823354231524455, -14.94646497050939793 ) ) ;
#30245=CARTESIAN_POINT ( 'NONE',  ( 10.40163623209820365, 16.77498095339038287, -17.46874319472340176 ) ) ;
#30256=CARTESIAN_POINT ( 'NONE',  ( 9.927226272117462003, 15.03792884684924402, -17.77782235690405344 ) ) ;
#30258=CARTESIAN_POINT ( 'NONE',  ( 20.12919692000023986, -2.949910412001375715, -15.69023992059449846 ) ) ;
#30259=CARTESIAN_POINT ( 'NONE',  ( 23.86816030614728135, 2.079196616232401595, -15.13732202275373062 ) ) ;
#30261=CARTESIAN_POINT ( 'NONE',  ( 19.47744964272635926, 1.166342761889149982, -14.46873920536258495 ) ) ;
ENDSEC;
END-ISO-10303-21;
